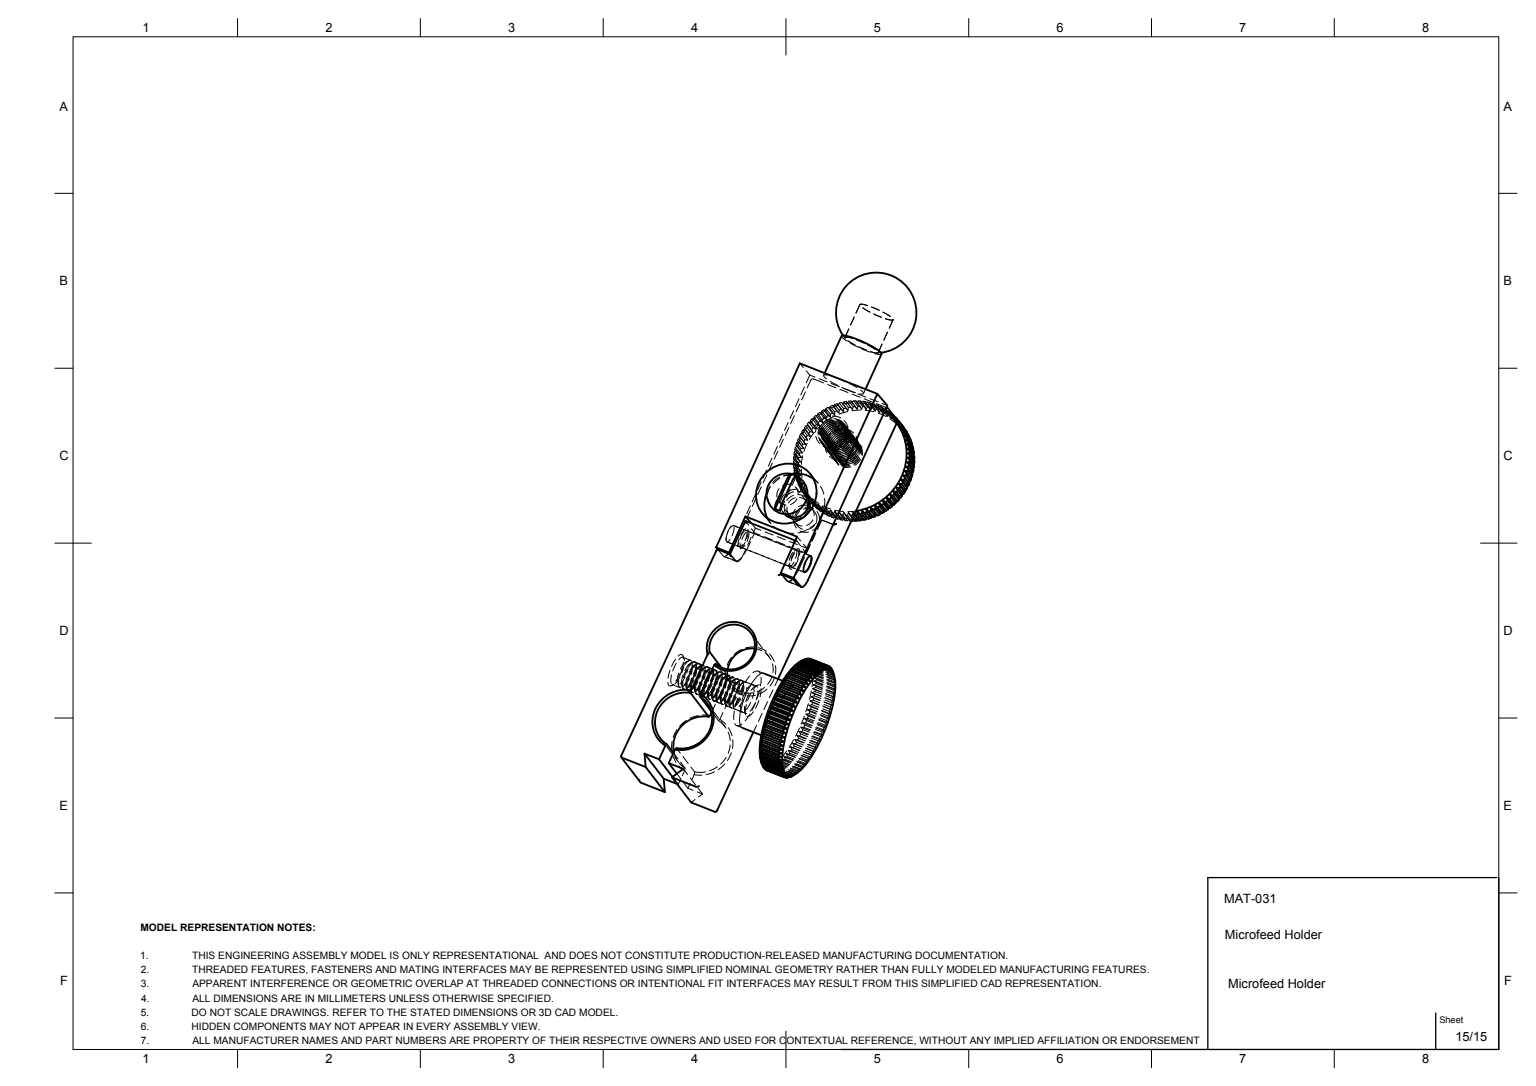
ISO-10303-21;
HEADER;
/* Generated by software containing ST-Developer
 * from STEP Tools, Inc. (www.steptools.com) 
 */

FILE_DESCRIPTION(
/* description */ ('STEP AP214'),
/* implementation_level */ '2;1');

FILE_NAME(
/* name */ 'Microfeed Holder.step',
/* time_stamp */ '2026-11-14T06:58:01-08:00',
/* author */ (''),
/* organization */ (''),
/* preprocessor_version */ 'ST-DEVELOPER v20.2',
/* originating_system */ 'Autodesk Translation Framework v15.17.0.0',
/* authorisation */ '');

FILE_SCHEMA (('AUTOMOTIVE_DESIGN { 1 0 10303 214 3 1 1 }'));
ENDSEC;

DATA;
#10=MECHANICAL_DESIGN_GEOMETRIC_PRESENTATION_REPRESENTATION('',(#1159,#1160,#1161,#1162,#1163,#1164,#1165),#38635);
#68=ELLIPSE('',#18534,0.424264068711536,0.299999999999714);
#69=ELLIPSE('',#18536,0.424264068712725,0.300000000000503);
#70=ELLIPSE('',#18544,0.424264068711314,0.299999999999553);
#71=ELLIPSE('',#18551,0.424264068712409,0.300000000000364);
#72=ELLIPSE('',#18570,0.424264068711872,0.299999999999922);
#73=ELLIPSE('',#18576,0.42426406871188,0.299999999999951);
#74=ELLIPSE('',#18583,0.424264068709732,0.299999999998459);
#75=ELLIPSE('',#18585,0.424264068710271,0.299999999998872);
#76=ELLIPSE('',#18587,0.424264068711053,0.29999999999941);
#77=ELLIPSE('',#18589,0.424264068710426,0.299999999998988);
#117=SPHERICAL_SURFACE('',#18547,0.3);
#118=SPHERICAL_SURFACE('',#18565,0.3);
#119=SPHERICAL_SURFACE('',#18567,0.3);
#120=SPHERICAL_SURFACE('',#18577,0.3);
#121=SPHERICAL_SURFACE('',#18580,0.3);
#122=SPHERICAL_SURFACE('',#18592,0.3);
#123=SPHERICAL_SURFACE('',#18653,5.5);
#179=TOROIDAL_SURFACE('',#18545,3.3,0.3);
#180=TOROIDAL_SURFACE('',#18563,3.3,0.3);
#181=TOROIDAL_SURFACE('',#18597,1.1,0.1);
#182=TOROIDAL_SURFACE('',#18602,1.1,0.1);
#183=TOROIDAL_SURFACE('',#18656,2.5,0.5);
#184=TOROIDAL_SURFACE('',#19189,1.81782234903766,0.9);
#185=TOROIDAL_SURFACE('',#19210,4.5,0.5);
#238=(
BOUNDED_CURVE()
B_SPLINE_CURVE(2,(#33393,#33394,#33395),.UNSPECIFIED.,.F.,.F.)
B_SPLINE_CURVE_WITH_KNOTS((3,3),(0.0421543904155743,0.059561882542862),
 .UNSPECIFIED.)
CURVE()
GEOMETRIC_REPRESENTATION_ITEM()
RATIONAL_B_SPLINE_CURVE((1.21505376344088,1.25768410333319,1.29885057471263))
REPRESENTATION_ITEM('')
);
#239=(
BOUNDED_CURVE()
B_SPLINE_CURVE(2,(#33398,#33399,#33400),.UNSPECIFIED.,.F.,.F.)
B_SPLINE_CURVE_WITH_KNOTS((3,3),(-0.162076637737085,-0.10981765032222),
 .UNSPECIFIED.)
CURVE()
GEOMETRIC_REPRESENTATION_ITEM()
RATIONAL_B_SPLINE_CURVE((1.22222222222222,1.19527460940787,1.16260162601569))
REPRESENTATION_ITEM('')
);
#240=(
BOUNDED_CURVE()
B_SPLINE_CURVE(2,(#33434,#33435,#33436),.UNSPECIFIED.,.F.,.F.)
B_SPLINE_CURVE_WITH_KNOTS((3,3),(0.109817650322217,0.162076637737086),
 .UNSPECIFIED.)
CURVE()
GEOMETRIC_REPRESENTATION_ITEM()
RATIONAL_B_SPLINE_CURVE((1.16260162601569,1.19527460940787,1.22222222222222))
REPRESENTATION_ITEM('')
);
#241=(
BOUNDED_CURVE()
B_SPLINE_CURVE(2,(#33439,#33440,#33441),.UNSPECIFIED.,.F.,.F.)
B_SPLINE_CURVE_WITH_KNOTS((3,3),(-0.0595618825429998,-0.0421543904157002),
 .UNSPECIFIED.)
CURVE()
GEOMETRIC_REPRESENTATION_ITEM()
RATIONAL_B_SPLINE_CURVE((1.29885057471333,1.25768410333386,1.21505376344153))
REPRESENTATION_ITEM('')
);
#242=(
BOUNDED_CURVE()
B_SPLINE_CURVE(2,(#34217,#34218,#34219),.UNSPECIFIED.,.F.,.F.)
B_SPLINE_CURVE_WITH_KNOTS((3,3),(0.536094506482407,0.589144372850599),
 .UNSPECIFIED.)
CURVE()
GEOMETRIC_REPRESENTATION_ITEM()
RATIONAL_B_SPLINE_CURVE((1.0242816296211,1.02311336089471,1.02147610370002))
REPRESENTATION_ITEM('')
);
#243=(
BOUNDED_CURVE()
B_SPLINE_CURVE(2,(#34223,#34224,#34225),.UNSPECIFIED.,.F.,.F.)
B_SPLINE_CURVE_WITH_KNOTS((3,3),(0.218746031477168,0.271795897845357),
 .UNSPECIFIED.)
CURVE()
GEOMETRIC_REPRESENTATION_ITEM()
RATIONAL_B_SPLINE_CURVE((1.02147610369998,1.02311336089466,1.02428162962105))
REPRESENTATION_ITEM('')
);
#244=(
BOUNDED_CURVE()
B_SPLINE_CURVE(2,(#34227,#34228,#34229),.UNSPECIFIED.,.F.,.F.)
B_SPLINE_CURVE_WITH_KNOTS((3,3),(0.536094506482406,0.589144372850588),
 .UNSPECIFIED.)
CURVE()
GEOMETRIC_REPRESENTATION_ITEM()
RATIONAL_B_SPLINE_CURVE((1.02428162962092,1.02311336089453,1.02147610369986))
REPRESENTATION_ITEM('')
);
#245=(
BOUNDED_CURVE()
B_SPLINE_CURVE(2,(#34233,#34234,#34235),.UNSPECIFIED.,.F.,.F.)
B_SPLINE_CURVE_WITH_KNOTS((3,3),(0.21874603147717,0.271795897845354),
 .UNSPECIFIED.)
CURVE()
GEOMETRIC_REPRESENTATION_ITEM()
RATIONAL_B_SPLINE_CURVE((1.02147610369991,1.02311336089458,1.02428162962097))
REPRESENTATION_ITEM('')
);
#246=(
BOUNDED_CURVE()
B_SPLINE_CURVE(2,(#34237,#34238,#34239),.UNSPECIFIED.,.F.,.F.)
B_SPLINE_CURVE_WITH_KNOTS((3,3),(0.536094506482412,0.589144372850605),
 .UNSPECIFIED.)
CURVE()
GEOMETRIC_REPRESENTATION_ITEM()
RATIONAL_B_SPLINE_CURVE((1.02428162962116,1.02311336089476,1.02147610370007))
REPRESENTATION_ITEM('')
);
#247=(
BOUNDED_CURVE()
B_SPLINE_CURVE(2,(#34243,#34244,#34245),.UNSPECIFIED.,.F.,.F.)
B_SPLINE_CURVE_WITH_KNOTS((3,3),(0.218746031477164,0.27179589784535),
 .UNSPECIFIED.)
CURVE()
GEOMETRIC_REPRESENTATION_ITEM()
RATIONAL_B_SPLINE_CURVE((1.02147610369995,1.02311336089462,1.02428162962101))
REPRESENTATION_ITEM('')
);
#248=(
BOUNDED_CURVE()
B_SPLINE_CURVE(2,(#34247,#34248,#34249),.UNSPECIFIED.,.F.,.F.)
B_SPLINE_CURVE_WITH_KNOTS((3,3),(0.536094506482389,0.589144372850566),
 .UNSPECIFIED.)
CURVE()
GEOMETRIC_REPRESENTATION_ITEM()
RATIONAL_B_SPLINE_CURVE((1.0242816296208,1.02311336089442,1.02147610369976))
REPRESENTATION_ITEM('')
);
#249=(
BOUNDED_CURVE()
B_SPLINE_CURVE(2,(#34253,#34254,#34255),.UNSPECIFIED.,.F.,.F.)
B_SPLINE_CURVE_WITH_KNOTS((3,3),(0.218746031477182,0.271795897845361),
 .UNSPECIFIED.)
CURVE()
GEOMETRIC_REPRESENTATION_ITEM()
RATIONAL_B_SPLINE_CURVE((1.02147610369979,1.02311336089445,1.02428162962083))
REPRESENTATION_ITEM('')
);
#250=(
BOUNDED_CURVE()
B_SPLINE_CURVE(2,(#34257,#34258,#34259),.UNSPECIFIED.,.F.,.F.)
B_SPLINE_CURVE_WITH_KNOTS((3,3),(0.536094506482412,0.589144372850601),
 .UNSPECIFIED.)
CURVE()
GEOMETRIC_REPRESENTATION_ITEM()
RATIONAL_B_SPLINE_CURVE((1.02428162962106,1.02311336089466,1.02147610369999))
REPRESENTATION_ITEM('')
);
#251=(
BOUNDED_CURVE()
B_SPLINE_CURVE(2,(#34263,#34264,#34265),.UNSPECIFIED.,.F.,.F.)
B_SPLINE_CURVE_WITH_KNOTS((3,3),(0.218746031477185,0.271795897845363),
 .UNSPECIFIED.)
CURVE()
GEOMETRIC_REPRESENTATION_ITEM()
RATIONAL_B_SPLINE_CURVE((1.02147610369979,1.02311336089445,1.02428162962084))
REPRESENTATION_ITEM('')
);
#252=(
BOUNDED_CURVE()
B_SPLINE_CURVE(2,(#34267,#34268,#34269),.UNSPECIFIED.,.F.,.F.)
B_SPLINE_CURVE_WITH_KNOTS((3,3),(0.536094506482394,0.589144372850572),
 .UNSPECIFIED.)
CURVE()
GEOMETRIC_REPRESENTATION_ITEM()
RATIONAL_B_SPLINE_CURVE((1.02428162962082,1.02311336089444,1.02147610369978))
REPRESENTATION_ITEM('')
);
#253=(
BOUNDED_CURVE()
B_SPLINE_CURVE(2,(#34273,#34274,#34275),.UNSPECIFIED.,.F.,.F.)
B_SPLINE_CURVE_WITH_KNOTS((3,3),(0.21874603147717,0.271795897845349),
 .UNSPECIFIED.)
CURVE()
GEOMETRIC_REPRESENTATION_ITEM()
RATIONAL_B_SPLINE_CURVE((1.02147610369983,1.0231133608945,1.02428162962088))
REPRESENTATION_ITEM('')
);
#254=(
BOUNDED_CURVE()
B_SPLINE_CURVE(2,(#34277,#34278,#34279),.UNSPECIFIED.,.F.,.F.)
B_SPLINE_CURVE_WITH_KNOTS((3,3),(0.536094506482412,0.589144372850599),
 .UNSPECIFIED.)
CURVE()
GEOMETRIC_REPRESENTATION_ITEM()
RATIONAL_B_SPLINE_CURVE((1.02428162962104,1.02311336089465,1.02147610369997))
REPRESENTATION_ITEM('')
);
#255=(
BOUNDED_CURVE()
B_SPLINE_CURVE(2,(#34283,#34284,#34285),.UNSPECIFIED.,.F.,.F.)
B_SPLINE_CURVE_WITH_KNOTS((3,3),(0.218746031477174,0.271795897845355),
 .UNSPECIFIED.)
CURVE()
GEOMETRIC_REPRESENTATION_ITEM()
RATIONAL_B_SPLINE_CURVE((1.02147610369982,1.02311336089449,1.02428162962087))
REPRESENTATION_ITEM('')
);
#256=(
BOUNDED_CURVE()
B_SPLINE_CURVE(2,(#34287,#34288,#34289),.UNSPECIFIED.,.F.,.F.)
B_SPLINE_CURVE_WITH_KNOTS((3,3),(0.536094506482407,0.589144372850592),
 .UNSPECIFIED.)
CURVE()
GEOMETRIC_REPRESENTATION_ITEM()
RATIONAL_B_SPLINE_CURVE((1.02428162962099,1.0231133608946,1.02147610369992))
REPRESENTATION_ITEM('')
);
#257=(
BOUNDED_CURVE()
B_SPLINE_CURVE(2,(#34293,#34294,#34295),.UNSPECIFIED.,.F.,.F.)
B_SPLINE_CURVE_WITH_KNOTS((3,3),(0.218746031477156,0.271795897845345),
 .UNSPECIFIED.)
CURVE()
GEOMETRIC_REPRESENTATION_ITEM()
RATIONAL_B_SPLINE_CURVE((1.02147610369998,1.02311336089466,1.02428162962106))
REPRESENTATION_ITEM('')
);
#258=(
BOUNDED_CURVE()
B_SPLINE_CURVE(2,(#34297,#34298,#34299),.UNSPECIFIED.,.F.,.F.)
B_SPLINE_CURVE_WITH_KNOTS((3,3),(0.53609450648241,0.5891443728506),
 .UNSPECIFIED.)
CURVE()
GEOMETRIC_REPRESENTATION_ITEM()
RATIONAL_B_SPLINE_CURVE((1.02428162962108,1.02311336089468,1.0214761037))
REPRESENTATION_ITEM('')
);
#259=(
BOUNDED_CURVE()
B_SPLINE_CURVE(2,(#34303,#34304,#34305),.UNSPECIFIED.,.F.,.F.)
B_SPLINE_CURVE_WITH_KNOTS((3,3),(0.21874603147718,0.271795897845362),
 .UNSPECIFIED.)
CURVE()
GEOMETRIC_REPRESENTATION_ITEM()
RATIONAL_B_SPLINE_CURVE((1.02147610369984,1.02311336089451,1.02428162962089))
REPRESENTATION_ITEM('')
);
#260=(
BOUNDED_CURVE()
B_SPLINE_CURVE(2,(#34307,#34308,#34309),.UNSPECIFIED.,.F.,.F.)
B_SPLINE_CURVE_WITH_KNOTS((3,3),(0.536094506482414,0.589144372850597),
 .UNSPECIFIED.)
CURVE()
GEOMETRIC_REPRESENTATION_ITEM()
RATIONAL_B_SPLINE_CURVE((1.02428162962095,1.02311336089456,1.02147610369989))
REPRESENTATION_ITEM('')
);
#261=(
BOUNDED_CURVE()
B_SPLINE_CURVE(2,(#34313,#34314,#34315),.UNSPECIFIED.,.F.,.F.)
B_SPLINE_CURVE_WITH_KNOTS((3,3),(0.218746031477174,0.27179589784536),
 .UNSPECIFIED.)
CURVE()
GEOMETRIC_REPRESENTATION_ITEM()
RATIONAL_B_SPLINE_CURVE((1.02147610369991,1.02311336089459,1.02428162962097))
REPRESENTATION_ITEM('')
);
#262=(
BOUNDED_CURVE()
B_SPLINE_CURVE(2,(#34317,#34318,#34319),.UNSPECIFIED.,.F.,.F.)
B_SPLINE_CURVE_WITH_KNOTS((3,3),(0.536094506482426,0.589144372850614),
 .UNSPECIFIED.)
CURVE()
GEOMETRIC_REPRESENTATION_ITEM()
RATIONAL_B_SPLINE_CURVE((1.02428162962107,1.02311336089468,1.0214761037))
REPRESENTATION_ITEM('')
);
#263=(
BOUNDED_CURVE()
B_SPLINE_CURVE(2,(#34323,#34324,#34325),.UNSPECIFIED.,.F.,.F.)
B_SPLINE_CURVE_WITH_KNOTS((3,3),(0.218746031477169,0.271795897845354),
 .UNSPECIFIED.)
CURVE()
GEOMETRIC_REPRESENTATION_ITEM()
RATIONAL_B_SPLINE_CURVE((1.02147610369993,1.0231133608946,1.02428162962099))
REPRESENTATION_ITEM('')
);
#264=(
BOUNDED_CURVE()
B_SPLINE_CURVE(2,(#34327,#34328,#34329),.UNSPECIFIED.,.F.,.F.)
B_SPLINE_CURVE_WITH_KNOTS((3,3),(0.536094506482401,0.589144372850587),
 .UNSPECIFIED.)
CURVE()
GEOMETRIC_REPRESENTATION_ITEM()
RATIONAL_B_SPLINE_CURVE((1.02428162962099,1.0231133608946,1.02147610369993))
REPRESENTATION_ITEM('')
);
#265=(
BOUNDED_CURVE()
B_SPLINE_CURVE(2,(#34333,#34334,#34335),.UNSPECIFIED.,.F.,.F.)
B_SPLINE_CURVE_WITH_KNOTS((3,3),(0.218746031477173,0.271795897845356),
 .UNSPECIFIED.)
CURVE()
GEOMETRIC_REPRESENTATION_ITEM()
RATIONAL_B_SPLINE_CURVE((1.02147610369988,1.02311336089455,1.02428162962094))
REPRESENTATION_ITEM('')
);
#266=(
BOUNDED_CURVE()
B_SPLINE_CURVE(2,(#34337,#34338,#34339),.UNSPECIFIED.,.F.,.F.)
B_SPLINE_CURVE_WITH_KNOTS((3,3),(0.536094506482398,0.589144372850579),
 .UNSPECIFIED.)
CURVE()
GEOMETRIC_REPRESENTATION_ITEM()
RATIONAL_B_SPLINE_CURVE((1.0242816296209,1.02311336089451,1.02147610369984))
REPRESENTATION_ITEM('')
);
#267=(
BOUNDED_CURVE()
B_SPLINE_CURVE(2,(#34343,#34344,#34345),.UNSPECIFIED.,.F.,.F.)
B_SPLINE_CURVE_WITH_KNOTS((3,3),(0.218746031477172,0.271795897845351),
 .UNSPECIFIED.)
CURVE()
GEOMETRIC_REPRESENTATION_ITEM()
RATIONAL_B_SPLINE_CURVE((1.02147610369978,1.02311336089444,1.02428162962083))
REPRESENTATION_ITEM('')
);
#268=(
BOUNDED_CURVE()
B_SPLINE_CURVE(2,(#34347,#34348,#34349),.UNSPECIFIED.,.F.,.F.)
B_SPLINE_CURVE_WITH_KNOTS((3,3),(0.536094506482419,0.589144372850608),
 .UNSPECIFIED.)
CURVE()
GEOMETRIC_REPRESENTATION_ITEM()
RATIONAL_B_SPLINE_CURVE((1.02428162962106,1.02311336089467,1.02147610369999))
REPRESENTATION_ITEM('')
);
#269=(
BOUNDED_CURVE()
B_SPLINE_CURVE(2,(#34353,#34354,#34355),.UNSPECIFIED.,.F.,.F.)
B_SPLINE_CURVE_WITH_KNOTS((3,3),(0.218746031477166,0.271795897845348),
 .UNSPECIFIED.)
CURVE()
GEOMETRIC_REPRESENTATION_ITEM()
RATIONAL_B_SPLINE_CURVE((1.02147610369987,1.02311336089454,1.02428162962093))
REPRESENTATION_ITEM('')
);
#270=(
BOUNDED_CURVE()
B_SPLINE_CURVE(2,(#34357,#34358,#34359),.UNSPECIFIED.,.F.,.F.)
B_SPLINE_CURVE_WITH_KNOTS((3,3),(0.536094506482413,0.589144372850599),
 .UNSPECIFIED.)
CURVE()
GEOMETRIC_REPRESENTATION_ITEM()
RATIONAL_B_SPLINE_CURVE((1.02428162962102,1.02311336089463,1.02147610369995))
REPRESENTATION_ITEM('')
);
#271=(
BOUNDED_CURVE()
B_SPLINE_CURVE(2,(#34363,#34364,#34365),.UNSPECIFIED.,.F.,.F.)
B_SPLINE_CURVE_WITH_KNOTS((3,3),(0.218746031477176,0.271795897845356),
 .UNSPECIFIED.)
CURVE()
GEOMETRIC_REPRESENTATION_ITEM()
RATIONAL_B_SPLINE_CURVE((1.02147610369983,1.0231133608945,1.02428162962088))
REPRESENTATION_ITEM('')
);
#272=(
BOUNDED_CURVE()
B_SPLINE_CURVE(2,(#34367,#34368,#34369),.UNSPECIFIED.,.F.,.F.)
B_SPLINE_CURVE_WITH_KNOTS((3,3),(0.536094506482413,0.589144372850592),
 .UNSPECIFIED.)
CURVE()
GEOMETRIC_REPRESENTATION_ITEM()
RATIONAL_B_SPLINE_CURVE((1.02428162962088,1.02311336089449,1.02147610369982))
REPRESENTATION_ITEM('')
);
#273=(
BOUNDED_CURVE()
B_SPLINE_CURVE(2,(#34373,#34374,#34375),.UNSPECIFIED.,.F.,.F.)
B_SPLINE_CURVE_WITH_KNOTS((3,3),(0.218746031477187,0.27179589784537),
 .UNSPECIFIED.)
CURVE()
GEOMETRIC_REPRESENTATION_ITEM()
RATIONAL_B_SPLINE_CURVE((1.02147610369983,1.0231133608945,1.02428162962088))
REPRESENTATION_ITEM('')
);
#274=(
BOUNDED_CURVE()
B_SPLINE_CURVE(2,(#34377,#34378,#34379),.UNSPECIFIED.,.F.,.F.)
B_SPLINE_CURVE_WITH_KNOTS((3,3),(0.53609450648241,0.589144372850596),
 .UNSPECIFIED.)
CURVE()
GEOMETRIC_REPRESENTATION_ITEM()
RATIONAL_B_SPLINE_CURVE((1.02428162962098,1.02311336089459,1.02147610369992))
REPRESENTATION_ITEM('')
);
#275=(
BOUNDED_CURVE()
B_SPLINE_CURVE(2,(#34383,#34384,#34385),.UNSPECIFIED.,.F.,.F.)
B_SPLINE_CURVE_WITH_KNOTS((3,3),(0.218746031477173,0.271795897845356),
 .UNSPECIFIED.)
CURVE()
GEOMETRIC_REPRESENTATION_ITEM()
RATIONAL_B_SPLINE_CURVE((1.02147610369988,1.02311336089455,1.02428162962094))
REPRESENTATION_ITEM('')
);
#276=(
BOUNDED_CURVE()
B_SPLINE_CURVE(2,(#34387,#34388,#34389),.UNSPECIFIED.,.F.,.F.)
B_SPLINE_CURVE_WITH_KNOTS((3,3),(0.536094506482401,0.589144372850587),
 .UNSPECIFIED.)
CURVE()
GEOMETRIC_REPRESENTATION_ITEM()
RATIONAL_B_SPLINE_CURVE((1.024281629621,1.02311336089461,1.02147610369994))
REPRESENTATION_ITEM('')
);
#277=(
BOUNDED_CURVE()
B_SPLINE_CURVE(2,(#34393,#34394,#34395),.UNSPECIFIED.,.F.,.F.)
B_SPLINE_CURVE_WITH_KNOTS((3,3),(0.218746031477176,0.271795897845359),
 .UNSPECIFIED.)
CURVE()
GEOMETRIC_REPRESENTATION_ITEM()
RATIONAL_B_SPLINE_CURVE((1.02147610369987,1.02311336089454,1.02428162962092))
REPRESENTATION_ITEM('')
);
#278=(
BOUNDED_CURVE()
B_SPLINE_CURVE(2,(#34397,#34398,#34399),.UNSPECIFIED.,.F.,.F.)
B_SPLINE_CURVE_WITH_KNOTS((3,3),(0.536094506482401,0.589144372850584),
 .UNSPECIFIED.)
CURVE()
GEOMETRIC_REPRESENTATION_ITEM()
RATIONAL_B_SPLINE_CURVE((1.02428162962093,1.02311336089454,1.02147610369987))
REPRESENTATION_ITEM('')
);
#279=(
BOUNDED_CURVE()
B_SPLINE_CURVE(2,(#34403,#34404,#34405),.UNSPECIFIED.,.F.,.F.)
B_SPLINE_CURVE_WITH_KNOTS((3,3),(0.218746031477161,0.271795897845347),
 .UNSPECIFIED.)
CURVE()
GEOMETRIC_REPRESENTATION_ITEM()
RATIONAL_B_SPLINE_CURVE((1.02147610369995,1.02311336089462,1.02428162962101))
REPRESENTATION_ITEM('')
);
#280=(
BOUNDED_CURVE()
B_SPLINE_CURVE(2,(#34407,#34408,#34409),.UNSPECIFIED.,.F.,.F.)
B_SPLINE_CURVE_WITH_KNOTS((3,3),(0.536094506482406,0.589144372850593),
 .UNSPECIFIED.)
CURVE()
GEOMETRIC_REPRESENTATION_ITEM()
RATIONAL_B_SPLINE_CURVE((1.02428162962101,1.02311336089462,1.02147610369994))
REPRESENTATION_ITEM('')
);
#281=(
BOUNDED_CURVE()
B_SPLINE_CURVE(2,(#34413,#34414,#34415),.UNSPECIFIED.,.F.,.F.)
B_SPLINE_CURVE_WITH_KNOTS((3,3),(0.218746031477175,0.271795897845356),
 .UNSPECIFIED.)
CURVE()
GEOMETRIC_REPRESENTATION_ITEM()
RATIONAL_B_SPLINE_CURVE((1.02147610369983,1.0231133608945,1.02428162962088))
REPRESENTATION_ITEM('')
);
#282=(
BOUNDED_CURVE()
B_SPLINE_CURVE(2,(#34417,#34418,#34419),.UNSPECIFIED.,.F.,.F.)
B_SPLINE_CURVE_WITH_KNOTS((3,3),(0.536094506482409,0.589144372850594),
 .UNSPECIFIED.)
CURVE()
GEOMETRIC_REPRESENTATION_ITEM()
RATIONAL_B_SPLINE_CURVE((1.02428162962098,1.02311336089459,1.02147610369992))
REPRESENTATION_ITEM('')
);
#283=(
BOUNDED_CURVE()
B_SPLINE_CURVE(2,(#34423,#34424,#34425),.UNSPECIFIED.,.F.,.F.)
B_SPLINE_CURVE_WITH_KNOTS((3,3),(0.218746031477174,0.271795897845362),
 .UNSPECIFIED.)
CURVE()
GEOMETRIC_REPRESENTATION_ITEM()
RATIONAL_B_SPLINE_CURVE((1.02147610369994,1.02311336089462,1.02428162962101))
REPRESENTATION_ITEM('')
);
#284=(
BOUNDED_CURVE()
B_SPLINE_CURVE(2,(#34427,#34428,#34429),.UNSPECIFIED.,.F.,.F.)
B_SPLINE_CURVE_WITH_KNOTS((3,3),(0.536094506482415,0.589144372850602),
 .UNSPECIFIED.)
CURVE()
GEOMETRIC_REPRESENTATION_ITEM()
RATIONAL_B_SPLINE_CURVE((1.02428162962101,1.02311336089462,1.02147610369994))
REPRESENTATION_ITEM('')
);
#285=(
BOUNDED_CURVE()
B_SPLINE_CURVE(2,(#34433,#34434,#34435),.UNSPECIFIED.,.F.,.F.)
B_SPLINE_CURVE_WITH_KNOTS((3,3),(0.218746031477172,0.271795897845355),
 .UNSPECIFIED.)
CURVE()
GEOMETRIC_REPRESENTATION_ITEM()
RATIONAL_B_SPLINE_CURVE((1.02147610369986,1.02311336089453,1.02428162962092))
REPRESENTATION_ITEM('')
);
#286=(
BOUNDED_CURVE()
B_SPLINE_CURVE(2,(#34437,#34438,#34439),.UNSPECIFIED.,.F.,.F.)
B_SPLINE_CURVE_WITH_KNOTS((3,3),(0.536094506482405,0.589144372850589),
 .UNSPECIFIED.)
CURVE()
GEOMETRIC_REPRESENTATION_ITEM()
RATIONAL_B_SPLINE_CURVE((1.02428162962097,1.02311336089458,1.02147610369991))
REPRESENTATION_ITEM('')
);
#287=(
BOUNDED_CURVE()
B_SPLINE_CURVE(2,(#34443,#34444,#34445),.UNSPECIFIED.,.F.,.F.)
B_SPLINE_CURVE_WITH_KNOTS((3,3),(0.218746031477162,0.271795897845346),
 .UNSPECIFIED.)
CURVE()
GEOMETRIC_REPRESENTATION_ITEM()
RATIONAL_B_SPLINE_CURVE((1.02147610369991,1.02311336089459,1.02428162962098))
REPRESENTATION_ITEM('')
);
#288=(
BOUNDED_CURVE()
B_SPLINE_CURVE(2,(#34447,#34448,#34449),.UNSPECIFIED.,.F.,.F.)
B_SPLINE_CURVE_WITH_KNOTS((3,3),(0.536094506482411,0.589144372850603),
 .UNSPECIFIED.)
CURVE()
GEOMETRIC_REPRESENTATION_ITEM()
RATIONAL_B_SPLINE_CURVE((1.02428162962113,1.02311336089474,1.02147610370005))
REPRESENTATION_ITEM('')
);
#289=(
BOUNDED_CURVE()
B_SPLINE_CURVE(2,(#34453,#34454,#34455),.UNSPECIFIED.,.F.,.F.)
B_SPLINE_CURVE_WITH_KNOTS((3,3),(0.218746031477171,0.271795897845351),
 .UNSPECIFIED.)
CURVE()
GEOMETRIC_REPRESENTATION_ITEM()
RATIONAL_B_SPLINE_CURVE((1.02147610369981,1.02311336089448,1.02428162962086))
REPRESENTATION_ITEM('')
);
#290=(
BOUNDED_CURVE()
B_SPLINE_CURVE(2,(#34457,#34458,#34459),.UNSPECIFIED.,.F.,.F.)
B_SPLINE_CURVE_WITH_KNOTS((3,3),(0.536094506482409,0.589144372850599),
 .UNSPECIFIED.)
CURVE()
GEOMETRIC_REPRESENTATION_ITEM()
RATIONAL_B_SPLINE_CURVE((1.02428162962106,1.02311336089467,1.02147610369999))
REPRESENTATION_ITEM('')
);
#291=(
BOUNDED_CURVE()
B_SPLINE_CURVE(2,(#34463,#34464,#34465),.UNSPECIFIED.,.F.,.F.)
B_SPLINE_CURVE_WITH_KNOTS((3,3),(0.218746031477179,0.271795897845364),
 .UNSPECIFIED.)
CURVE()
GEOMETRIC_REPRESENTATION_ITEM()
RATIONAL_B_SPLINE_CURVE((1.02147610369988,1.02311336089455,1.02428162962094))
REPRESENTATION_ITEM('')
);
#292=(
BOUNDED_CURVE()
B_SPLINE_CURVE(2,(#34467,#34468,#34469),.UNSPECIFIED.,.F.,.F.)
B_SPLINE_CURVE_WITH_KNOTS((3,3),(0.536094506482416,0.589144372850601),
 .UNSPECIFIED.)
CURVE()
GEOMETRIC_REPRESENTATION_ITEM()
RATIONAL_B_SPLINE_CURVE((1.024281629621,1.02311336089461,1.02147610369993))
REPRESENTATION_ITEM('')
);
#293=(
BOUNDED_CURVE()
B_SPLINE_CURVE(2,(#34473,#34474,#34475),.UNSPECIFIED.,.F.,.F.)
B_SPLINE_CURVE_WITH_KNOTS((3,3),(0.218746031477175,0.27179589784536),
 .UNSPECIFIED.)
CURVE()
GEOMETRIC_REPRESENTATION_ITEM()
RATIONAL_B_SPLINE_CURVE((1.02147610369991,1.02311336089459,1.02428162962098))
REPRESENTATION_ITEM('')
);
#294=(
BOUNDED_CURVE()
B_SPLINE_CURVE(2,(#34477,#34478,#34479),.UNSPECIFIED.,.F.,.F.)
B_SPLINE_CURVE_WITH_KNOTS((3,3),(0.5360945064824,0.58914437285059),
 .UNSPECIFIED.)
CURVE()
GEOMETRIC_REPRESENTATION_ITEM()
RATIONAL_B_SPLINE_CURVE((1.02428162962107,1.02311336089468,1.0214761037))
REPRESENTATION_ITEM('')
);
#295=(
BOUNDED_CURVE()
B_SPLINE_CURVE(2,(#34483,#34484,#34485),.UNSPECIFIED.,.F.,.F.)
B_SPLINE_CURVE_WITH_KNOTS((3,3),(0.218746031477166,0.271795897845347),
 .UNSPECIFIED.)
CURVE()
GEOMETRIC_REPRESENTATION_ITEM()
RATIONAL_B_SPLINE_CURVE((1.02147610369984,1.0231133608945,1.02428162962089))
REPRESENTATION_ITEM('')
);
#296=(
BOUNDED_CURVE()
B_SPLINE_CURVE(2,(#34487,#34488,#34489),.UNSPECIFIED.,.F.,.F.)
B_SPLINE_CURVE_WITH_KNOTS((3,3),(0.536094506482403,0.589144372850591),
 .UNSPECIFIED.)
CURVE()
GEOMETRIC_REPRESENTATION_ITEM()
RATIONAL_B_SPLINE_CURVE((1.02428162962102,1.02311336089463,1.02147610369995))
REPRESENTATION_ITEM('')
);
#297=(
BOUNDED_CURVE()
B_SPLINE_CURVE(2,(#34493,#34494,#34495),.UNSPECIFIED.,.F.,.F.)
B_SPLINE_CURVE_WITH_KNOTS((3,3),(0.218746031477165,0.271795897845349),
 .UNSPECIFIED.)
CURVE()
GEOMETRIC_REPRESENTATION_ITEM()
RATIONAL_B_SPLINE_CURVE((1.02147610369991,1.02311336089458,1.02428162962097))
REPRESENTATION_ITEM('')
);
#298=(
BOUNDED_CURVE()
B_SPLINE_CURVE(2,(#34497,#34498,#34499),.UNSPECIFIED.,.F.,.F.)
B_SPLINE_CURVE_WITH_KNOTS((3,3),(0.536094506482402,0.589144372850584),
 .UNSPECIFIED.)
CURVE()
GEOMETRIC_REPRESENTATION_ITEM()
RATIONAL_B_SPLINE_CURVE((1.02428162962092,1.02311336089454,1.02147610369987))
REPRESENTATION_ITEM('')
);
#299=(
BOUNDED_CURVE()
B_SPLINE_CURVE(2,(#34503,#34504,#34505),.UNSPECIFIED.,.F.,.F.)
B_SPLINE_CURVE_WITH_KNOTS((3,3),(0.218746031477178,0.271795897845364),
 .UNSPECIFIED.)
CURVE()
GEOMETRIC_REPRESENTATION_ITEM()
RATIONAL_B_SPLINE_CURVE((1.02147610369991,1.02311336089458,1.02428162962097))
REPRESENTATION_ITEM('')
);
#300=(
BOUNDED_CURVE()
B_SPLINE_CURVE(2,(#34507,#34508,#34509),.UNSPECIFIED.,.F.,.F.)
B_SPLINE_CURVE_WITH_KNOTS((3,3),(0.536094506482408,0.589144372850591),
 .UNSPECIFIED.)
CURVE()
GEOMETRIC_REPRESENTATION_ITEM()
RATIONAL_B_SPLINE_CURVE((1.02428162962092,1.02311336089453,1.02147610369986))
REPRESENTATION_ITEM('')
);
#301=(
BOUNDED_CURVE()
B_SPLINE_CURVE(2,(#34513,#34514,#34515),.UNSPECIFIED.,.F.,.F.)
B_SPLINE_CURVE_WITH_KNOTS((3,3),(0.218746031477175,0.27179589784536),
 .UNSPECIFIED.)
CURVE()
GEOMETRIC_REPRESENTATION_ITEM()
RATIONAL_B_SPLINE_CURVE((1.02147610369989,1.02311336089456,1.02428162962095))
REPRESENTATION_ITEM('')
);
#302=(
BOUNDED_CURVE()
B_SPLINE_CURVE(2,(#34517,#34518,#34519),.UNSPECIFIED.,.F.,.F.)
B_SPLINE_CURVE_WITH_KNOTS((3,3),(0.536094506482411,0.589144372850602),
 .UNSPECIFIED.)
CURVE()
GEOMETRIC_REPRESENTATION_ITEM()
RATIONAL_B_SPLINE_CURVE((1.0242816296211,1.02311336089471,1.02147610370002))
REPRESENTATION_ITEM('')
);
#303=(
BOUNDED_CURVE()
B_SPLINE_CURVE(2,(#34523,#34524,#34525),.UNSPECIFIED.,.F.,.F.)
B_SPLINE_CURVE_WITH_KNOTS((3,3),(0.218746031477173,0.271795897845357),
 .UNSPECIFIED.)
CURVE()
GEOMETRIC_REPRESENTATION_ITEM()
RATIONAL_B_SPLINE_CURVE((1.0214761036999,1.02311336089457,1.02428162962096))
REPRESENTATION_ITEM('')
);
#304=(
BOUNDED_CURVE()
B_SPLINE_CURVE(2,(#34527,#34528,#34529),.UNSPECIFIED.,.F.,.F.)
B_SPLINE_CURVE_WITH_KNOTS((3,3),(0.536094506482408,0.589144372850595),
 .UNSPECIFIED.)
CURVE()
GEOMETRIC_REPRESENTATION_ITEM()
RATIONAL_B_SPLINE_CURVE((1.02428162962105,1.02311336089466,1.02147610369998))
REPRESENTATION_ITEM('')
);
#305=(
BOUNDED_CURVE()
B_SPLINE_CURVE(2,(#34533,#34534,#34535),.UNSPECIFIED.,.F.,.F.)
B_SPLINE_CURVE_WITH_KNOTS((3,3),(0.218746031477171,0.271795897845354),
 .UNSPECIFIED.)
CURVE()
GEOMETRIC_REPRESENTATION_ITEM()
RATIONAL_B_SPLINE_CURVE((1.02147610369989,1.02311336089456,1.02428162962095))
REPRESENTATION_ITEM('')
);
#306=(
BOUNDED_CURVE()
B_SPLINE_CURVE(2,(#34537,#34538,#34539),.UNSPECIFIED.,.F.,.F.)
B_SPLINE_CURVE_WITH_KNOTS((3,3),(0.536094506482412,0.5891443728506),
 .UNSPECIFIED.)
CURVE()
GEOMETRIC_REPRESENTATION_ITEM()
RATIONAL_B_SPLINE_CURVE((1.02428162962106,1.02311336089467,1.02147610369999))
REPRESENTATION_ITEM('')
);
#307=(
BOUNDED_CURVE()
B_SPLINE_CURVE(2,(#34543,#34544,#34545),.UNSPECIFIED.,.F.,.F.)
B_SPLINE_CURVE_WITH_KNOTS((3,3),(0.218746031477183,0.27179589784537),
 .UNSPECIFIED.)
CURVE()
GEOMETRIC_REPRESENTATION_ITEM()
RATIONAL_B_SPLINE_CURVE((1.02147610369993,1.02311336089461,1.024281629621))
REPRESENTATION_ITEM('')
);
#308=(
BOUNDED_CURVE()
B_SPLINE_CURVE(2,(#34547,#34548,#34549),.UNSPECIFIED.,.F.,.F.)
B_SPLINE_CURVE_WITH_KNOTS((3,3),(0.536094506482412,0.589144372850597),
 .UNSPECIFIED.)
CURVE()
GEOMETRIC_REPRESENTATION_ITEM()
RATIONAL_B_SPLINE_CURVE((1.02428162962099,1.0231133608946,1.02147610369993))
REPRESENTATION_ITEM('')
);
#309=(
BOUNDED_CURVE()
B_SPLINE_CURVE(2,(#34553,#34554,#34555),.UNSPECIFIED.,.F.,.F.)
B_SPLINE_CURVE_WITH_KNOTS((3,3),(0.218746031477163,0.271795897845347),
 .UNSPECIFIED.)
CURVE()
GEOMETRIC_REPRESENTATION_ITEM()
RATIONAL_B_SPLINE_CURVE((1.02147610369992,1.0231133608946,1.02428162962099))
REPRESENTATION_ITEM('')
);
#310=(
BOUNDED_CURVE()
B_SPLINE_CURVE(2,(#34557,#34558,#34559),.UNSPECIFIED.,.F.,.F.)
B_SPLINE_CURVE_WITH_KNOTS((3,3),(0.536094506482402,0.589144372850587),
 .UNSPECIFIED.)
CURVE()
GEOMETRIC_REPRESENTATION_ITEM()
RATIONAL_B_SPLINE_CURVE((1.02428162962094,1.02311336089455,1.02147610369988))
REPRESENTATION_ITEM('')
);
#311=(
BOUNDED_CURVE()
B_SPLINE_CURVE(2,(#34563,#34564,#34565),.UNSPECIFIED.,.F.,.F.)
B_SPLINE_CURVE_WITH_KNOTS((3,3),(0.218746031477181,0.271795897845363),
 .UNSPECIFIED.)
CURVE()
GEOMETRIC_REPRESENTATION_ITEM()
RATIONAL_B_SPLINE_CURVE((1.02147610369986,1.02311336089453,1.02428162962091))
REPRESENTATION_ITEM('')
);
#312=(
BOUNDED_CURVE()
B_SPLINE_CURVE(2,(#34567,#34568,#34569),.UNSPECIFIED.,.F.,.F.)
B_SPLINE_CURVE_WITH_KNOTS((3,3),(0.536094506482409,0.58914437285059),
 .UNSPECIFIED.)
CURVE()
GEOMETRIC_REPRESENTATION_ITEM()
RATIONAL_B_SPLINE_CURVE((1.02428162962091,1.02311336089453,1.02147610369986))
REPRESENTATION_ITEM('')
);
#313=(
BOUNDED_CURVE()
B_SPLINE_CURVE(2,(#34573,#34574,#34575),.UNSPECIFIED.,.F.,.F.)
B_SPLINE_CURVE_WITH_KNOTS((3,3),(0.218746031477169,0.271795897845353),
 .UNSPECIFIED.)
CURVE()
GEOMETRIC_REPRESENTATION_ITEM()
RATIONAL_B_SPLINE_CURVE((1.0214761036999,1.02311336089457,1.02428162962096))
REPRESENTATION_ITEM('')
);
#314=(
BOUNDED_CURVE()
B_SPLINE_CURVE(2,(#34577,#34578,#34579),.UNSPECIFIED.,.F.,.F.)
B_SPLINE_CURVE_WITH_KNOTS((3,3),(0.536094506482403,0.58914437285059),
 .UNSPECIFIED.)
CURVE()
GEOMETRIC_REPRESENTATION_ITEM()
RATIONAL_B_SPLINE_CURVE((1.02428162962102,1.02311336089462,1.02147610369995))
REPRESENTATION_ITEM('')
);
#315=(
BOUNDED_CURVE()
B_SPLINE_CURVE(2,(#34583,#34584,#34585),.UNSPECIFIED.,.F.,.F.)
B_SPLINE_CURVE_WITH_KNOTS((3,3),(0.218746031477163,0.271795897845352),
 .UNSPECIFIED.)
CURVE()
GEOMETRIC_REPRESENTATION_ITEM()
RATIONAL_B_SPLINE_CURVE((1.02147610369997,1.02311336089465,1.02428162962104))
REPRESENTATION_ITEM('')
);
#316=(
BOUNDED_CURVE()
B_SPLINE_CURVE(2,(#34587,#34588,#34589),.UNSPECIFIED.,.F.,.F.)
B_SPLINE_CURVE_WITH_KNOTS((3,3),(0.536094506482408,0.589144372850588),
 .UNSPECIFIED.)
CURVE()
GEOMETRIC_REPRESENTATION_ITEM()
RATIONAL_B_SPLINE_CURVE((1.02428162962085,1.02311336089447,1.0214761036998))
REPRESENTATION_ITEM('')
);
#317=(
BOUNDED_CURVE()
B_SPLINE_CURVE(2,(#34593,#34594,#34595),.UNSPECIFIED.,.F.,.F.)
B_SPLINE_CURVE_WITH_KNOTS((3,3),(0.218746031477151,0.271795897845338),
 .UNSPECIFIED.)
CURVE()
GEOMETRIC_REPRESENTATION_ITEM()
RATIONAL_B_SPLINE_CURVE((1.02147610369997,1.02311336089465,1.02428162962104))
REPRESENTATION_ITEM('')
);
#318=(
BOUNDED_CURVE()
B_SPLINE_CURVE(2,(#34597,#34598,#34599),.UNSPECIFIED.,.F.,.F.)
B_SPLINE_CURVE_WITH_KNOTS((3,3),(0.536094506482401,0.589144372850584),
 .UNSPECIFIED.)
CURVE()
GEOMETRIC_REPRESENTATION_ITEM()
RATIONAL_B_SPLINE_CURVE((1.02428162962094,1.02311336089455,1.02147610369988))
REPRESENTATION_ITEM('')
);
#319=(
BOUNDED_CURVE()
B_SPLINE_CURVE(2,(#34603,#34604,#34605),.UNSPECIFIED.,.F.,.F.)
B_SPLINE_CURVE_WITH_KNOTS((3,3),(-0.271795897845348,-0.270098893534579),
 .UNSPECIFIED.)
CURVE()
GEOMETRIC_REPRESENTATION_ITEM()
RATIONAL_B_SPLINE_CURVE((1.02428162962101,1.02424425804592,1.02420640656119))
REPRESENTATION_ITEM('')
);
#320=(
BOUNDED_CURVE()
B_SPLINE_CURVE(2,(#34610,#34611,#34612),.UNSPECIFIED.,.F.,.F.)
B_SPLINE_CURVE_WITH_KNOTS((3,3),(-0.270098893534579,-0.218746031477162),
 .UNSPECIFIED.)
CURVE()
GEOMETRIC_REPRESENTATION_ITEM()
RATIONAL_B_SPLINE_CURVE((1.02420640656119,1.02306098691694,1.02147610369995))
REPRESENTATION_ITEM('')
);
#321=(
BOUNDED_CURVE()
B_SPLINE_CURVE(2,(#34614,#34615,#34616),.UNSPECIFIED.,.F.,.F.)
B_SPLINE_CURVE_WITH_KNOTS((3,3),(0.536094506482409,0.589144372850596),
 .UNSPECIFIED.)
CURVE()
GEOMETRIC_REPRESENTATION_ITEM()
RATIONAL_B_SPLINE_CURVE((1.02428162962102,1.02311336089463,1.02147610369996))
REPRESENTATION_ITEM('')
);
#322=(
BOUNDED_CURVE()
B_SPLINE_CURVE(2,(#34620,#34621,#34622),.UNSPECIFIED.,.F.,.F.)
B_SPLINE_CURVE_WITH_KNOTS((3,3),(0.21874603147716,0.271795897845345),
 .UNSPECIFIED.)
CURVE()
GEOMETRIC_REPRESENTATION_ITEM()
RATIONAL_B_SPLINE_CURVE((1.02147610369993,1.0231133608946,1.02428162962099))
REPRESENTATION_ITEM('')
);
#323=(
BOUNDED_CURVE()
B_SPLINE_CURVE(2,(#34624,#34625,#34626),.UNSPECIFIED.,.F.,.F.)
B_SPLINE_CURVE_WITH_KNOTS((3,3),(0.5360945064824,0.589144372850584),
 .UNSPECIFIED.)
CURVE()
GEOMETRIC_REPRESENTATION_ITEM()
RATIONAL_B_SPLINE_CURVE((1.02428162962094,1.02311336089455,1.02147610369988))
REPRESENTATION_ITEM('')
);
#324=(
BOUNDED_CURVE()
B_SPLINE_CURVE(2,(#34630,#34631,#34632),.UNSPECIFIED.,.F.,.F.)
B_SPLINE_CURVE_WITH_KNOTS((3,3),(0.218746031477174,0.271795897845361),
 .UNSPECIFIED.)
CURVE()
GEOMETRIC_REPRESENTATION_ITEM()
RATIONAL_B_SPLINE_CURVE((1.02147610369996,1.02311336089464,1.02428162962103))
REPRESENTATION_ITEM('')
);
#325=(
BOUNDED_CURVE()
B_SPLINE_CURVE(2,(#34634,#34635,#34636),.UNSPECIFIED.,.F.,.F.)
B_SPLINE_CURVE_WITH_KNOTS((3,3),(0.536094506482401,0.589144372850589),
 .UNSPECIFIED.)
CURVE()
GEOMETRIC_REPRESENTATION_ITEM()
RATIONAL_B_SPLINE_CURVE((1.02428162962104,1.02311336089465,1.02147610369997))
REPRESENTATION_ITEM('')
);
#326=(
BOUNDED_CURVE()
B_SPLINE_CURVE(2,(#34640,#34641,#34642),.UNSPECIFIED.,.F.,.F.)
B_SPLINE_CURVE_WITH_KNOTS((3,3),(0.218746031477168,0.271795897845352),
 .UNSPECIFIED.)
CURVE()
GEOMETRIC_REPRESENTATION_ITEM()
RATIONAL_B_SPLINE_CURVE((1.02147610369989,1.02311336089456,1.02428162962095))
REPRESENTATION_ITEM('')
);
#327=(
BOUNDED_CURVE()
B_SPLINE_CURVE(2,(#34644,#34645,#34646),.UNSPECIFIED.,.F.,.F.)
B_SPLINE_CURVE_WITH_KNOTS((3,3),(0.536094506482407,0.589144372850594),
 .UNSPECIFIED.)
CURVE()
GEOMETRIC_REPRESENTATION_ITEM()
RATIONAL_B_SPLINE_CURVE((1.02428162962103,1.02311336089464,1.02147610369996))
REPRESENTATION_ITEM('')
);
#328=(
BOUNDED_CURVE()
B_SPLINE_CURVE(2,(#34650,#34651,#34652),.UNSPECIFIED.,.F.,.F.)
B_SPLINE_CURVE_WITH_KNOTS((3,3),(0.218746031477174,0.27179589784536),
 .UNSPECIFIED.)
CURVE()
GEOMETRIC_REPRESENTATION_ITEM()
RATIONAL_B_SPLINE_CURVE((1.02147610369993,1.02311336089461,1.024281629621))
REPRESENTATION_ITEM('')
);
#329=(
BOUNDED_CURVE()
B_SPLINE_CURVE(2,(#34654,#34655,#34656),.UNSPECIFIED.,.F.,.F.)
B_SPLINE_CURVE_WITH_KNOTS((3,3),(0.536094506482403,0.589144372850591),
 .UNSPECIFIED.)
CURVE()
GEOMETRIC_REPRESENTATION_ITEM()
RATIONAL_B_SPLINE_CURVE((1.02428162962104,1.02311336089464,1.02147610369997))
REPRESENTATION_ITEM('')
);
#330=(
BOUNDED_CURVE()
B_SPLINE_CURVE(2,(#34660,#34661,#34662),.UNSPECIFIED.,.F.,.F.)
B_SPLINE_CURVE_WITH_KNOTS((3,3),(0.218746031477165,0.271795897845354),
 .UNSPECIFIED.)
CURVE()
GEOMETRIC_REPRESENTATION_ITEM()
RATIONAL_B_SPLINE_CURVE((1.02147610370001,1.02311336089469,1.02428162962109))
REPRESENTATION_ITEM('')
);
#331=(
BOUNDED_CURVE()
B_SPLINE_CURVE(2,(#34664,#34665,#34666),.UNSPECIFIED.,.F.,.F.)
B_SPLINE_CURVE_WITH_KNOTS((3,3),(0.536094506482406,0.589144372850589),
 .UNSPECIFIED.)
CURVE()
GEOMETRIC_REPRESENTATION_ITEM()
RATIONAL_B_SPLINE_CURVE((1.02428162962095,1.02311336089456,1.02147610369989))
REPRESENTATION_ITEM('')
);
#332=(
BOUNDED_CURVE()
B_SPLINE_CURVE(2,(#34670,#34671,#34672),.UNSPECIFIED.,.F.,.F.)
B_SPLINE_CURVE_WITH_KNOTS((3,3),(0.218746031477167,0.271795897845354),
 .UNSPECIFIED.)
CURVE()
GEOMETRIC_REPRESENTATION_ITEM()
RATIONAL_B_SPLINE_CURVE((1.02147610369995,1.02311336089462,1.02428162962101))
REPRESENTATION_ITEM('')
);
#333=(
BOUNDED_CURVE()
B_SPLINE_CURVE(2,(#34674,#34675,#34676),.UNSPECIFIED.,.F.,.F.)
B_SPLINE_CURVE_WITH_KNOTS((3,3),(0.536094506482406,0.58914437285059),
 .UNSPECIFIED.)
CURVE()
GEOMETRIC_REPRESENTATION_ITEM()
RATIONAL_B_SPLINE_CURVE((1.02428162962094,1.02311336089456,1.02147610369988))
REPRESENTATION_ITEM('')
);
#334=(
BOUNDED_CURVE()
B_SPLINE_CURVE(2,(#34680,#34681,#34682),.UNSPECIFIED.,.F.,.F.)
B_SPLINE_CURVE_WITH_KNOTS((3,3),(0.218746031477163,0.271795897845349),
 .UNSPECIFIED.)
CURVE()
GEOMETRIC_REPRESENTATION_ITEM()
RATIONAL_B_SPLINE_CURVE((1.02147610369995,1.02311336089462,1.02428162962102))
REPRESENTATION_ITEM('')
);
#335=(
BOUNDED_CURVE()
B_SPLINE_CURVE(2,(#34684,#34685,#34686),.UNSPECIFIED.,.F.,.F.)
B_SPLINE_CURVE_WITH_KNOTS((3,3),(0.536094506482405,0.58914437285059),
 .UNSPECIFIED.)
CURVE()
GEOMETRIC_REPRESENTATION_ITEM()
RATIONAL_B_SPLINE_CURVE((1.02428162962098,1.02311336089459,1.02147610369992))
REPRESENTATION_ITEM('')
);
#336=(
BOUNDED_CURVE()
B_SPLINE_CURVE(2,(#34690,#34691,#34692),.UNSPECIFIED.,.F.,.F.)
B_SPLINE_CURVE_WITH_KNOTS((3,3),(0.21874603147717,0.271795897845354),
 .UNSPECIFIED.)
CURVE()
GEOMETRIC_REPRESENTATION_ITEM()
RATIONAL_B_SPLINE_CURVE((1.0214761036999,1.02311336089457,1.02428162962096))
REPRESENTATION_ITEM('')
);
#337=(
BOUNDED_CURVE()
B_SPLINE_CURVE(2,(#34694,#34695,#34696),.UNSPECIFIED.,.F.,.F.)
B_SPLINE_CURVE_WITH_KNOTS((3,3),(0.536094506482405,0.589144372850589),
 .UNSPECIFIED.)
CURVE()
GEOMETRIC_REPRESENTATION_ITEM()
RATIONAL_B_SPLINE_CURVE((1.02428162962096,1.02311336089458,1.0214761036999))
REPRESENTATION_ITEM('')
);
#338=(
BOUNDED_CURVE()
B_SPLINE_CURVE(2,(#34700,#34701,#34702),.UNSPECIFIED.,.F.,.F.)
B_SPLINE_CURVE_WITH_KNOTS((3,3),(0.218746031477176,0.271795897845357),
 .UNSPECIFIED.)
CURVE()
GEOMETRIC_REPRESENTATION_ITEM()
RATIONAL_B_SPLINE_CURVE((1.02147610369985,1.02311336089452,1.02428162962091))
REPRESENTATION_ITEM('')
);
#339=(
BOUNDED_CURVE()
B_SPLINE_CURVE(2,(#34704,#34705,#34706),.UNSPECIFIED.,.F.,.F.)
B_SPLINE_CURVE_WITH_KNOTS((3,3),(0.536094506482407,0.589144372850591),
 .UNSPECIFIED.)
CURVE()
GEOMETRIC_REPRESENTATION_ITEM()
RATIONAL_B_SPLINE_CURVE((1.02428162962095,1.02311336089456,1.02147610369989))
REPRESENTATION_ITEM('')
);
#340=(
BOUNDED_CURVE()
B_SPLINE_CURVE(2,(#34710,#34711,#34712),.UNSPECIFIED.,.F.,.F.)
B_SPLINE_CURVE_WITH_KNOTS((3,3),(0.218746031477161,0.271795897845349),
 .UNSPECIFIED.)
CURVE()
GEOMETRIC_REPRESENTATION_ITEM()
RATIONAL_B_SPLINE_CURVE((1.02147610369998,1.02311336089466,1.02428162962106))
REPRESENTATION_ITEM('')
);
#341=(
BOUNDED_CURVE()
B_SPLINE_CURVE(2,(#34714,#34715,#34716),.UNSPECIFIED.,.F.,.F.)
B_SPLINE_CURVE_WITH_KNOTS((3,3),(0.536094506482414,0.589144372850592),
 .UNSPECIFIED.)
CURVE()
GEOMETRIC_REPRESENTATION_ITEM()
RATIONAL_B_SPLINE_CURVE((1.02428162962083,1.02311336089444,1.02147610369978))
REPRESENTATION_ITEM('')
);
#342=(
BOUNDED_CURVE()
B_SPLINE_CURVE(2,(#34720,#34721,#34722),.UNSPECIFIED.,.F.,.F.)
B_SPLINE_CURVE_WITH_KNOTS((3,3),(0.218746031477167,0.271795897845358),
 .UNSPECIFIED.)
CURVE()
GEOMETRIC_REPRESENTATION_ITEM()
RATIONAL_B_SPLINE_CURVE((1.02147610370001,1.02311336089469,1.02428162962108))
REPRESENTATION_ITEM('')
);
#343=(
BOUNDED_CURVE()
B_SPLINE_CURVE(2,(#34724,#34725,#34726),.UNSPECIFIED.,.F.,.F.)
B_SPLINE_CURVE_WITH_KNOTS((3,3),(0.536094506482411,0.589144372850593),
 .UNSPECIFIED.)
CURVE()
GEOMETRIC_REPRESENTATION_ITEM()
RATIONAL_B_SPLINE_CURVE((1.02428162962092,1.02311336089453,1.02147610369986))
REPRESENTATION_ITEM('')
);
#344=(
BOUNDED_CURVE()
B_SPLINE_CURVE(2,(#34730,#34731,#34732),.UNSPECIFIED.,.F.,.F.)
B_SPLINE_CURVE_WITH_KNOTS((3,3),(0.21874603147718,0.27179589784536),
 .UNSPECIFIED.)
CURVE()
GEOMETRIC_REPRESENTATION_ITEM()
RATIONAL_B_SPLINE_CURVE((1.02147610369982,1.02311336089449,1.02428162962087))
REPRESENTATION_ITEM('')
);
#345=(
BOUNDED_CURVE()
B_SPLINE_CURVE(2,(#34734,#34735,#34736),.UNSPECIFIED.,.F.,.F.)
B_SPLINE_CURVE_WITH_KNOTS((3,3),(0.536094506482394,0.589144372850576),
 .UNSPECIFIED.)
CURVE()
GEOMETRIC_REPRESENTATION_ITEM()
RATIONAL_B_SPLINE_CURVE((1.0242816296209,1.02311336089451,1.02147610369985))
REPRESENTATION_ITEM('')
);
#346=(
BOUNDED_CURVE()
B_SPLINE_CURVE(2,(#34740,#34741,#34742),.UNSPECIFIED.,.F.,.F.)
B_SPLINE_CURVE_WITH_KNOTS((3,3),(0.218746031477168,0.271795897845353),
 .UNSPECIFIED.)
CURVE()
GEOMETRIC_REPRESENTATION_ITEM()
RATIONAL_B_SPLINE_CURVE((1.02147610369992,1.0231133608946,1.02428162962099))
REPRESENTATION_ITEM('')
);
#347=(
BOUNDED_CURVE()
B_SPLINE_CURVE(2,(#34744,#34745,#34746),.UNSPECIFIED.,.F.,.F.)
B_SPLINE_CURVE_WITH_KNOTS((3,3),(0.536094506482401,0.589144372850586),
 .UNSPECIFIED.)
CURVE()
GEOMETRIC_REPRESENTATION_ITEM()
RATIONAL_B_SPLINE_CURVE((1.02428162962097,1.02311336089458,1.02147610369991))
REPRESENTATION_ITEM('')
);
#348=(
BOUNDED_CURVE()
B_SPLINE_CURVE(2,(#34750,#34751,#34752),.UNSPECIFIED.,.F.,.F.)
B_SPLINE_CURVE_WITH_KNOTS((3,3),(0.218746031477169,0.271795897845357),
 .UNSPECIFIED.)
CURVE()
GEOMETRIC_REPRESENTATION_ITEM()
RATIONAL_B_SPLINE_CURVE((1.02147610369996,1.02311336089463,1.02428162962103))
REPRESENTATION_ITEM('')
);
#349=(
BOUNDED_CURVE()
B_SPLINE_CURVE(2,(#34754,#34755,#34756),.UNSPECIFIED.,.F.,.F.)
B_SPLINE_CURVE_WITH_KNOTS((3,3),(0.53609450648239,0.589144372850573),
 .UNSPECIFIED.)
CURVE()
GEOMETRIC_REPRESENTATION_ITEM()
RATIONAL_B_SPLINE_CURVE((1.02428162962093,1.02311336089454,1.02147610369987))
REPRESENTATION_ITEM('')
);
#350=(
BOUNDED_CURVE()
B_SPLINE_CURVE(2,(#34760,#34761,#34762),.UNSPECIFIED.,.F.,.F.)
B_SPLINE_CURVE_WITH_KNOTS((3,3),(0.218746031477159,0.271795897845342),
 .UNSPECIFIED.)
CURVE()
GEOMETRIC_REPRESENTATION_ITEM()
RATIONAL_B_SPLINE_CURVE((1.02147610369989,1.02311336089456,1.02428162962095))
REPRESENTATION_ITEM('')
);
#351=(
BOUNDED_CURVE()
B_SPLINE_CURVE(2,(#34764,#34765,#34766),.UNSPECIFIED.,.F.,.F.)
B_SPLINE_CURVE_WITH_KNOTS((3,3),(0.536094506482392,0.58914437285058),
 .UNSPECIFIED.)
CURVE()
GEOMETRIC_REPRESENTATION_ITEM()
RATIONAL_B_SPLINE_CURVE((1.02428162962103,1.02311336089464,1.02147610369996))
REPRESENTATION_ITEM('')
);
#352=(
BOUNDED_CURVE()
B_SPLINE_CURVE(2,(#34770,#34771,#34772),.UNSPECIFIED.,.F.,.F.)
B_SPLINE_CURVE_WITH_KNOTS((3,3),(0.218746031477161,0.271795897845349),
 .UNSPECIFIED.)
CURVE()
GEOMETRIC_REPRESENTATION_ITEM()
RATIONAL_B_SPLINE_CURVE((1.02147610369998,1.02311336089466,1.02428162962105))
REPRESENTATION_ITEM('')
);
#353=(
BOUNDED_CURVE()
B_SPLINE_CURVE(2,(#34774,#34775,#34776),.UNSPECIFIED.,.F.,.F.)
B_SPLINE_CURVE_WITH_KNOTS((3,3),(0.536094506482406,0.589144372850593),
 .UNSPECIFIED.)
CURVE()
GEOMETRIC_REPRESENTATION_ITEM()
RATIONAL_B_SPLINE_CURVE((1.024281629621,1.02311336089461,1.02147610369993))
REPRESENTATION_ITEM('')
);
#354=(
BOUNDED_CURVE()
B_SPLINE_CURVE(2,(#34780,#34781,#34782),.UNSPECIFIED.,.F.,.F.)
B_SPLINE_CURVE_WITH_KNOTS((3,3),(0.218746031477174,0.271795897845361),
 .UNSPECIFIED.)
CURVE()
GEOMETRIC_REPRESENTATION_ITEM()
RATIONAL_B_SPLINE_CURVE((1.02147610369995,1.02311336089462,1.02428162962101))
REPRESENTATION_ITEM('')
);
#355=(
BOUNDED_CURVE()
B_SPLINE_CURVE(2,(#34784,#34785,#34786),.UNSPECIFIED.,.F.,.F.)
B_SPLINE_CURVE_WITH_KNOTS((3,3),(0.536094506482403,0.589144372850589),
 .UNSPECIFIED.)
CURVE()
GEOMETRIC_REPRESENTATION_ITEM()
RATIONAL_B_SPLINE_CURVE((1.02428162962099,1.0231133608946,1.02147610369993))
REPRESENTATION_ITEM('')
);
#356=(
BOUNDED_CURVE()
B_SPLINE_CURVE(2,(#34790,#34791,#34792),.UNSPECIFIED.,.F.,.F.)
B_SPLINE_CURVE_WITH_KNOTS((3,3),(0.218746031477177,0.271795897845364),
 .UNSPECIFIED.)
CURVE()
GEOMETRIC_REPRESENTATION_ITEM()
RATIONAL_B_SPLINE_CURVE((1.0214761036999,1.02311336089457,1.02428162962096))
REPRESENTATION_ITEM('')
);
#357=(
BOUNDED_CURVE()
B_SPLINE_CURVE(2,(#34794,#34795,#34796),.UNSPECIFIED.,.F.,.F.)
B_SPLINE_CURVE_WITH_KNOTS((3,3),(0.536094506482414,0.589144372850605),
 .UNSPECIFIED.)
CURVE()
GEOMETRIC_REPRESENTATION_ITEM()
RATIONAL_B_SPLINE_CURVE((1.02428162962111,1.02311336089472,1.02147610370003))
REPRESENTATION_ITEM('')
);
#358=(
BOUNDED_CURVE()
B_SPLINE_CURVE(2,(#34800,#34801,#34802),.UNSPECIFIED.,.F.,.F.)
B_SPLINE_CURVE_WITH_KNOTS((3,3),(0.218746031477174,0.271795897845363),
 .UNSPECIFIED.)
CURVE()
GEOMETRIC_REPRESENTATION_ITEM()
RATIONAL_B_SPLINE_CURVE((1.02147610369998,1.02311336089465,1.02428162962105))
REPRESENTATION_ITEM('')
);
#359=(
BOUNDED_CURVE()
B_SPLINE_CURVE(2,(#34804,#34805,#34806),.UNSPECIFIED.,.F.,.F.)
B_SPLINE_CURVE_WITH_KNOTS((3,3),(0.536094506482404,0.589144372850588),
 .UNSPECIFIED.)
CURVE()
GEOMETRIC_REPRESENTATION_ITEM()
RATIONAL_B_SPLINE_CURVE((1.02428162962096,1.02311336089458,1.0214761036999))
REPRESENTATION_ITEM('')
);
#360=(
BOUNDED_CURVE()
B_SPLINE_CURVE(2,(#34810,#34811,#34812),.UNSPECIFIED.,.F.,.F.)
B_SPLINE_CURVE_WITH_KNOTS((3,3),(0.218746031477183,0.271795897845364),
 .UNSPECIFIED.)
CURVE()
GEOMETRIC_REPRESENTATION_ITEM()
RATIONAL_B_SPLINE_CURVE((1.02147610369985,1.02311336089452,1.0242816296209))
REPRESENTATION_ITEM('')
);
#361=(
BOUNDED_CURVE()
B_SPLINE_CURVE(2,(#34814,#34815,#34816),.UNSPECIFIED.,.F.,.F.)
B_SPLINE_CURVE_WITH_KNOTS((3,3),(0.536094506482398,0.589144372850582),
 .UNSPECIFIED.)
CURVE()
GEOMETRIC_REPRESENTATION_ITEM()
RATIONAL_B_SPLINE_CURVE((1.02428162962094,1.02311336089455,1.02147610369988))
REPRESENTATION_ITEM('')
);
#362=(
BOUNDED_CURVE()
B_SPLINE_CURVE(2,(#34820,#34821,#34822),.UNSPECIFIED.,.F.,.F.)
B_SPLINE_CURVE_WITH_KNOTS((3,3),(0.21874603147717,0.271795897845347),
 .UNSPECIFIED.)
CURVE()
GEOMETRIC_REPRESENTATION_ITEM()
RATIONAL_B_SPLINE_CURVE((1.0214761036998,1.02311336089446,1.02428162962084))
REPRESENTATION_ITEM('')
);
#363=(
BOUNDED_CURVE()
B_SPLINE_CURVE(2,(#34824,#34825,#34826),.UNSPECIFIED.,.F.,.F.)
B_SPLINE_CURVE_WITH_KNOTS((3,3),(0.536094506482403,0.589144372850584),
 .UNSPECIFIED.)
CURVE()
GEOMETRIC_REPRESENTATION_ITEM()
RATIONAL_B_SPLINE_CURVE((1.02428162962089,1.02311336089451,1.02147610369984))
REPRESENTATION_ITEM('')
);
#364=(
BOUNDED_CURVE()
B_SPLINE_CURVE(2,(#34830,#34831,#34832),.UNSPECIFIED.,.F.,.F.)
B_SPLINE_CURVE_WITH_KNOTS((3,3),(0.218746031477161,0.271795897845346),
 .UNSPECIFIED.)
CURVE()
GEOMETRIC_REPRESENTATION_ITEM()
RATIONAL_B_SPLINE_CURVE((1.02147610369993,1.0231133608946,1.024281629621))
REPRESENTATION_ITEM('')
);
#365=(
BOUNDED_CURVE()
B_SPLINE_CURVE(2,(#34834,#34835,#34836),.UNSPECIFIED.,.F.,.F.)
B_SPLINE_CURVE_WITH_KNOTS((3,3),(0.53609450648241,0.589144372850597),
 .UNSPECIFIED.)
CURVE()
GEOMETRIC_REPRESENTATION_ITEM()
RATIONAL_B_SPLINE_CURVE((1.02428162962105,1.02311336089465,1.02147610369997))
REPRESENTATION_ITEM('')
);
#366=(
BOUNDED_CURVE()
B_SPLINE_CURVE(2,(#34840,#34841,#34842),.UNSPECIFIED.,.F.,.F.)
B_SPLINE_CURVE_WITH_KNOTS((3,3),(0.21874603147718,0.271795897845363),
 .UNSPECIFIED.)
CURVE()
GEOMETRIC_REPRESENTATION_ITEM()
RATIONAL_B_SPLINE_CURVE((1.02147610369987,1.02311336089453,1.02428162962092))
REPRESENTATION_ITEM('')
);
#367=(
BOUNDED_CURVE()
B_SPLINE_CURVE(2,(#34844,#34845,#34846),.UNSPECIFIED.,.F.,.F.)
B_SPLINE_CURVE_WITH_KNOTS((3,3),(0.536094506482391,0.589144372850573),
 .UNSPECIFIED.)
CURVE()
GEOMETRIC_REPRESENTATION_ITEM()
RATIONAL_B_SPLINE_CURVE((1.02428162962087,1.02311336089449,1.02147610369982))
REPRESENTATION_ITEM('')
);
#368=(
BOUNDED_CURVE()
B_SPLINE_CURVE(2,(#34850,#34851,#34852),.UNSPECIFIED.,.F.,.F.)
B_SPLINE_CURVE_WITH_KNOTS((3,3),(0.218746031477181,0.271795897845364),
 .UNSPECIFIED.)
CURVE()
GEOMETRIC_REPRESENTATION_ITEM()
RATIONAL_B_SPLINE_CURVE((1.02147610369986,1.02311336089452,1.02428162962091))
REPRESENTATION_ITEM('')
);
#369=(
BOUNDED_CURVE()
B_SPLINE_CURVE(2,(#34854,#34855,#34856),.UNSPECIFIED.,.F.,.F.)
B_SPLINE_CURVE_WITH_KNOTS((3,3),(0.536094506482413,0.589144372850602),
 .UNSPECIFIED.)
CURVE()
GEOMETRIC_REPRESENTATION_ITEM()
RATIONAL_B_SPLINE_CURVE((1.02428162962106,1.02311336089467,1.02147610369999))
REPRESENTATION_ITEM('')
);
#370=(
BOUNDED_CURVE()
B_SPLINE_CURVE(2,(#34860,#34861,#34862),.UNSPECIFIED.,.F.,.F.)
B_SPLINE_CURVE_WITH_KNOTS((3,3),(0.218746031477165,0.271795897845346),
 .UNSPECIFIED.)
CURVE()
GEOMETRIC_REPRESENTATION_ITEM()
RATIONAL_B_SPLINE_CURVE((1.02147610369987,1.02311336089454,1.02428162962093))
REPRESENTATION_ITEM('')
);
#371=(
BOUNDED_CURVE()
B_SPLINE_CURVE(2,(#34864,#34865,#34866),.UNSPECIFIED.,.F.,.F.)
B_SPLINE_CURVE_WITH_KNOTS((3,3),(0.53609450648241,0.589144372850598),
 .UNSPECIFIED.)
CURVE()
GEOMETRIC_REPRESENTATION_ITEM()
RATIONAL_B_SPLINE_CURVE((1.02428162962105,1.02311336089466,1.02147610369998))
REPRESENTATION_ITEM('')
);
#372=(
BOUNDED_CURVE()
B_SPLINE_CURVE(2,(#34870,#34871,#34872),.UNSPECIFIED.,.F.,.F.)
B_SPLINE_CURVE_WITH_KNOTS((3,3),(0.21874603147717,0.271795897845357),
 .UNSPECIFIED.)
CURVE()
GEOMETRIC_REPRESENTATION_ITEM()
RATIONAL_B_SPLINE_CURVE((1.02147610369995,1.02311336089463,1.02428162962102))
REPRESENTATION_ITEM('')
);
#373=(
BOUNDED_CURVE()
B_SPLINE_CURVE(2,(#34874,#34875,#34876),.UNSPECIFIED.,.F.,.F.)
B_SPLINE_CURVE_WITH_KNOTS((3,3),(0.536094506482409,0.589144372850597),
 .UNSPECIFIED.)
CURVE()
GEOMETRIC_REPRESENTATION_ITEM()
RATIONAL_B_SPLINE_CURVE((1.02428162962106,1.02311336089466,1.02147610369998))
REPRESENTATION_ITEM('')
);
#374=(
BOUNDED_CURVE()
B_SPLINE_CURVE(2,(#34880,#34881,#34882),.UNSPECIFIED.,.F.,.F.)
B_SPLINE_CURVE_WITH_KNOTS((3,3),(0.21874603147717,0.271795897845356),
 .UNSPECIFIED.)
CURVE()
GEOMETRIC_REPRESENTATION_ITEM()
RATIONAL_B_SPLINE_CURVE((1.02147610369992,1.02311336089459,1.02428162962098))
REPRESENTATION_ITEM('')
);
#375=(
BOUNDED_CURVE()
B_SPLINE_CURVE(2,(#34884,#34885,#34886),.UNSPECIFIED.,.F.,.F.)
B_SPLINE_CURVE_WITH_KNOTS((3,3),(0.536094506482409,0.589144372850597),
 .UNSPECIFIED.)
CURVE()
GEOMETRIC_REPRESENTATION_ITEM()
RATIONAL_B_SPLINE_CURVE((1.02428162962106,1.02311336089467,1.02147610369999))
REPRESENTATION_ITEM('')
);
#376=(
BOUNDED_CURVE()
B_SPLINE_CURVE(2,(#34890,#34891,#34892),.UNSPECIFIED.,.F.,.F.)
B_SPLINE_CURVE_WITH_KNOTS((3,3),(0.218746031477176,0.271795897845358),
 .UNSPECIFIED.)
CURVE()
GEOMETRIC_REPRESENTATION_ITEM()
RATIONAL_B_SPLINE_CURVE((1.02147610369985,1.02311336089452,1.0242816296209))
REPRESENTATION_ITEM('')
);
#377=(
BOUNDED_CURVE()
B_SPLINE_CURVE(2,(#34894,#34895,#34896),.UNSPECIFIED.,.F.,.F.)
B_SPLINE_CURVE_WITH_KNOTS((3,3),(0.536094506482385,0.589144372850568),
 .UNSPECIFIED.)
CURVE()
GEOMETRIC_REPRESENTATION_ITEM()
RATIONAL_B_SPLINE_CURVE((1.02428162962089,1.0231133608945,1.02147610369984))
REPRESENTATION_ITEM('')
);
#378=(
BOUNDED_CURVE()
B_SPLINE_CURVE(2,(#34900,#34901,#34902),.UNSPECIFIED.,.F.,.F.)
B_SPLINE_CURVE_WITH_KNOTS((3,3),(0.218746031477173,0.271795897845358),
 .UNSPECIFIED.)
CURVE()
GEOMETRIC_REPRESENTATION_ITEM()
RATIONAL_B_SPLINE_CURVE((1.02147610369988,1.02311336089455,1.02428162962094))
REPRESENTATION_ITEM('')
);
#379=(
BOUNDED_CURVE()
B_SPLINE_CURVE(2,(#34904,#34905,#34906),.UNSPECIFIED.,.F.,.F.)
B_SPLINE_CURVE_WITH_KNOTS((3,3),(0.536094506482398,0.589144372850582),
 .UNSPECIFIED.)
CURVE()
GEOMETRIC_REPRESENTATION_ITEM()
RATIONAL_B_SPLINE_CURVE((1.02428162962091,1.02311336089453,1.02147610369986))
REPRESENTATION_ITEM('')
);
#380=(
BOUNDED_CURVE()
B_SPLINE_CURVE(2,(#34910,#34911,#34912),.UNSPECIFIED.,.F.,.F.)
B_SPLINE_CURVE_WITH_KNOTS((3,3),(0.218746031477167,0.271795897845352),
 .UNSPECIFIED.)
CURVE()
GEOMETRIC_REPRESENTATION_ITEM()
RATIONAL_B_SPLINE_CURVE((1.02147610369992,1.0231133608946,1.02428162962099))
REPRESENTATION_ITEM('')
);
#381=(
BOUNDED_CURVE()
B_SPLINE_CURVE(2,(#34914,#34915,#34916),.UNSPECIFIED.,.F.,.F.)
B_SPLINE_CURVE_WITH_KNOTS((3,3),(0.536094506482388,0.589144372850568),
 .UNSPECIFIED.)
CURVE()
GEOMETRIC_REPRESENTATION_ITEM()
RATIONAL_B_SPLINE_CURVE((1.02428162962083,1.02311336089444,1.02147610369978))
REPRESENTATION_ITEM('')
);
#382=(
BOUNDED_CURVE()
B_SPLINE_CURVE(2,(#34920,#34921,#34922),.UNSPECIFIED.,.F.,.F.)
B_SPLINE_CURVE_WITH_KNOTS((3,3),(0.218746031477159,0.271795897845343),
 .UNSPECIFIED.)
CURVE()
GEOMETRIC_REPRESENTATION_ITEM()
RATIONAL_B_SPLINE_CURVE((1.02147610369992,1.02311336089459,1.02428162962098))
REPRESENTATION_ITEM('')
);
#383=(
BOUNDED_CURVE()
B_SPLINE_CURVE(2,(#34924,#34925,#34926),.UNSPECIFIED.,.F.,.F.)
B_SPLINE_CURVE_WITH_KNOTS((3,3),(0.536094506482409,0.589144372850598),
 .UNSPECIFIED.)
CURVE()
GEOMETRIC_REPRESENTATION_ITEM()
RATIONAL_B_SPLINE_CURVE((1.02428162962104,1.02311336089465,1.02147610369997))
REPRESENTATION_ITEM('')
);
#384=(
BOUNDED_CURVE()
B_SPLINE_CURVE(2,(#34930,#34931,#34932),.UNSPECIFIED.,.F.,.F.)
B_SPLINE_CURVE_WITH_KNOTS((3,3),(0.218746031477167,0.271795897845353),
 .UNSPECIFIED.)
CURVE()
GEOMETRIC_REPRESENTATION_ITEM()
RATIONAL_B_SPLINE_CURVE((1.02147610369994,1.02311336089461,1.024281629621))
REPRESENTATION_ITEM('')
);
#385=(
BOUNDED_CURVE()
B_SPLINE_CURVE(2,(#34934,#34935,#34936),.UNSPECIFIED.,.F.,.F.)
B_SPLINE_CURVE_WITH_KNOTS((3,3),(0.536094506482415,0.589144372850595),
 .UNSPECIFIED.)
CURVE()
GEOMETRIC_REPRESENTATION_ITEM()
RATIONAL_B_SPLINE_CURVE((1.0242816296209,1.02311336089451,1.02147610369984))
REPRESENTATION_ITEM('')
);
#386=(
BOUNDED_CURVE()
B_SPLINE_CURVE(2,(#34940,#34941,#34942),.UNSPECIFIED.,.F.,.F.)
B_SPLINE_CURVE_WITH_KNOTS((3,3),(0.218746031477164,0.271795897845348),
 .UNSPECIFIED.)
CURVE()
GEOMETRIC_REPRESENTATION_ITEM()
RATIONAL_B_SPLINE_CURVE((1.02147610369991,1.02311336089458,1.02428162962097))
REPRESENTATION_ITEM('')
);
#387=(
BOUNDED_CURVE()
B_SPLINE_CURVE(2,(#34944,#34945,#34946),.UNSPECIFIED.,.F.,.F.)
B_SPLINE_CURVE_WITH_KNOTS((3,3),(0.536094506482408,0.589144372850597),
 .UNSPECIFIED.)
CURVE()
GEOMETRIC_REPRESENTATION_ITEM()
RATIONAL_B_SPLINE_CURVE((1.02428162962106,1.02311336089466,1.02147610369999))
REPRESENTATION_ITEM('')
);
#388=(
BOUNDED_CURVE()
B_SPLINE_CURVE(2,(#34950,#34951,#34952),.UNSPECIFIED.,.F.,.F.)
B_SPLINE_CURVE_WITH_KNOTS((3,3),(0.218746031477166,0.271795897845352),
 .UNSPECIFIED.)
CURVE()
GEOMETRIC_REPRESENTATION_ITEM()
RATIONAL_B_SPLINE_CURVE((1.02147610369992,1.0231133608946,1.02428162962099))
REPRESENTATION_ITEM('')
);
#389=(
BOUNDED_CURVE()
B_SPLINE_CURVE(2,(#34954,#34955,#34956),.UNSPECIFIED.,.F.,.F.)
B_SPLINE_CURVE_WITH_KNOTS((3,3),(0.536094506482395,0.589144372850571),
 .UNSPECIFIED.)
CURVE()
GEOMETRIC_REPRESENTATION_ITEM()
RATIONAL_B_SPLINE_CURVE((1.02428162962077,1.02311336089439,1.02147610369973))
REPRESENTATION_ITEM('')
);
#390=(
BOUNDED_CURVE()
B_SPLINE_CURVE(2,(#34960,#34961,#34962),.UNSPECIFIED.,.F.,.F.)
B_SPLINE_CURVE_WITH_KNOTS((3,3),(0.218746031477178,0.27179589784536),
 .UNSPECIFIED.)
CURVE()
GEOMETRIC_REPRESENTATION_ITEM()
RATIONAL_B_SPLINE_CURVE((1.02147610369982,1.02311336089448,1.02428162962087))
REPRESENTATION_ITEM('')
);
#391=(
BOUNDED_CURVE()
B_SPLINE_CURVE(2,(#34964,#34965,#34966),.UNSPECIFIED.,.F.,.F.)
B_SPLINE_CURVE_WITH_KNOTS((3,3),(0.536094506482417,0.589144372850603),
 .UNSPECIFIED.)
CURVE()
GEOMETRIC_REPRESENTATION_ITEM()
RATIONAL_B_SPLINE_CURVE((1.02428162962101,1.02311336089462,1.02147610369994))
REPRESENTATION_ITEM('')
);
#392=(
BOUNDED_CURVE()
B_SPLINE_CURVE(2,(#34970,#34971,#34972),.UNSPECIFIED.,.F.,.F.)
B_SPLINE_CURVE_WITH_KNOTS((3,3),(0.218746031477165,0.271795897845348),
 .UNSPECIFIED.)
CURVE()
GEOMETRIC_REPRESENTATION_ITEM()
RATIONAL_B_SPLINE_CURVE((1.02147610369987,1.02311336089454,1.02428162962093))
REPRESENTATION_ITEM('')
);
#393=(
BOUNDED_CURVE()
B_SPLINE_CURVE(2,(#34974,#34975,#34976),.UNSPECIFIED.,.F.,.F.)
B_SPLINE_CURVE_WITH_KNOTS((3,3),(0.536094506482408,0.589144372850592),
 .UNSPECIFIED.)
CURVE()
GEOMETRIC_REPRESENTATION_ITEM()
RATIONAL_B_SPLINE_CURVE((1.02428162962092,1.02311336089454,1.02147610369987))
REPRESENTATION_ITEM('')
);
#394=(
BOUNDED_CURVE()
B_SPLINE_CURVE(2,(#34980,#34981,#34982),.UNSPECIFIED.,.F.,.F.)
B_SPLINE_CURVE_WITH_KNOTS((3,3),(0.218746031477181,0.271795897845365),
 .UNSPECIFIED.)
CURVE()
GEOMETRIC_REPRESENTATION_ITEM()
RATIONAL_B_SPLINE_CURVE((1.02147610369986,1.02311336089453,1.02428162962092))
REPRESENTATION_ITEM('')
);
#395=(
BOUNDED_CURVE()
B_SPLINE_CURVE(2,(#34984,#34985,#34986),.UNSPECIFIED.,.F.,.F.)
B_SPLINE_CURVE_WITH_KNOTS((3,3),(0.536094506482407,0.589144372850588),
 .UNSPECIFIED.)
CURVE()
GEOMETRIC_REPRESENTATION_ITEM()
RATIONAL_B_SPLINE_CURVE((1.02428162962089,1.0231133608945,1.02147610369984))
REPRESENTATION_ITEM('')
);
#396=(
BOUNDED_CURVE()
B_SPLINE_CURVE(2,(#34989,#34990,#34991),.UNSPECIFIED.,.F.,.F.)
B_SPLINE_CURVE_WITH_KNOTS((3,3),(0.218746031477154,0.27179589784534),
 .UNSPECIFIED.)
CURVE()
GEOMETRIC_REPRESENTATION_ITEM()
RATIONAL_B_SPLINE_CURVE((1.02147610369997,1.02311336089464,1.02428162962104))
REPRESENTATION_ITEM('')
);
#397=(
BOUNDED_CURVE()
B_SPLINE_CURVE(2,(#34995,#34996,#34997),.UNSPECIFIED.,.F.,.F.)
B_SPLINE_CURVE_WITH_KNOTS((3,3),(0.536094506482396,0.589144372850575),
 .UNSPECIFIED.)
CURVE()
GEOMETRIC_REPRESENTATION_ITEM()
RATIONAL_B_SPLINE_CURVE((1.02428162962084,1.02311336089446,1.0214761036998))
REPRESENTATION_ITEM('')
);
#398=(
BOUNDED_CURVE()
B_SPLINE_CURVE(2,(#35001,#35002,#35003),.UNSPECIFIED.,.F.,.F.)
B_SPLINE_CURVE_WITH_KNOTS((3,3),(-0.271795897845359,-0.218746031477171),
 .UNSPECIFIED.)
CURVE()
GEOMETRIC_REPRESENTATION_ITEM()
RATIONAL_B_SPLINE_CURVE((1.02428162962104,1.02311336089465,1.02147610369997))
REPRESENTATION_ITEM('')
);
#399=(
BOUNDED_CURVE()
B_SPLINE_CURVE(2,(#35005,#35006,#35007),.UNSPECIFIED.,.F.,.F.)
B_SPLINE_CURVE_WITH_KNOTS((3,3),(-0.589144372850596,-0.536094506482412),
 .UNSPECIFIED.)
CURVE()
GEOMETRIC_REPRESENTATION_ITEM()
RATIONAL_B_SPLINE_CURVE((1.02147610369993,1.02311336089461,1.024281629621))
REPRESENTATION_ITEM('')
);
#400=(
BOUNDED_CURVE()
B_SPLINE_CURVE(2,(#35011,#35012,#35013),.UNSPECIFIED.,.F.,.F.)
B_SPLINE_CURVE_WITH_KNOTS((3,3),(-0.271795897845366,-0.218746031477182),
 .UNSPECIFIED.)
CURVE()
GEOMETRIC_REPRESENTATION_ITEM()
RATIONAL_B_SPLINE_CURVE((1.02428162962093,1.02311336089455,1.02147610369988))
REPRESENTATION_ITEM('')
);
#401=(
BOUNDED_CURVE()
B_SPLINE_CURVE(2,(#35015,#35016,#35017),.UNSPECIFIED.,.F.,.F.)
B_SPLINE_CURVE_WITH_KNOTS((3,3),(-0.589144372850618,-0.53609450648243),
 .UNSPECIFIED.)
CURVE()
GEOMETRIC_REPRESENTATION_ITEM()
RATIONAL_B_SPLINE_CURVE((1.02147610370001,1.02311336089469,1.02428162962108))
REPRESENTATION_ITEM('')
);
#402=(
BOUNDED_CURVE()
B_SPLINE_CURVE(2,(#35021,#35022,#35023),.UNSPECIFIED.,.F.,.F.)
B_SPLINE_CURVE_WITH_KNOTS((3,3),(-0.271795897845358,-0.218746031477173),
 .UNSPECIFIED.)
CURVE()
GEOMETRIC_REPRESENTATION_ITEM()
RATIONAL_B_SPLINE_CURVE((1.02428162962097,1.02311336089459,1.02147610369991))
REPRESENTATION_ITEM('')
);
#403=(
BOUNDED_CURVE()
B_SPLINE_CURVE(2,(#35025,#35026,#35027),.UNSPECIFIED.,.F.,.F.)
B_SPLINE_CURVE_WITH_KNOTS((3,3),(-0.589144372850595,-0.53609450648241),
 .UNSPECIFIED.)
CURVE()
GEOMETRIC_REPRESENTATION_ITEM()
RATIONAL_B_SPLINE_CURVE((1.02147610369992,1.0231133608946,1.02428162962099))
REPRESENTATION_ITEM('')
);
#404=(
BOUNDED_CURVE()
B_SPLINE_CURVE(2,(#35031,#35032,#35033),.UNSPECIFIED.,.F.,.F.)
B_SPLINE_CURVE_WITH_KNOTS((3,3),(-0.271795897845356,-0.218746031477171),
 .UNSPECIFIED.)
CURVE()
GEOMETRIC_REPRESENTATION_ITEM()
RATIONAL_B_SPLINE_CURVE((1.024281629621,1.02311336089461,1.02147610369993))
REPRESENTATION_ITEM('')
);
#405=(
BOUNDED_CURVE()
B_SPLINE_CURVE(2,(#35035,#35036,#35037),.UNSPECIFIED.,.F.,.F.)
B_SPLINE_CURVE_WITH_KNOTS((3,3),(-0.589144372850588,-0.536094506482404),
 .UNSPECIFIED.)
CURVE()
GEOMETRIC_REPRESENTATION_ITEM()
RATIONAL_B_SPLINE_CURVE((1.0214761036999,1.02311336089458,1.02428162962097))
REPRESENTATION_ITEM('')
);
#406=(
BOUNDED_CURVE()
B_SPLINE_CURVE(2,(#35041,#35042,#35043),.UNSPECIFIED.,.F.,.F.)
B_SPLINE_CURVE_WITH_KNOTS((3,3),(-0.271795897845343,-0.218746031477154),
 .UNSPECIFIED.)
CURVE()
GEOMETRIC_REPRESENTATION_ITEM()
RATIONAL_B_SPLINE_CURVE((1.02428162962107,1.02311336089467,1.02147610369999))
REPRESENTATION_ITEM('')
);
#407=(
BOUNDED_CURVE()
B_SPLINE_CURVE(2,(#35045,#35046,#35047),.UNSPECIFIED.,.F.,.F.)
B_SPLINE_CURVE_WITH_KNOTS((3,3),(-0.589144372850603,-0.536094506482417),
 .UNSPECIFIED.)
CURVE()
GEOMETRIC_REPRESENTATION_ITEM()
RATIONAL_B_SPLINE_CURVE((1.02147610369995,1.02311336089463,1.02428162962102))
REPRESENTATION_ITEM('')
);
#408=(
BOUNDED_CURVE()
B_SPLINE_CURVE(2,(#35051,#35052,#35053),.UNSPECIFIED.,.F.,.F.)
B_SPLINE_CURVE_WITH_KNOTS((3,3),(-0.271795897845354,-0.218746031477172),
 .UNSPECIFIED.)
CURVE()
GEOMETRIC_REPRESENTATION_ITEM()
RATIONAL_B_SPLINE_CURVE((1.02428162962093,1.02311336089455,1.02147610369988))
REPRESENTATION_ITEM('')
);
#409=(
BOUNDED_CURVE()
B_SPLINE_CURVE(2,(#35055,#35056,#35057),.UNSPECIFIED.,.F.,.F.)
B_SPLINE_CURVE_WITH_KNOTS((3,3),(-0.589144372850597,-0.536094506482412),
 .UNSPECIFIED.)
CURVE()
GEOMETRIC_REPRESENTATION_ITEM()
RATIONAL_B_SPLINE_CURVE((1.02147610369993,1.02311336089461,1.024281629621))
REPRESENTATION_ITEM('')
);
#410=(
BOUNDED_CURVE()
B_SPLINE_CURVE(2,(#35061,#35062,#35063),.UNSPECIFIED.,.F.,.F.)
B_SPLINE_CURVE_WITH_KNOTS((3,3),(-0.271795897845357,-0.218746031477169),
 .UNSPECIFIED.)
CURVE()
GEOMETRIC_REPRESENTATION_ITEM()
RATIONAL_B_SPLINE_CURVE((1.02428162962103,1.02311336089464,1.02147610369996))
REPRESENTATION_ITEM('')
);
#411=(
BOUNDED_CURVE()
B_SPLINE_CURVE(2,(#35065,#35066,#35067),.UNSPECIFIED.,.F.,.F.)
B_SPLINE_CURVE_WITH_KNOTS((3,3),(-0.589144372850578,-0.536094506482397),
 .UNSPECIFIED.)
CURVE()
GEOMETRIC_REPRESENTATION_ITEM()
RATIONAL_B_SPLINE_CURVE((1.02147610369984,1.02311336089451,1.02428162962089))
REPRESENTATION_ITEM('')
);
#412=(
BOUNDED_CURVE()
B_SPLINE_CURVE(2,(#35071,#35072,#35073),.UNSPECIFIED.,.F.,.F.)
B_SPLINE_CURVE_WITH_KNOTS((3,3),(-0.271795897845352,-0.21874603147717),
 .UNSPECIFIED.)
CURVE()
GEOMETRIC_REPRESENTATION_ITEM()
RATIONAL_B_SPLINE_CURVE((1.02428162962095,1.02311336089456,1.02147610369989))
REPRESENTATION_ITEM('')
);
#413=(
BOUNDED_CURVE()
B_SPLINE_CURVE(2,(#35075,#35076,#35077),.UNSPECIFIED.,.F.,.F.)
B_SPLINE_CURVE_WITH_KNOTS((3,3),(-0.589144372850593,-0.536094506482411),
 .UNSPECIFIED.)
CURVE()
GEOMETRIC_REPRESENTATION_ITEM()
RATIONAL_B_SPLINE_CURVE((1.02147610369986,1.02311336089453,1.02428162962091))
REPRESENTATION_ITEM('')
);
#414=(
BOUNDED_CURVE()
B_SPLINE_CURVE(2,(#35081,#35082,#35083),.UNSPECIFIED.,.F.,.F.)
B_SPLINE_CURVE_WITH_KNOTS((3,3),(-0.271795897845351,-0.218746031477166),
 .UNSPECIFIED.)
CURVE()
GEOMETRIC_REPRESENTATION_ITEM()
RATIONAL_B_SPLINE_CURVE((1.02428162962098,1.02311336089459,1.02147610369992))
REPRESENTATION_ITEM('')
);
#415=(
BOUNDED_CURVE()
B_SPLINE_CURVE(2,(#35085,#35086,#35087),.UNSPECIFIED.,.F.,.F.)
B_SPLINE_CURVE_WITH_KNOTS((3,3),(-0.589144372850585,-0.536094506482403),
 .UNSPECIFIED.)
CURVE()
GEOMETRIC_REPRESENTATION_ITEM()
RATIONAL_B_SPLINE_CURVE((1.02147610369985,1.02311336089452,1.02428162962091))
REPRESENTATION_ITEM('')
);
#416=(
BOUNDED_CURVE()
B_SPLINE_CURVE(2,(#35091,#35092,#35093),.UNSPECIFIED.,.F.,.F.)
B_SPLINE_CURVE_WITH_KNOTS((3,3),(-0.271795897845359,-0.218746031477178),
 .UNSPECIFIED.)
CURVE()
GEOMETRIC_REPRESENTATION_ITEM()
RATIONAL_B_SPLINE_CURVE((1.02428162962089,1.02311336089451,1.02147610369984))
REPRESENTATION_ITEM('')
);
#417=(
BOUNDED_CURVE()
B_SPLINE_CURVE(2,(#35095,#35096,#35097),.UNSPECIFIED.,.F.,.F.)
B_SPLINE_CURVE_WITH_KNOTS((3,3),(-0.589144372850604,-0.536094506482418),
 .UNSPECIFIED.)
CURVE()
GEOMETRIC_REPRESENTATION_ITEM()
RATIONAL_B_SPLINE_CURVE((1.02147610369994,1.02311336089462,1.02428162962101))
REPRESENTATION_ITEM('')
);
#418=(
BOUNDED_CURVE()
B_SPLINE_CURVE(2,(#35101,#35102,#35103),.UNSPECIFIED.,.F.,.F.)
B_SPLINE_CURVE_WITH_KNOTS((3,3),(-0.271795897845358,-0.218746031477175),
 .UNSPECIFIED.)
CURVE()
GEOMETRIC_REPRESENTATION_ITEM()
RATIONAL_B_SPLINE_CURVE((1.02428162962093,1.02311336089454,1.02147610369987))
REPRESENTATION_ITEM('')
);
#419=(
BOUNDED_CURVE()
B_SPLINE_CURVE(2,(#35105,#35106,#35107),.UNSPECIFIED.,.F.,.F.)
B_SPLINE_CURVE_WITH_KNOTS((3,3),(-0.589144372850589,-0.536094506482406),
 .UNSPECIFIED.)
CURVE()
GEOMETRIC_REPRESENTATION_ITEM()
RATIONAL_B_SPLINE_CURVE((1.02147610369989,1.02311336089456,1.02428162962095))
REPRESENTATION_ITEM('')
);
#420=(
BOUNDED_CURVE()
B_SPLINE_CURVE(2,(#35111,#35112,#35113),.UNSPECIFIED.,.F.,.F.)
B_SPLINE_CURVE_WITH_KNOTS((3,3),(-0.271795897845353,-0.218746031477168),
 .UNSPECIFIED.)
CURVE()
GEOMETRIC_REPRESENTATION_ITEM()
RATIONAL_B_SPLINE_CURVE((1.02428162962098,1.0231133608946,1.02147610369992))
REPRESENTATION_ITEM('')
);
#421=(
BOUNDED_CURVE()
B_SPLINE_CURVE(2,(#35115,#35116,#35117),.UNSPECIFIED.,.F.,.F.)
B_SPLINE_CURVE_WITH_KNOTS((3,3),(-0.589144372850587,-0.536094506482403),
 .UNSPECIFIED.)
CURVE()
GEOMETRIC_REPRESENTATION_ITEM()
RATIONAL_B_SPLINE_CURVE((1.02147610369986,1.02311336089453,1.02428162962092))
REPRESENTATION_ITEM('')
);
#422=(
BOUNDED_CURVE()
B_SPLINE_CURVE(2,(#35121,#35122,#35123),.UNSPECIFIED.,.F.,.F.)
B_SPLINE_CURVE_WITH_KNOTS((3,3),(-0.271795897845348,-0.218746031477167),
 .UNSPECIFIED.)
CURVE()
GEOMETRIC_REPRESENTATION_ITEM()
RATIONAL_B_SPLINE_CURVE((1.02428162962092,1.02311336089453,1.02147610369986))
REPRESENTATION_ITEM('')
);
#423=(
BOUNDED_CURVE()
B_SPLINE_CURVE(2,(#35125,#35126,#35127),.UNSPECIFIED.,.F.,.F.)
B_SPLINE_CURVE_WITH_KNOTS((3,3),(-0.589144372850583,-0.536094506482401),
 .UNSPECIFIED.)
CURVE()
GEOMETRIC_REPRESENTATION_ITEM()
RATIONAL_B_SPLINE_CURVE((1.02147610369985,1.02311336089452,1.0242816296209))
REPRESENTATION_ITEM('')
);
#424=(
BOUNDED_CURVE()
B_SPLINE_CURVE(2,(#35131,#35132,#35133),.UNSPECIFIED.,.F.,.F.)
B_SPLINE_CURVE_WITH_KNOTS((3,3),(-0.271795897845352,-0.218746031477164),
 .UNSPECIFIED.)
CURVE()
GEOMETRIC_REPRESENTATION_ITEM()
RATIONAL_B_SPLINE_CURVE((1.02428162962106,1.02311336089466,1.02147610369999))
REPRESENTATION_ITEM('')
);
#425=(
BOUNDED_CURVE()
B_SPLINE_CURVE(2,(#35135,#35136,#35137),.UNSPECIFIED.,.F.,.F.)
B_SPLINE_CURVE_WITH_KNOTS((3,3),(-0.589144372850585,-0.536094506482407),
 .UNSPECIFIED.)
CURVE()
GEOMETRIC_REPRESENTATION_ITEM()
RATIONAL_B_SPLINE_CURVE((1.02147610369979,1.02311336089446,1.02428162962084))
REPRESENTATION_ITEM('')
);
#426=(
BOUNDED_CURVE()
B_SPLINE_CURVE(2,(#35141,#35142,#35143),.UNSPECIFIED.,.F.,.F.)
B_SPLINE_CURVE_WITH_KNOTS((3,3),(-0.271795897845344,-0.21874603147716),
 .UNSPECIFIED.)
CURVE()
GEOMETRIC_REPRESENTATION_ITEM()
RATIONAL_B_SPLINE_CURVE((1.02428162962098,1.02311336089459,1.02147610369992))
REPRESENTATION_ITEM('')
);
#427=(
BOUNDED_CURVE()
B_SPLINE_CURVE(2,(#35145,#35146,#35147),.UNSPECIFIED.,.F.,.F.)
B_SPLINE_CURVE_WITH_KNOTS((3,3),(-0.589144372850594,-0.536094506482412),
 .UNSPECIFIED.)
CURVE()
GEOMETRIC_REPRESENTATION_ITEM()
RATIONAL_B_SPLINE_CURVE((1.02147610369985,1.02311336089452,1.02428162962091))
REPRESENTATION_ITEM('')
);
#428=(
BOUNDED_CURVE()
B_SPLINE_CURVE(2,(#35151,#35152,#35153),.UNSPECIFIED.,.F.,.F.)
B_SPLINE_CURVE_WITH_KNOTS((3,3),(-0.271795897845361,-0.218746031477178),
 .UNSPECIFIED.)
CURVE()
GEOMETRIC_REPRESENTATION_ITEM()
RATIONAL_B_SPLINE_CURVE((1.02428162962094,1.02311336089455,1.02147610369988))
REPRESENTATION_ITEM('')
);
#429=(
BOUNDED_CURVE()
B_SPLINE_CURVE(2,(#35155,#35156,#35157),.UNSPECIFIED.,.F.,.F.)
B_SPLINE_CURVE_WITH_KNOTS((3,3),(-0.589144372850589,-0.536094506482408),
 .UNSPECIFIED.)
CURVE()
GEOMETRIC_REPRESENTATION_ITEM()
RATIONAL_B_SPLINE_CURVE((1.02147610369984,1.02311336089451,1.02428162962089))
REPRESENTATION_ITEM('')
);
#430=(
BOUNDED_CURVE()
B_SPLINE_CURVE(2,(#35161,#35162,#35163),.UNSPECIFIED.,.F.,.F.)
B_SPLINE_CURVE_WITH_KNOTS((3,3),(-0.271795897845358,-0.218746031477168),
 .UNSPECIFIED.)
CURVE()
GEOMETRIC_REPRESENTATION_ITEM()
RATIONAL_B_SPLINE_CURVE((1.0242816296211,1.02311336089471,1.02147610370002))
REPRESENTATION_ITEM('')
);
#431=(
BOUNDED_CURVE()
B_SPLINE_CURVE(2,(#35165,#35166,#35167),.UNSPECIFIED.,.F.,.F.)
B_SPLINE_CURVE_WITH_KNOTS((3,3),(-0.5891443728506,-0.536094506482411),
 .UNSPECIFIED.)
CURVE()
GEOMETRIC_REPRESENTATION_ITEM()
RATIONAL_B_SPLINE_CURVE((1.02147610369999,1.02311336089467,1.02428162962106))
REPRESENTATION_ITEM('')
);
#432=(
BOUNDED_CURVE()
B_SPLINE_CURVE(2,(#35171,#35172,#35173),.UNSPECIFIED.,.F.,.F.)
B_SPLINE_CURVE_WITH_KNOTS((3,3),(-0.271795897845357,-0.218746031477171),
 .UNSPECIFIED.)
CURVE()
GEOMETRIC_REPRESENTATION_ITEM()
RATIONAL_B_SPLINE_CURVE((1.02428162962099,1.0231133608946,1.02147610369993))
REPRESENTATION_ITEM('')
);
#433=(
BOUNDED_CURVE()
B_SPLINE_CURVE(2,(#35175,#35176,#35177),.UNSPECIFIED.,.F.,.F.)
B_SPLINE_CURVE_WITH_KNOTS((3,3),(-0.589144372850592,-0.536094506482407),
 .UNSPECIFIED.)
CURVE()
GEOMETRIC_REPRESENTATION_ITEM()
RATIONAL_B_SPLINE_CURVE((1.02147610369992,1.0231133608946,1.02428162962099))
REPRESENTATION_ITEM('')
);
#434=(
BOUNDED_CURVE()
B_SPLINE_CURVE(2,(#35181,#35182,#35183),.UNSPECIFIED.,.F.,.F.)
B_SPLINE_CURVE_WITH_KNOTS((3,3),(-0.27179589784535,-0.218746031477161),
 .UNSPECIFIED.)
CURVE()
GEOMETRIC_REPRESENTATION_ITEM()
RATIONAL_B_SPLINE_CURVE((1.02428162962108,1.02311336089469,1.02147610370001))
REPRESENTATION_ITEM('')
);
#435=(
BOUNDED_CURVE()
B_SPLINE_CURVE(2,(#35185,#35186,#35187),.UNSPECIFIED.,.F.,.F.)
B_SPLINE_CURVE_WITH_KNOTS((3,3),(-0.589144372850596,-0.536094506482411),
 .UNSPECIFIED.)
CURVE()
GEOMETRIC_REPRESENTATION_ITEM()
RATIONAL_B_SPLINE_CURVE((1.02147610369991,1.02311336089458,1.02428162962097))
REPRESENTATION_ITEM('')
);
#436=(
BOUNDED_CURVE()
B_SPLINE_CURVE(2,(#35191,#35192,#35193),.UNSPECIFIED.,.F.,.F.)
B_SPLINE_CURVE_WITH_KNOTS((3,3),(-0.271795897845359,-0.218746031477175),
 .UNSPECIFIED.)
CURVE()
GEOMETRIC_REPRESENTATION_ITEM()
RATIONAL_B_SPLINE_CURVE((1.02428162962097,1.02311336089458,1.02147610369991))
REPRESENTATION_ITEM('')
);
#437=(
BOUNDED_CURVE()
B_SPLINE_CURVE(2,(#35195,#35196,#35197),.UNSPECIFIED.,.F.,.F.)
B_SPLINE_CURVE_WITH_KNOTS((3,3),(-0.589144372850594,-0.536094506482411),
 .UNSPECIFIED.)
CURVE()
GEOMETRIC_REPRESENTATION_ITEM()
RATIONAL_B_SPLINE_CURVE((1.02147610369989,1.02311336089456,1.02428162962095))
REPRESENTATION_ITEM('')
);
#438=(
BOUNDED_CURVE()
B_SPLINE_CURVE(2,(#35201,#35202,#35203),.UNSPECIFIED.,.F.,.F.)
B_SPLINE_CURVE_WITH_KNOTS((3,3),(-0.271795897845358,-0.218746031477177),
 .UNSPECIFIED.)
CURVE()
GEOMETRIC_REPRESENTATION_ITEM()
RATIONAL_B_SPLINE_CURVE((1.02428162962088,1.0231133608945,1.02147610369983))
REPRESENTATION_ITEM('')
);
#439=(
BOUNDED_CURVE()
B_SPLINE_CURVE(2,(#35205,#35206,#35207),.UNSPECIFIED.,.F.,.F.)
B_SPLINE_CURVE_WITH_KNOTS((3,3),(-0.589144372850591,-0.536094506482403),
 .UNSPECIFIED.)
CURVE()
GEOMETRIC_REPRESENTATION_ITEM()
RATIONAL_B_SPLINE_CURVE((1.02147610369996,1.02311336089463,1.02428162962103))
REPRESENTATION_ITEM('')
);
#440=(
BOUNDED_CURVE()
B_SPLINE_CURVE(2,(#35211,#35212,#35213),.UNSPECIFIED.,.F.,.F.)
B_SPLINE_CURVE_WITH_KNOTS((3,3),(-0.271795897845352,-0.218746031477168),
 .UNSPECIFIED.)
CURVE()
GEOMETRIC_REPRESENTATION_ITEM()
RATIONAL_B_SPLINE_CURVE((1.02428162962098,1.02311336089459,1.02147610369992))
REPRESENTATION_ITEM('')
);
#441=(
BOUNDED_CURVE()
B_SPLINE_CURVE(2,(#35215,#35216,#35217),.UNSPECIFIED.,.F.,.F.)
B_SPLINE_CURVE_WITH_KNOTS((3,3),(-0.589144372850591,-0.536094506482408),
 .UNSPECIFIED.)
CURVE()
GEOMETRIC_REPRESENTATION_ITEM()
RATIONAL_B_SPLINE_CURVE((1.02147610369988,1.02311336089455,1.02428162962094))
REPRESENTATION_ITEM('')
);
#442=(
BOUNDED_CURVE()
B_SPLINE_CURVE(2,(#35221,#35222,#35223),.UNSPECIFIED.,.F.,.F.)
B_SPLINE_CURVE_WITH_KNOTS((3,3),(-0.271795897845345,-0.21874603147716),
 .UNSPECIFIED.)
CURVE()
GEOMETRIC_REPRESENTATION_ITEM()
RATIONAL_B_SPLINE_CURVE((1.024281629621,1.02311336089461,1.02147610369993))
REPRESENTATION_ITEM('')
);
#443=(
BOUNDED_CURVE()
B_SPLINE_CURVE(2,(#35225,#35226,#35227),.UNSPECIFIED.,.F.,.F.)
B_SPLINE_CURVE_WITH_KNOTS((3,3),(-0.589144372850594,-0.536094506482409),
 .UNSPECIFIED.)
CURVE()
GEOMETRIC_REPRESENTATION_ITEM()
RATIONAL_B_SPLINE_CURVE((1.02147610369992,1.02311336089459,1.02428162962098))
REPRESENTATION_ITEM('')
);
#444=(
BOUNDED_CURVE()
B_SPLINE_CURVE(2,(#35231,#35232,#35233),.UNSPECIFIED.,.F.,.F.)
B_SPLINE_CURVE_WITH_KNOTS((3,3),(-0.271795897845346,-0.218746031477163),
 .UNSPECIFIED.)
CURVE()
GEOMETRIC_REPRESENTATION_ITEM()
RATIONAL_B_SPLINE_CURVE((1.02428162962097,1.02311336089458,1.02147610369991))
REPRESENTATION_ITEM('')
);
#445=(
BOUNDED_CURVE()
B_SPLINE_CURVE(2,(#35235,#35236,#35237),.UNSPECIFIED.,.F.,.F.)
B_SPLINE_CURVE_WITH_KNOTS((3,3),(-0.589144372850596,-0.536094506482413),
 .UNSPECIFIED.)
CURVE()
GEOMETRIC_REPRESENTATION_ITEM()
RATIONAL_B_SPLINE_CURVE((1.02147610369989,1.02311336089456,1.02428162962095))
REPRESENTATION_ITEM('')
);
#446=(
BOUNDED_CURVE()
B_SPLINE_CURVE(2,(#35241,#35242,#35243),.UNSPECIFIED.,.F.,.F.)
B_SPLINE_CURVE_WITH_KNOTS((3,3),(-0.271795897845354,-0.218746031477172),
 .UNSPECIFIED.)
CURVE()
GEOMETRIC_REPRESENTATION_ITEM()
RATIONAL_B_SPLINE_CURVE((1.02428162962092,1.02311336089453,1.02147610369987))
REPRESENTATION_ITEM('')
);
#447=(
BOUNDED_CURVE()
B_SPLINE_CURVE(2,(#35245,#35246,#35247),.UNSPECIFIED.,.F.,.F.)
B_SPLINE_CURVE_WITH_KNOTS((3,3),(-0.589144372850593,-0.53609450648241),
 .UNSPECIFIED.)
CURVE()
GEOMETRIC_REPRESENTATION_ITEM()
RATIONAL_B_SPLINE_CURVE((1.02147610369989,1.02311336089456,1.02428162962095))
REPRESENTATION_ITEM('')
);
#448=(
BOUNDED_CURVE()
B_SPLINE_CURVE(2,(#35251,#35252,#35253),.UNSPECIFIED.,.F.,.F.)
B_SPLINE_CURVE_WITH_KNOTS((3,3),(-0.271795897845358,-0.218746031477176),
 .UNSPECIFIED.)
CURVE()
GEOMETRIC_REPRESENTATION_ITEM()
RATIONAL_B_SPLINE_CURVE((1.02428162962091,1.02311336089452,1.02147610369985))
REPRESENTATION_ITEM('')
);
#449=(
BOUNDED_CURVE()
B_SPLINE_CURVE(2,(#35255,#35256,#35257),.UNSPECIFIED.,.F.,.F.)
B_SPLINE_CURVE_WITH_KNOTS((3,3),(-0.589144372850596,-0.536094506482412),
 .UNSPECIFIED.)
CURVE()
GEOMETRIC_REPRESENTATION_ITEM()
RATIONAL_B_SPLINE_CURVE((1.02147610369988,1.02311336089455,1.02428162962094))
REPRESENTATION_ITEM('')
);
#450=(
BOUNDED_CURVE()
B_SPLINE_CURVE(2,(#35261,#35262,#35263),.UNSPECIFIED.,.F.,.F.)
B_SPLINE_CURVE_WITH_KNOTS((3,3),(-0.271795897845353,-0.218746031477168),
 .UNSPECIFIED.)
CURVE()
GEOMETRIC_REPRESENTATION_ITEM()
RATIONAL_B_SPLINE_CURVE((1.024281629621,1.02311336089461,1.02147610369994))
REPRESENTATION_ITEM('')
);
#451=(
BOUNDED_CURVE()
B_SPLINE_CURVE(2,(#35265,#35266,#35267),.UNSPECIFIED.,.F.,.F.)
B_SPLINE_CURVE_WITH_KNOTS((3,3),(-0.589144372850586,-0.536094506482402),
 .UNSPECIFIED.)
CURVE()
GEOMETRIC_REPRESENTATION_ITEM()
RATIONAL_B_SPLINE_CURVE((1.02147610369992,1.02311336089459,1.02428162962098))
REPRESENTATION_ITEM('')
);
#452=(
BOUNDED_CURVE()
B_SPLINE_CURVE(2,(#35271,#35272,#35273),.UNSPECIFIED.,.F.,.F.)
B_SPLINE_CURVE_WITH_KNOTS((3,3),(-0.271795897845356,-0.218746031477171),
 .UNSPECIFIED.)
CURVE()
GEOMETRIC_REPRESENTATION_ITEM()
RATIONAL_B_SPLINE_CURVE((1.02428162962097,1.02311336089458,1.0214761036999))
REPRESENTATION_ITEM('')
);
#453=(
BOUNDED_CURVE()
B_SPLINE_CURVE(2,(#35275,#35276,#35277),.UNSPECIFIED.,.F.,.F.)
B_SPLINE_CURVE_WITH_KNOTS((3,3),(-0.589144372850589,-0.536094506482406),
 .UNSPECIFIED.)
CURVE()
GEOMETRIC_REPRESENTATION_ITEM()
RATIONAL_B_SPLINE_CURVE((1.02147610369989,1.02311336089456,1.02428162962095))
REPRESENTATION_ITEM('')
);
#454=(
BOUNDED_CURVE()
B_SPLINE_CURVE(2,(#35281,#35282,#35283),.UNSPECIFIED.,.F.,.F.)
B_SPLINE_CURVE_WITH_KNOTS((3,3),(-0.271795897845358,-0.218746031477175),
 .UNSPECIFIED.)
CURVE()
GEOMETRIC_REPRESENTATION_ITEM()
RATIONAL_B_SPLINE_CURVE((1.02428162962095,1.02311336089456,1.02147610369989))
REPRESENTATION_ITEM('')
);
#455=(
BOUNDED_CURVE()
B_SPLINE_CURVE(2,(#35285,#35286,#35287),.UNSPECIFIED.,.F.,.F.)
B_SPLINE_CURVE_WITH_KNOTS((3,3),(-0.589144372850611,-0.536094506482426),
 .UNSPECIFIED.)
CURVE()
GEOMETRIC_REPRESENTATION_ITEM()
RATIONAL_B_SPLINE_CURVE((1.02147610369994,1.02311336089462,1.02428162962101))
REPRESENTATION_ITEM('')
);
#456=(
BOUNDED_CURVE()
B_SPLINE_CURVE(2,(#35291,#35292,#35293),.UNSPECIFIED.,.F.,.F.)
B_SPLINE_CURVE_WITH_KNOTS((3,3),(-0.271795897845356,-0.218746031477171),
 .UNSPECIFIED.)
CURVE()
GEOMETRIC_REPRESENTATION_ITEM()
RATIONAL_B_SPLINE_CURVE((1.02428162962099,1.0231133608946,1.02147610369993))
REPRESENTATION_ITEM('')
);
#457=(
BOUNDED_CURVE()
B_SPLINE_CURVE(2,(#35295,#35296,#35297),.UNSPECIFIED.,.F.,.F.)
B_SPLINE_CURVE_WITH_KNOTS((3,3),(-0.589144372850582,-0.536094506482403),
 .UNSPECIFIED.)
CURVE()
GEOMETRIC_REPRESENTATION_ITEM()
RATIONAL_B_SPLINE_CURVE((1.02147610369981,1.02311336089448,1.02428162962086))
REPRESENTATION_ITEM('')
);
#458=(
BOUNDED_CURVE()
B_SPLINE_CURVE(2,(#35301,#35302,#35303),.UNSPECIFIED.,.F.,.F.)
B_SPLINE_CURVE_WITH_KNOTS((3,3),(-0.271795897845348,-0.218746031477162),
 .UNSPECIFIED.)
CURVE()
GEOMETRIC_REPRESENTATION_ITEM()
RATIONAL_B_SPLINE_CURVE((1.02428162962101,1.02311336089462,1.02147610369994))
REPRESENTATION_ITEM('')
);
#459=(
BOUNDED_CURVE()
B_SPLINE_CURVE(2,(#35305,#35306,#35307),.UNSPECIFIED.,.F.,.F.)
B_SPLINE_CURVE_WITH_KNOTS((3,3),(-0.589144372850586,-0.536094506482406),
 .UNSPECIFIED.)
CURVE()
GEOMETRIC_REPRESENTATION_ITEM()
RATIONAL_B_SPLINE_CURVE((1.02147610369985,1.02311336089452,1.02428162962091))
REPRESENTATION_ITEM('')
);
#460=(
BOUNDED_CURVE()
B_SPLINE_CURVE(2,(#35311,#35312,#35313),.UNSPECIFIED.,.F.,.F.)
B_SPLINE_CURVE_WITH_KNOTS((3,3),(-0.271795897845348,-0.218746031477166),
 .UNSPECIFIED.)
CURVE()
GEOMETRIC_REPRESENTATION_ITEM()
RATIONAL_B_SPLINE_CURVE((1.02428162962094,1.02311336089455,1.02147610369988))
REPRESENTATION_ITEM('')
);
#461=(
BOUNDED_CURVE()
B_SPLINE_CURVE(2,(#35315,#35316,#35317),.UNSPECIFIED.,.F.,.F.)
B_SPLINE_CURVE_WITH_KNOTS((3,3),(-0.589144372850589,-0.536094506482402),
 .UNSPECIFIED.)
CURVE()
GEOMETRIC_REPRESENTATION_ITEM()
RATIONAL_B_SPLINE_CURVE((1.02147610369993,1.0231133608946,1.02428162962099))
REPRESENTATION_ITEM('')
);
#462=(
BOUNDED_CURVE()
B_SPLINE_CURVE(2,(#35321,#35322,#35323),.UNSPECIFIED.,.F.,.F.)
B_SPLINE_CURVE_WITH_KNOTS((3,3),(-0.271795897845359,-0.218746031477172),
 .UNSPECIFIED.)
CURVE()
GEOMETRIC_REPRESENTATION_ITEM()
RATIONAL_B_SPLINE_CURVE((1.02428162962103,1.02311336089464,1.02147610369996))
REPRESENTATION_ITEM('')
);
#463=(
BOUNDED_CURVE()
B_SPLINE_CURVE(2,(#35325,#35326,#35327),.UNSPECIFIED.,.F.,.F.)
B_SPLINE_CURVE_WITH_KNOTS((3,3),(-0.589144372850584,-0.536094506482398),
 .UNSPECIFIED.)
CURVE()
GEOMETRIC_REPRESENTATION_ITEM()
RATIONAL_B_SPLINE_CURVE((1.02147610369995,1.02311336089463,1.02428162962102))
REPRESENTATION_ITEM('')
);
#464=(
BOUNDED_CURVE()
B_SPLINE_CURVE(2,(#35331,#35332,#35333),.UNSPECIFIED.,.F.,.F.)
B_SPLINE_CURVE_WITH_KNOTS((3,3),(-0.271795897845344,-0.218746031477162),
 .UNSPECIFIED.)
CURVE()
GEOMETRIC_REPRESENTATION_ITEM()
RATIONAL_B_SPLINE_CURVE((1.02428162962092,1.02311336089454,1.02147610369987))
REPRESENTATION_ITEM('')
);
#465=(
BOUNDED_CURVE()
B_SPLINE_CURVE(2,(#35335,#35336,#35337),.UNSPECIFIED.,.F.,.F.)
B_SPLINE_CURVE_WITH_KNOTS((3,3),(-0.589144372850587,-0.536094506482403),
 .UNSPECIFIED.)
CURVE()
GEOMETRIC_REPRESENTATION_ITEM()
RATIONAL_B_SPLINE_CURVE((1.0214761036999,1.02311336089457,1.02428162962096))
REPRESENTATION_ITEM('')
);
#466=(
BOUNDED_CURVE()
B_SPLINE_CURVE(2,(#35341,#35342,#35343),.UNSPECIFIED.,.F.,.F.)
B_SPLINE_CURVE_WITH_KNOTS((3,3),(-0.27179589784536,-0.218746031477177),
 .UNSPECIFIED.)
CURVE()
GEOMETRIC_REPRESENTATION_ITEM()
RATIONAL_B_SPLINE_CURVE((1.02428162962093,1.02311336089455,1.02147610369988))
REPRESENTATION_ITEM('')
);
#467=(
BOUNDED_CURVE()
B_SPLINE_CURVE(2,(#35345,#35346,#35347),.UNSPECIFIED.,.F.,.F.)
B_SPLINE_CURVE_WITH_KNOTS((3,3),(-0.589144372850582,-0.536094506482399),
 .UNSPECIFIED.)
CURVE()
GEOMETRIC_REPRESENTATION_ITEM()
RATIONAL_B_SPLINE_CURVE((1.02147610369987,1.02311336089454,1.02428162962092))
REPRESENTATION_ITEM('')
);
#468=(
BOUNDED_CURVE()
B_SPLINE_CURVE(2,(#35351,#35352,#35353),.UNSPECIFIED.,.F.,.F.)
B_SPLINE_CURVE_WITH_KNOTS((3,3),(-0.27179589784536,-0.21874603147718),
 .UNSPECIFIED.)
CURVE()
GEOMETRIC_REPRESENTATION_ITEM()
RATIONAL_B_SPLINE_CURVE((1.02428162962089,1.0231133608945,1.02147610369983))
REPRESENTATION_ITEM('')
);
#469=(
BOUNDED_CURVE()
B_SPLINE_CURVE(2,(#35355,#35356,#35357),.UNSPECIFIED.,.F.,.F.)
B_SPLINE_CURVE_WITH_KNOTS((3,3),(-0.589144372850591,-0.536094506482404),
 .UNSPECIFIED.)
CURVE()
GEOMETRIC_REPRESENTATION_ITEM()
RATIONAL_B_SPLINE_CURVE((1.02147610369995,1.02311336089462,1.02428162962101))
REPRESENTATION_ITEM('')
);
#470=(
BOUNDED_CURVE()
B_SPLINE_CURVE(2,(#35361,#35362,#35363),.UNSPECIFIED.,.F.,.F.)
B_SPLINE_CURVE_WITH_KNOTS((3,3),(-0.271795897845354,-0.21874603147717),
 .UNSPECIFIED.)
CURVE()
GEOMETRIC_REPRESENTATION_ITEM()
RATIONAL_B_SPLINE_CURVE((1.02428162962096,1.02311336089457,1.0214761036999))
REPRESENTATION_ITEM('')
);
#471=(
BOUNDED_CURVE()
B_SPLINE_CURVE(2,(#35365,#35366,#35367),.UNSPECIFIED.,.F.,.F.)
B_SPLINE_CURVE_WITH_KNOTS((3,3),(-0.58914437285059,-0.536094506482403),
 .UNSPECIFIED.)
CURVE()
GEOMETRIC_REPRESENTATION_ITEM()
RATIONAL_B_SPLINE_CURVE((1.02147610369995,1.02311336089463,1.02428162962102))
REPRESENTATION_ITEM('')
);
#472=(
BOUNDED_CURVE()
B_SPLINE_CURVE(2,(#35371,#35372,#35373),.UNSPECIFIED.,.F.,.F.)
B_SPLINE_CURVE_WITH_KNOTS((3,3),(-0.271795897845357,-0.218746031477171),
 .UNSPECIFIED.)
CURVE()
GEOMETRIC_REPRESENTATION_ITEM()
RATIONAL_B_SPLINE_CURVE((1.024281629621,1.02311336089461,1.02147610369993))
REPRESENTATION_ITEM('')
);
#473=(
BOUNDED_CURVE()
B_SPLINE_CURVE(2,(#35375,#35376,#35377),.UNSPECIFIED.,.F.,.F.)
B_SPLINE_CURVE_WITH_KNOTS((3,3),(-0.589144372850596,-0.536094506482413),
 .UNSPECIFIED.)
CURVE()
GEOMETRIC_REPRESENTATION_ITEM()
RATIONAL_B_SPLINE_CURVE((1.02147610369988,1.02311336089455,1.02428162962094))
REPRESENTATION_ITEM('')
);
#474=(
BOUNDED_CURVE()
B_SPLINE_CURVE(2,(#35381,#35382,#35383),.UNSPECIFIED.,.F.,.F.)
B_SPLINE_CURVE_WITH_KNOTS((3,3),(-0.27179589784535,-0.270098893534619),
 .UNSPECIFIED.)
CURVE()
GEOMETRIC_REPRESENTATION_ITEM()
RATIONAL_B_SPLINE_CURVE((1.02428162962103,1.02424425804593,1.02420640656121))
REPRESENTATION_ITEM('')
);
#475=(
BOUNDED_CURVE()
B_SPLINE_CURVE(2,(#35388,#35389,#35390),.UNSPECIFIED.,.F.,.F.)
B_SPLINE_CURVE_WITH_KNOTS((3,3),(-0.270098893534619,-0.218746031477162),
 .UNSPECIFIED.)
CURVE()
GEOMETRIC_REPRESENTATION_ITEM()
RATIONAL_B_SPLINE_CURVE((1.02420640656121,1.02306098691696,1.02147610369996))
REPRESENTATION_ITEM('')
);
#476=(
BOUNDED_CURVE()
B_SPLINE_CURVE(2,(#35392,#35393,#35394),.UNSPECIFIED.,.F.,.F.)
B_SPLINE_CURVE_WITH_KNOTS((3,3),(-0.589144372850598,-0.536094506482416),
 .UNSPECIFIED.)
CURVE()
GEOMETRIC_REPRESENTATION_ITEM()
RATIONAL_B_SPLINE_CURVE((1.02147610369987,1.02311336089454,1.02428162962093))
REPRESENTATION_ITEM('')
);
#477=(
BOUNDED_CURVE()
B_SPLINE_CURVE(2,(#35398,#35399,#35400),.UNSPECIFIED.,.F.,.F.)
B_SPLINE_CURVE_WITH_KNOTS((3,3),(-0.271795897845349,-0.218746031477166),
 .UNSPECIFIED.)
CURVE()
GEOMETRIC_REPRESENTATION_ITEM()
RATIONAL_B_SPLINE_CURVE((1.02428162962097,1.02311336089458,1.02147610369991))
REPRESENTATION_ITEM('')
);
#478=(
BOUNDED_CURVE()
B_SPLINE_CURVE(2,(#35402,#35403,#35404),.UNSPECIFIED.,.F.,.F.)
B_SPLINE_CURVE_WITH_KNOTS((3,3),(-0.589144372850578,-0.536094506482394),
 .UNSPECIFIED.)
CURVE()
GEOMETRIC_REPRESENTATION_ITEM()
RATIONAL_B_SPLINE_CURVE((1.02147610369988,1.02311336089455,1.02428162962093))
REPRESENTATION_ITEM('')
);
#479=(
BOUNDED_CURVE()
B_SPLINE_CURVE(2,(#35408,#35409,#35410),.UNSPECIFIED.,.F.,.F.)
B_SPLINE_CURVE_WITH_KNOTS((3,3),(-0.27179589784536,-0.218746031477173),
 .UNSPECIFIED.)
CURVE()
GEOMETRIC_REPRESENTATION_ITEM()
RATIONAL_B_SPLINE_CURVE((1.024281629621,1.02311336089461,1.02147610369993))
REPRESENTATION_ITEM('')
);
#480=(
BOUNDED_CURVE()
B_SPLINE_CURVE(2,(#35412,#35413,#35414),.UNSPECIFIED.,.F.,.F.)
B_SPLINE_CURVE_WITH_KNOTS((3,3),(-0.589144372850572,-0.536094506482391),
 .UNSPECIFIED.)
CURVE()
GEOMETRIC_REPRESENTATION_ITEM()
RATIONAL_B_SPLINE_CURVE((1.02147610369982,1.02311336089448,1.02428162962086))
REPRESENTATION_ITEM('')
);
#481=(
BOUNDED_CURVE()
B_SPLINE_CURVE(2,(#35418,#35419,#35420),.UNSPECIFIED.,.F.,.F.)
B_SPLINE_CURVE_WITH_KNOTS((3,3),(-0.271795897845356,-0.21874603147717),
 .UNSPECIFIED.)
CURVE()
GEOMETRIC_REPRESENTATION_ITEM()
RATIONAL_B_SPLINE_CURVE((1.02428162962099,1.0231133608946,1.02147610369993))
REPRESENTATION_ITEM('')
);
#482=(
BOUNDED_CURVE()
B_SPLINE_CURVE(2,(#35422,#35423,#35424),.UNSPECIFIED.,.F.,.F.)
B_SPLINE_CURVE_WITH_KNOTS((3,3),(-0.589144372850566,-0.536094506482389),
 .UNSPECIFIED.)
CURVE()
GEOMETRIC_REPRESENTATION_ITEM()
RATIONAL_B_SPLINE_CURVE((1.02147610369972,1.02311336089438,1.02428162962076))
REPRESENTATION_ITEM('')
);
#483=(
BOUNDED_CURVE()
B_SPLINE_CURVE(2,(#35428,#35429,#35430),.UNSPECIFIED.,.F.,.F.)
B_SPLINE_CURVE_WITH_KNOTS((3,3),(-0.271795897845343,-0.218746031477157),
 .UNSPECIFIED.)
CURVE()
GEOMETRIC_REPRESENTATION_ITEM()
RATIONAL_B_SPLINE_CURVE((1.02428162962101,1.02311336089462,1.02147610369994))
REPRESENTATION_ITEM('')
);
#484=(
BOUNDED_CURVE()
B_SPLINE_CURVE(2,(#35432,#35433,#35434),.UNSPECIFIED.,.F.,.F.)
B_SPLINE_CURVE_WITH_KNOTS((3,3),(-0.589144372850584,-0.536094506482395),
 .UNSPECIFIED.)
CURVE()
GEOMETRIC_REPRESENTATION_ITEM()
RATIONAL_B_SPLINE_CURVE((1.02147610369997,1.02311336089465,1.02428162962104))
REPRESENTATION_ITEM('')
);
#485=(
BOUNDED_CURVE()
B_SPLINE_CURVE(2,(#35438,#35439,#35440),.UNSPECIFIED.,.F.,.F.)
B_SPLINE_CURVE_WITH_KNOTS((3,3),(-0.27179589784534,-0.218746031477154),
 .UNSPECIFIED.)
CURVE()
GEOMETRIC_REPRESENTATION_ITEM()
RATIONAL_B_SPLINE_CURVE((1.02428162962103,1.02311336089464,1.02147610369996))
REPRESENTATION_ITEM('')
);
#486=(
BOUNDED_CURVE()
B_SPLINE_CURVE(2,(#35442,#35443,#35444),.UNSPECIFIED.,.F.,.F.)
B_SPLINE_CURVE_WITH_KNOTS((3,3),(-0.589144372850587,-0.536094506482399),
 .UNSPECIFIED.)
CURVE()
GEOMETRIC_REPRESENTATION_ITEM()
RATIONAL_B_SPLINE_CURVE((1.02147610369995,1.02311336089463,1.02428162962102))
REPRESENTATION_ITEM('')
);
#487=(
BOUNDED_CURVE()
B_SPLINE_CURVE(2,(#35448,#35449,#35450),.UNSPECIFIED.,.F.,.F.)
B_SPLINE_CURVE_WITH_KNOTS((3,3),(-0.271795897845355,-0.218746031477173),
 .UNSPECIFIED.)
CURVE()
GEOMETRIC_REPRESENTATION_ITEM()
RATIONAL_B_SPLINE_CURVE((1.02428162962092,1.02311336089454,1.02147610369987))
REPRESENTATION_ITEM('')
);
#488=(
BOUNDED_CURVE()
B_SPLINE_CURVE(2,(#35452,#35453,#35454),.UNSPECIFIED.,.F.,.F.)
B_SPLINE_CURVE_WITH_KNOTS((3,3),(-0.58914437285059,-0.536094506482405),
 .UNSPECIFIED.)
CURVE()
GEOMETRIC_REPRESENTATION_ITEM()
RATIONAL_B_SPLINE_CURVE((1.02147610369994,1.02311336089462,1.02428162962101))
REPRESENTATION_ITEM('')
);
#489=(
BOUNDED_CURVE()
B_SPLINE_CURVE(2,(#35458,#35459,#35460),.UNSPECIFIED.,.F.,.F.)
B_SPLINE_CURVE_WITH_KNOTS((3,3),(-0.271795897845348,-0.218746031477163),
 .UNSPECIFIED.)
CURVE()
GEOMETRIC_REPRESENTATION_ITEM()
RATIONAL_B_SPLINE_CURVE((1.02428162962098,1.02311336089459,1.02147610369992))
REPRESENTATION_ITEM('')
);
#490=(
BOUNDED_CURVE()
B_SPLINE_CURVE(2,(#35462,#35463,#35464),.UNSPECIFIED.,.F.,.F.)
B_SPLINE_CURVE_WITH_KNOTS((3,3),(-0.589144372850584,-0.536094506482403),
 .UNSPECIFIED.)
CURVE()
GEOMETRIC_REPRESENTATION_ITEM()
RATIONAL_B_SPLINE_CURVE((1.02147610369983,1.0231133608945,1.02428162962088))
REPRESENTATION_ITEM('')
);
#491=(
BOUNDED_CURVE()
B_SPLINE_CURVE(2,(#35468,#35469,#35470),.UNSPECIFIED.,.F.,.F.)
B_SPLINE_CURVE_WITH_KNOTS((3,3),(-0.27179589784536,-0.218746031477177),
 .UNSPECIFIED.)
CURVE()
GEOMETRIC_REPRESENTATION_ITEM()
RATIONAL_B_SPLINE_CURVE((1.02428162962094,1.02311336089455,1.02147610369988))
REPRESENTATION_ITEM('')
);
#492=(
BOUNDED_CURVE()
B_SPLINE_CURVE(2,(#35472,#35473,#35474),.UNSPECIFIED.,.F.,.F.)
B_SPLINE_CURVE_WITH_KNOTS((3,3),(-0.589144372850591,-0.536094506482406),
 .UNSPECIFIED.)
CURVE()
GEOMETRIC_REPRESENTATION_ITEM()
RATIONAL_B_SPLINE_CURVE((1.02147610369995,1.02311336089463,1.02428162962102))
REPRESENTATION_ITEM('')
);
#493=(
BOUNDED_CURVE()
B_SPLINE_CURVE(2,(#35478,#35479,#35480),.UNSPECIFIED.,.F.,.F.)
B_SPLINE_CURVE_WITH_KNOTS((3,3),(-0.271795897845357,-0.218746031477177),
 .UNSPECIFIED.)
CURVE()
GEOMETRIC_REPRESENTATION_ITEM()
RATIONAL_B_SPLINE_CURVE((1.02428162962087,1.02311336089449,1.02147610369982))
REPRESENTATION_ITEM('')
);
#494=(
BOUNDED_CURVE()
B_SPLINE_CURVE(2,(#35482,#35483,#35484),.UNSPECIFIED.,.F.,.F.)
B_SPLINE_CURVE_WITH_KNOTS((3,3),(-0.589144372850584,-0.536094506482401),
 .UNSPECIFIED.)
CURVE()
GEOMETRIC_REPRESENTATION_ITEM()
RATIONAL_B_SPLINE_CURVE((1.02147610369986,1.02311336089452,1.02428162962091))
REPRESENTATION_ITEM('')
);
#495=(
BOUNDED_CURVE()
B_SPLINE_CURVE(2,(#35488,#35489,#35490),.UNSPECIFIED.,.F.,.F.)
B_SPLINE_CURVE_WITH_KNOTS((3,3),(-0.27179589784536,-0.21874603147717),
 .UNSPECIFIED.)
CURVE()
GEOMETRIC_REPRESENTATION_ITEM()
RATIONAL_B_SPLINE_CURVE((1.02428162962108,1.02311336089468,1.0214761037))
REPRESENTATION_ITEM('')
);
#496=(
BOUNDED_CURVE()
B_SPLINE_CURVE(2,(#35492,#35493,#35494),.UNSPECIFIED.,.F.,.F.)
B_SPLINE_CURVE_WITH_KNOTS((3,3),(-0.589144372850587,-0.536094506482401),
 .UNSPECIFIED.)
CURVE()
GEOMETRIC_REPRESENTATION_ITEM()
RATIONAL_B_SPLINE_CURVE((1.02147610369992,1.02311336089459,1.02428162962098))
REPRESENTATION_ITEM('')
);
#497=(
BOUNDED_CURVE()
B_SPLINE_CURVE(2,(#35498,#35499,#35500),.UNSPECIFIED.,.F.,.F.)
B_SPLINE_CURVE_WITH_KNOTS((3,3),(-0.271795897845351,-0.218746031477167),
 .UNSPECIFIED.)
CURVE()
GEOMETRIC_REPRESENTATION_ITEM()
RATIONAL_B_SPLINE_CURVE((1.02428162962096,1.02311336089457,1.0214761036999))
REPRESENTATION_ITEM('')
);
#498=(
BOUNDED_CURVE()
B_SPLINE_CURVE(2,(#35502,#35503,#35504),.UNSPECIFIED.,.F.,.F.)
B_SPLINE_CURVE_WITH_KNOTS((3,3),(-0.589144372850593,-0.53609450648241),
 .UNSPECIFIED.)
CURVE()
GEOMETRIC_REPRESENTATION_ITEM()
RATIONAL_B_SPLINE_CURVE((1.02147610369987,1.02311336089454,1.02428162962093))
REPRESENTATION_ITEM('')
);
#499=(
BOUNDED_CURVE()
B_SPLINE_CURVE(2,(#35508,#35509,#35510),.UNSPECIFIED.,.F.,.F.)
B_SPLINE_CURVE_WITH_KNOTS((3,3),(-0.271795897845359,-0.218746031477174),
 .UNSPECIFIED.)
CURVE()
GEOMETRIC_REPRESENTATION_ITEM()
RATIONAL_B_SPLINE_CURVE((1.02428162962098,1.02311336089459,1.02147610369992))
REPRESENTATION_ITEM('')
);
#500=(
BOUNDED_CURVE()
B_SPLINE_CURVE(2,(#35512,#35513,#35514),.UNSPECIFIED.,.F.,.F.)
B_SPLINE_CURVE_WITH_KNOTS((3,3),(-0.589144372850586,-0.536094506482401),
 .UNSPECIFIED.)
CURVE()
GEOMETRIC_REPRESENTATION_ITEM()
RATIONAL_B_SPLINE_CURVE((1.02147610369989,1.02311336089456,1.02428162962095))
REPRESENTATION_ITEM('')
);
#501=(
BOUNDED_CURVE()
B_SPLINE_CURVE(2,(#35518,#35519,#35520),.UNSPECIFIED.,.F.,.F.)
B_SPLINE_CURVE_WITH_KNOTS((3,3),(-0.271795897845355,-0.218746031477172),
 .UNSPECIFIED.)
CURVE()
GEOMETRIC_REPRESENTATION_ITEM()
RATIONAL_B_SPLINE_CURVE((1.02428162962095,1.02311336089456,1.02147610369989))
REPRESENTATION_ITEM('')
);
#502=(
BOUNDED_CURVE()
B_SPLINE_CURVE(2,(#35522,#35523,#35524),.UNSPECIFIED.,.F.,.F.)
B_SPLINE_CURVE_WITH_KNOTS((3,3),(-0.589144372850602,-0.536094506482415),
 .UNSPECIFIED.)
CURVE()
GEOMETRIC_REPRESENTATION_ITEM()
RATIONAL_B_SPLINE_CURVE((1.02147610369999,1.02311336089467,1.02428162962106))
REPRESENTATION_ITEM('')
);
#503=(
BOUNDED_CURVE()
B_SPLINE_CURVE(2,(#35528,#35529,#35530),.UNSPECIFIED.,.F.,.F.)
B_SPLINE_CURVE_WITH_KNOTS((3,3),(-0.271795897845356,-0.218746031477167),
 .UNSPECIFIED.)
CURVE()
GEOMETRIC_REPRESENTATION_ITEM()
RATIONAL_B_SPLINE_CURVE((1.02428162962107,1.02311336089467,1.02147610369999))
REPRESENTATION_ITEM('')
);
#504=(
BOUNDED_CURVE()
B_SPLINE_CURVE(2,(#35532,#35533,#35534),.UNSPECIFIED.,.F.,.F.)
B_SPLINE_CURVE_WITH_KNOTS((3,3),(-0.589144372850598,-0.53609450648241),
 .UNSPECIFIED.)
CURVE()
GEOMETRIC_REPRESENTATION_ITEM()
RATIONAL_B_SPLINE_CURVE((1.02147610369999,1.02311336089467,1.02428162962106))
REPRESENTATION_ITEM('')
);
#505=(
BOUNDED_CURVE()
B_SPLINE_CURVE(2,(#35538,#35539,#35540),.UNSPECIFIED.,.F.,.F.)
B_SPLINE_CURVE_WITH_KNOTS((3,3),(-0.271795897845352,-0.218746031477168),
 .UNSPECIFIED.)
CURVE()
GEOMETRIC_REPRESENTATION_ITEM()
RATIONAL_B_SPLINE_CURVE((1.02428162962095,1.02311336089457,1.02147610369989))
REPRESENTATION_ITEM('')
);
#506=(
BOUNDED_CURVE()
B_SPLINE_CURVE(2,(#35542,#35543,#35544),.UNSPECIFIED.,.F.,.F.)
B_SPLINE_CURVE_WITH_KNOTS((3,3),(-0.5891443728506,-0.536094506482413),
 .UNSPECIFIED.)
CURVE()
GEOMETRIC_REPRESENTATION_ITEM()
RATIONAL_B_SPLINE_CURVE((1.02147610369997,1.02311336089465,1.02428162962104))
REPRESENTATION_ITEM('')
);
#507=(
BOUNDED_CURVE()
B_SPLINE_CURVE(2,(#35548,#35549,#35550),.UNSPECIFIED.,.F.,.F.)
B_SPLINE_CURVE_WITH_KNOTS((3,3),(-0.271795897845352,-0.218746031477163),
 .UNSPECIFIED.)
CURVE()
GEOMETRIC_REPRESENTATION_ITEM()
RATIONAL_B_SPLINE_CURVE((1.02428162962108,1.02311336089468,1.0214761037))
REPRESENTATION_ITEM('')
);
#508=(
BOUNDED_CURVE()
B_SPLINE_CURVE(2,(#35552,#35553,#35554),.UNSPECIFIED.,.F.,.F.)
B_SPLINE_CURVE_WITH_KNOTS((3,3),(-0.589144372850592,-0.536094506482407),
 .UNSPECIFIED.)
CURVE()
GEOMETRIC_REPRESENTATION_ITEM()
RATIONAL_B_SPLINE_CURVE((1.02147610369993,1.0231133608946,1.02428162962099))
REPRESENTATION_ITEM('')
);
#509=(
BOUNDED_CURVE()
B_SPLINE_CURVE(2,(#35558,#35559,#35560),.UNSPECIFIED.,.F.,.F.)
B_SPLINE_CURVE_WITH_KNOTS((3,3),(-0.271795897845362,-0.218746031477183),
 .UNSPECIFIED.)
CURVE()
GEOMETRIC_REPRESENTATION_ITEM()
RATIONAL_B_SPLINE_CURVE((1.02428162962086,1.02311336089448,1.02147610369982))
REPRESENTATION_ITEM('')
);
#510=(
BOUNDED_CURVE()
B_SPLINE_CURVE(2,(#35562,#35563,#35564),.UNSPECIFIED.,.F.,.F.)
B_SPLINE_CURVE_WITH_KNOTS((3,3),(-0.589144372850588,-0.536094506482407),
 .UNSPECIFIED.)
CURVE()
GEOMETRIC_REPRESENTATION_ITEM()
RATIONAL_B_SPLINE_CURVE((1.02147610369984,1.0231133608945,1.02428162962089))
REPRESENTATION_ITEM('')
);
#511=(
BOUNDED_CURVE()
B_SPLINE_CURVE(2,(#35568,#35569,#35570),.UNSPECIFIED.,.F.,.F.)
B_SPLINE_CURVE_WITH_KNOTS((3,3),(-0.271795897845349,-0.218746031477166),
 .UNSPECIFIED.)
CURVE()
GEOMETRIC_REPRESENTATION_ITEM()
RATIONAL_B_SPLINE_CURVE((1.02428162962096,1.02311336089457,1.0214761036999))
REPRESENTATION_ITEM('')
);
#512=(
BOUNDED_CURVE()
B_SPLINE_CURVE(2,(#35572,#35573,#35574),.UNSPECIFIED.,.F.,.F.)
B_SPLINE_CURVE_WITH_KNOTS((3,3),(-0.589144372850592,-0.536094506482409),
 .UNSPECIFIED.)
CURVE()
GEOMETRIC_REPRESENTATION_ITEM()
RATIONAL_B_SPLINE_CURVE((1.02147610369988,1.02311336089455,1.02428162962093))
REPRESENTATION_ITEM('')
);
#513=(
BOUNDED_CURVE()
B_SPLINE_CURVE(2,(#35578,#35579,#35580),.UNSPECIFIED.,.F.,.F.)
B_SPLINE_CURVE_WITH_KNOTS((3,3),(-0.271795897845356,-0.218746031477174),
 .UNSPECIFIED.)
CURVE()
GEOMETRIC_REPRESENTATION_ITEM()
RATIONAL_B_SPLINE_CURVE((1.0242816296209,1.02311336089451,1.02147610369985))
REPRESENTATION_ITEM('')
);
#514=(
BOUNDED_CURVE()
B_SPLINE_CURVE(2,(#35582,#35583,#35584),.UNSPECIFIED.,.F.,.F.)
B_SPLINE_CURVE_WITH_KNOTS((3,3),(-0.589144372850584,-0.536094506482399),
 .UNSPECIFIED.)
CURVE()
GEOMETRIC_REPRESENTATION_ITEM()
RATIONAL_B_SPLINE_CURVE((1.02147610369989,1.02311336089456,1.02428162962095))
REPRESENTATION_ITEM('')
);
#515=(
BOUNDED_CURVE()
B_SPLINE_CURVE(2,(#35588,#35589,#35590),.UNSPECIFIED.,.F.,.F.)
B_SPLINE_CURVE_WITH_KNOTS((3,3),(-0.271795897845347,-0.218746031477166),
 .UNSPECIFIED.)
CURVE()
GEOMETRIC_REPRESENTATION_ITEM()
RATIONAL_B_SPLINE_CURVE((1.02428162962092,1.02311336089453,1.02147610369987))
REPRESENTATION_ITEM('')
);
#516=(
BOUNDED_CURVE()
B_SPLINE_CURVE(2,(#35592,#35593,#35594),.UNSPECIFIED.,.F.,.F.)
B_SPLINE_CURVE_WITH_KNOTS((3,3),(-0.58914437285059,-0.536094506482399),
 .UNSPECIFIED.)
CURVE()
GEOMETRIC_REPRESENTATION_ITEM()
RATIONAL_B_SPLINE_CURVE((1.02147610370001,1.02311336089469,1.02428162962109))
REPRESENTATION_ITEM('')
);
#517=(
BOUNDED_CURVE()
B_SPLINE_CURVE(2,(#35598,#35599,#35600),.UNSPECIFIED.,.F.,.F.)
B_SPLINE_CURVE_WITH_KNOTS((3,3),(-0.271795897845344,-0.218746031477161),
 .UNSPECIFIED.)
CURVE()
GEOMETRIC_REPRESENTATION_ITEM()
RATIONAL_B_SPLINE_CURVE((1.02428162962097,1.02311336089458,1.02147610369991))
REPRESENTATION_ITEM('')
);
#518=(
BOUNDED_CURVE()
B_SPLINE_CURVE(2,(#35602,#35603,#35604),.UNSPECIFIED.,.F.,.F.)
B_SPLINE_CURVE_WITH_KNOTS((3,3),(-0.589144372850593,-0.536094506482405),
 .UNSPECIFIED.)
CURVE()
GEOMETRIC_REPRESENTATION_ITEM()
RATIONAL_B_SPLINE_CURVE((1.02147610369996,1.02311336089464,1.02428162962103))
REPRESENTATION_ITEM('')
);
#519=(
BOUNDED_CURVE()
B_SPLINE_CURVE(2,(#35608,#35609,#35610),.UNSPECIFIED.,.F.,.F.)
B_SPLINE_CURVE_WITH_KNOTS((3,3),(-0.271795897845349,-0.218746031477166),
 .UNSPECIFIED.)
CURVE()
GEOMETRIC_REPRESENTATION_ITEM()
RATIONAL_B_SPLINE_CURVE((1.02428162962095,1.02311336089457,1.02147610369989))
REPRESENTATION_ITEM('')
);
#520=(
BOUNDED_CURVE()
B_SPLINE_CURVE(2,(#35612,#35613,#35614),.UNSPECIFIED.,.F.,.F.)
B_SPLINE_CURVE_WITH_KNOTS((3,3),(-0.589144372850592,-0.536094506482407),
 .UNSPECIFIED.)
CURVE()
GEOMETRIC_REPRESENTATION_ITEM()
RATIONAL_B_SPLINE_CURVE((1.02147610369992,1.02311336089459,1.02428162962098))
REPRESENTATION_ITEM('')
);
#521=(
BOUNDED_CURVE()
B_SPLINE_CURVE(2,(#35618,#35619,#35620),.UNSPECIFIED.,.F.,.F.)
B_SPLINE_CURVE_WITH_KNOTS((3,3),(-0.271795897845362,-0.218746031477179),
 .UNSPECIFIED.)
CURVE()
GEOMETRIC_REPRESENTATION_ITEM()
RATIONAL_B_SPLINE_CURVE((1.02428162962093,1.02311336089454,1.02147610369987))
REPRESENTATION_ITEM('')
);
#522=(
BOUNDED_CURVE()
B_SPLINE_CURVE(2,(#35622,#35623,#35624),.UNSPECIFIED.,.F.,.F.)
B_SPLINE_CURVE_WITH_KNOTS((3,3),(-0.589144372850592,-0.536094506482405),
 .UNSPECIFIED.)
CURVE()
GEOMETRIC_REPRESENTATION_ITEM()
RATIONAL_B_SPLINE_CURVE((1.02147610369993,1.02311336089461,1.024281629621))
REPRESENTATION_ITEM('')
);
#523=(
BOUNDED_CURVE()
B_SPLINE_CURVE(2,(#35628,#35629,#35630),.UNSPECIFIED.,.F.,.F.)
B_SPLINE_CURVE_WITH_KNOTS((3,3),(-0.271795897845364,-0.218746031477179),
 .UNSPECIFIED.)
CURVE()
GEOMETRIC_REPRESENTATION_ITEM()
RATIONAL_B_SPLINE_CURVE((1.02428162962097,1.02311336089458,1.02147610369991))
REPRESENTATION_ITEM('')
);
#524=(
BOUNDED_CURVE()
B_SPLINE_CURVE(2,(#35632,#35633,#35634),.UNSPECIFIED.,.F.,.F.)
B_SPLINE_CURVE_WITH_KNOTS((3,3),(-0.589144372850588,-0.536094506482402),
 .UNSPECIFIED.)
CURVE()
GEOMETRIC_REPRESENTATION_ITEM()
RATIONAL_B_SPLINE_CURVE((1.02147610369993,1.0231133608946,1.02428162962099))
REPRESENTATION_ITEM('')
);
#525=(
BOUNDED_CURVE()
B_SPLINE_CURVE(2,(#35638,#35639,#35640),.UNSPECIFIED.,.F.,.F.)
B_SPLINE_CURVE_WITH_KNOTS((3,3),(-0.271795897845357,-0.218746031477173),
 .UNSPECIFIED.)
CURVE()
GEOMETRIC_REPRESENTATION_ITEM()
RATIONAL_B_SPLINE_CURVE((1.02428162962094,1.02311336089455,1.02147610369988))
REPRESENTATION_ITEM('')
);
#526=(
BOUNDED_CURVE()
B_SPLINE_CURVE(2,(#35642,#35643,#35644),.UNSPECIFIED.,.F.,.F.)
B_SPLINE_CURVE_WITH_KNOTS((3,3),(-0.589144372850606,-0.536094506482418),
 .UNSPECIFIED.)
CURVE()
GEOMETRIC_REPRESENTATION_ITEM()
RATIONAL_B_SPLINE_CURVE((1.02147610369999,1.02311336089467,1.02428162962107))
REPRESENTATION_ITEM('')
);
#527=(
BOUNDED_CURVE()
B_SPLINE_CURVE(2,(#35648,#35649,#35650),.UNSPECIFIED.,.F.,.F.)
B_SPLINE_CURVE_WITH_KNOTS((3,3),(-0.27179589784536,-0.218746031477177),
 .UNSPECIFIED.)
CURVE()
GEOMETRIC_REPRESENTATION_ITEM()
RATIONAL_B_SPLINE_CURVE((1.02428162962094,1.02311336089455,1.02147610369988))
REPRESENTATION_ITEM('')
);
#528=(
BOUNDED_CURVE()
B_SPLINE_CURVE(2,(#35652,#35653,#35654),.UNSPECIFIED.,.F.,.F.)
B_SPLINE_CURVE_WITH_KNOTS((3,3),(-0.589144372850577,-0.536094506482401),
 .UNSPECIFIED.)
CURVE()
GEOMETRIC_REPRESENTATION_ITEM()
RATIONAL_B_SPLINE_CURVE((1.02147610369975,1.02311336089441,1.02428162962079))
REPRESENTATION_ITEM('')
);
#529=(
BOUNDED_CURVE()
B_SPLINE_CURVE(2,(#35658,#35659,#35660),.UNSPECIFIED.,.F.,.F.)
B_SPLINE_CURVE_WITH_KNOTS((3,3),(-0.271795897845361,-0.218746031477175),
 .UNSPECIFIED.)
CURVE()
GEOMETRIC_REPRESENTATION_ITEM()
RATIONAL_B_SPLINE_CURVE((1.02428162962098,1.02311336089459,1.02147610369992))
REPRESENTATION_ITEM('')
);
#530=(
BOUNDED_CURVE()
B_SPLINE_CURVE(2,(#35662,#35663,#35664),.UNSPECIFIED.,.F.,.F.)
B_SPLINE_CURVE_WITH_KNOTS((3,3),(-0.589144372850604,-0.536094506482412),
 .UNSPECIFIED.)
CURVE()
GEOMETRIC_REPRESENTATION_ITEM()
RATIONAL_B_SPLINE_CURVE((1.02147610370004,1.02311336089473,1.02428162962113))
REPRESENTATION_ITEM('')
);
#531=(
BOUNDED_CURVE()
B_SPLINE_CURVE(2,(#35668,#35669,#35670),.UNSPECIFIED.,.F.,.F.)
B_SPLINE_CURVE_WITH_KNOTS((3,3),(-0.271795897845358,-0.218746031477174),
 .UNSPECIFIED.)
CURVE()
GEOMETRIC_REPRESENTATION_ITEM()
RATIONAL_B_SPLINE_CURVE((1.02428162962094,1.02311336089455,1.02147610369988))
REPRESENTATION_ITEM('')
);
#532=(
BOUNDED_CURVE()
B_SPLINE_CURVE(2,(#35672,#35673,#35674),.UNSPECIFIED.,.F.,.F.)
B_SPLINE_CURVE_WITH_KNOTS((3,3),(-0.589144372850599,-0.536094506482411),
 .UNSPECIFIED.)
CURVE()
GEOMETRIC_REPRESENTATION_ITEM()
RATIONAL_B_SPLINE_CURVE((1.02147610369999,1.02311336089467,1.02428162962106))
REPRESENTATION_ITEM('')
);
#533=(
BOUNDED_CURVE()
B_SPLINE_CURVE(2,(#35678,#35679,#35680),.UNSPECIFIED.,.F.,.F.)
B_SPLINE_CURVE_WITH_KNOTS((3,3),(-0.271795897845357,-0.218746031477171),
 .UNSPECIFIED.)
CURVE()
GEOMETRIC_REPRESENTATION_ITEM()
RATIONAL_B_SPLINE_CURVE((1.02428162962099,1.0231133608946,1.02147610369993))
REPRESENTATION_ITEM('')
);
#534=(
BOUNDED_CURVE()
B_SPLINE_CURVE(2,(#35682,#35683,#35684),.UNSPECIFIED.,.F.,.F.)
B_SPLINE_CURVE_WITH_KNOTS((3,3),(-0.58914437285059,-0.536094506482401),
 .UNSPECIFIED.)
CURVE()
GEOMETRIC_REPRESENTATION_ITEM()
RATIONAL_B_SPLINE_CURVE((1.02147610369998,1.02311336089466,1.02428162962105))
REPRESENTATION_ITEM('')
);
#535=(
BOUNDED_CURVE()
B_SPLINE_CURVE(2,(#35688,#35689,#35690),.UNSPECIFIED.,.F.,.F.)
B_SPLINE_CURVE_WITH_KNOTS((3,3),(-0.271795897845351,-0.218746031477169),
 .UNSPECIFIED.)
CURVE()
GEOMETRIC_REPRESENTATION_ITEM()
RATIONAL_B_SPLINE_CURVE((1.02428162962091,1.02311336089453,1.02147610369986))
REPRESENTATION_ITEM('')
);
#536=(
BOUNDED_CURVE()
B_SPLINE_CURVE(2,(#35692,#35693,#35694),.UNSPECIFIED.,.F.,.F.)
B_SPLINE_CURVE_WITH_KNOTS((3,3),(-0.589144372850574,-0.536094506482395),
 .UNSPECIFIED.)
CURVE()
GEOMETRIC_REPRESENTATION_ITEM()
RATIONAL_B_SPLINE_CURVE((1.02147610369979,1.02311336089445,1.02428162962084))
REPRESENTATION_ITEM('')
);
#537=(
BOUNDED_CURVE()
B_SPLINE_CURVE(2,(#35698,#35699,#35700),.UNSPECIFIED.,.F.,.F.)
B_SPLINE_CURVE_WITH_KNOTS((3,3),(-0.271795897845357,-0.21874603147717),
 .UNSPECIFIED.)
CURVE()
GEOMETRIC_REPRESENTATION_ITEM()
RATIONAL_B_SPLINE_CURVE((1.02428162962101,1.02311336089462,1.02147610369994))
REPRESENTATION_ITEM('')
);
#538=(
BOUNDED_CURVE()
B_SPLINE_CURVE(2,(#35702,#35703,#35704),.UNSPECIFIED.,.F.,.F.)
B_SPLINE_CURVE_WITH_KNOTS((3,3),(-0.589144372850572,-0.536094506482391),
 .UNSPECIFIED.)
CURVE()
GEOMETRIC_REPRESENTATION_ITEM()
RATIONAL_B_SPLINE_CURVE((1.02147610369981,1.02311336089448,1.02428162962086))
REPRESENTATION_ITEM('')
);
#539=(
BOUNDED_CURVE()
B_SPLINE_CURVE(2,(#35708,#35709,#35710),.UNSPECIFIED.,.F.,.F.)
B_SPLINE_CURVE_WITH_KNOTS((3,3),(-0.271795897845355,-0.218746031477175),
 .UNSPECIFIED.)
CURVE()
GEOMETRIC_REPRESENTATION_ITEM()
RATIONAL_B_SPLINE_CURVE((1.02428162962088,1.02311336089449,1.02147610369983))
REPRESENTATION_ITEM('')
);
#540=(
BOUNDED_CURVE()
B_SPLINE_CURVE(2,(#35712,#35713,#35714),.UNSPECIFIED.,.F.,.F.)
B_SPLINE_CURVE_WITH_KNOTS((3,3),(-0.589144372850594,-0.53609450648241),
 .UNSPECIFIED.)
CURVE()
GEOMETRIC_REPRESENTATION_ITEM()
RATIONAL_B_SPLINE_CURVE((1.02147610369989,1.02311336089456,1.02428162962095))
REPRESENTATION_ITEM('')
);
#541=(
BOUNDED_CURVE()
B_SPLINE_CURVE(2,(#35718,#35719,#35720),.UNSPECIFIED.,.F.,.F.)
B_SPLINE_CURVE_WITH_KNOTS((3,3),(-0.271795897845355,-0.218746031477174),
 .UNSPECIFIED.)
CURVE()
GEOMETRIC_REPRESENTATION_ITEM()
RATIONAL_B_SPLINE_CURVE((1.0242816296209,1.02311336089451,1.02147610369984))
REPRESENTATION_ITEM('')
);
#542=(
BOUNDED_CURVE()
B_SPLINE_CURVE(2,(#35722,#35723,#35724),.UNSPECIFIED.,.F.,.F.)
B_SPLINE_CURVE_WITH_KNOTS((3,3),(-0.589144372850579,-0.536094506482395),
 .UNSPECIFIED.)
CURVE()
GEOMETRIC_REPRESENTATION_ITEM()
RATIONAL_B_SPLINE_CURVE((1.02147610369989,1.02311336089457,1.02428162962095))
REPRESENTATION_ITEM('')
);
#543=(
BOUNDED_CURVE()
B_SPLINE_CURVE(2,(#35728,#35729,#35730),.UNSPECIFIED.,.F.,.F.)
B_SPLINE_CURVE_WITH_KNOTS((3,3),(-0.271795897845349,-0.218746031477161),
 .UNSPECIFIED.)
CURVE()
GEOMETRIC_REPRESENTATION_ITEM()
RATIONAL_B_SPLINE_CURVE((1.02428162962106,1.02311336089467,1.02147610369999))
REPRESENTATION_ITEM('')
);
#544=(
BOUNDED_CURVE()
B_SPLINE_CURVE(2,(#35732,#35733,#35734),.UNSPECIFIED.,.F.,.F.)
B_SPLINE_CURVE_WITH_KNOTS((3,3),(-0.589144372850575,-0.536094506482389),
 .UNSPECIFIED.)
CURVE()
GEOMETRIC_REPRESENTATION_ITEM()
RATIONAL_B_SPLINE_CURVE((1.02147610369993,1.0231133608946,1.02428162962099))
REPRESENTATION_ITEM('')
);
#545=(
BOUNDED_CURVE()
B_SPLINE_CURVE(2,(#35738,#35739,#35740),.UNSPECIFIED.,.F.,.F.)
B_SPLINE_CURVE_WITH_KNOTS((3,3),(-0.271795897845358,-0.218746031477173),
 .UNSPECIFIED.)
CURVE()
GEOMETRIC_REPRESENTATION_ITEM()
RATIONAL_B_SPLINE_CURVE((1.02428162962099,1.0231133608946,1.02147610369993))
REPRESENTATION_ITEM('')
);
#546=(
BOUNDED_CURVE()
B_SPLINE_CURVE(2,(#35742,#35743,#35744),.UNSPECIFIED.,.F.,.F.)
B_SPLINE_CURVE_WITH_KNOTS((3,3),(-0.589144372850595,-0.536094506482406),
 .UNSPECIFIED.)
CURVE()
GEOMETRIC_REPRESENTATION_ITEM()
RATIONAL_B_SPLINE_CURVE((1.02147610369996,1.02311336089464,1.02428162962103))
REPRESENTATION_ITEM('')
);
#547=(
BOUNDED_CURVE()
B_SPLINE_CURVE(2,(#35748,#35749,#35750),.UNSPECIFIED.,.F.,.F.)
B_SPLINE_CURVE_WITH_KNOTS((3,3),(-0.271795897845368,-0.218746031477185),
 .UNSPECIFIED.)
CURVE()
GEOMETRIC_REPRESENTATION_ITEM()
RATIONAL_B_SPLINE_CURVE((1.02428162962092,1.02311336089454,1.02147610369987))
REPRESENTATION_ITEM('')
);
#548=(
BOUNDED_CURVE()
B_SPLINE_CURVE(2,(#35752,#35753,#35754),.UNSPECIFIED.,.F.,.F.)
B_SPLINE_CURVE_WITH_KNOTS((3,3),(-0.589144372850581,-0.536094506482396),
 .UNSPECIFIED.)
CURVE()
GEOMETRIC_REPRESENTATION_ITEM()
RATIONAL_B_SPLINE_CURVE((1.02147610369993,1.0231133608946,1.02428162962099))
REPRESENTATION_ITEM('')
);
#549=(
BOUNDED_CURVE()
B_SPLINE_CURVE(2,(#35758,#35759,#35760),.UNSPECIFIED.,.F.,.F.)
B_SPLINE_CURVE_WITH_KNOTS((3,3),(-0.271795897845348,-0.218746031477166),
 .UNSPECIFIED.)
CURVE()
GEOMETRIC_REPRESENTATION_ITEM()
RATIONAL_B_SPLINE_CURVE((1.02428162962094,1.02311336089455,1.02147610369988))
REPRESENTATION_ITEM('')
);
#550=(
BOUNDED_CURVE()
B_SPLINE_CURVE(2,(#35762,#35763,#35764),.UNSPECIFIED.,.F.,.F.)
B_SPLINE_CURVE_WITH_KNOTS((3,3),(-0.589144372850584,-0.536094506482403),
 .UNSPECIFIED.)
CURVE()
GEOMETRIC_REPRESENTATION_ITEM()
RATIONAL_B_SPLINE_CURVE((1.02147610369986,1.02311336089453,1.02428162962092))
REPRESENTATION_ITEM('')
);
#551=(
BOUNDED_CURVE()
B_SPLINE_CURVE(2,(#35767,#35768,#35769),.UNSPECIFIED.,.F.,.F.)
B_SPLINE_CURVE_WITH_KNOTS((3,3),(-0.271795897845352,-0.218746031477171),
 .UNSPECIFIED.)
CURVE()
GEOMETRIC_REPRESENTATION_ITEM()
RATIONAL_B_SPLINE_CURVE((1.02428162962091,1.02311336089452,1.02147610369985))
REPRESENTATION_ITEM('')
);
#552=(
BOUNDED_CURVE()
B_SPLINE_CURVE(2,(#36567,#36568,#36569),.UNSPECIFIED.,.F.,.F.)
B_SPLINE_CURVE_WITH_KNOTS((3,3),(0.536094506482412,0.5891443728506),
 .UNSPECIFIED.)
CURVE()
GEOMETRIC_REPRESENTATION_ITEM()
RATIONAL_B_SPLINE_CURVE((1.02428162962103,1.02311336089463,1.02147610369996))
REPRESENTATION_ITEM('')
);
#553=(
BOUNDED_CURVE()
B_SPLINE_CURVE(2,(#36573,#36574,#36575),.UNSPECIFIED.,.F.,.F.)
B_SPLINE_CURVE_WITH_KNOTS((3,3),(-0.27179589784535,-0.218746031477165),
 .UNSPECIFIED.)
CURVE()
GEOMETRIC_REPRESENTATION_ITEM()
RATIONAL_B_SPLINE_CURVE((1.02428162962098,1.02311336089459,1.02147610369991))
REPRESENTATION_ITEM('')
);
#554=(
BOUNDED_CURVE()
B_SPLINE_CURVE(2,(#36577,#36578,#36579),.UNSPECIFIED.,.F.,.F.)
B_SPLINE_CURVE_WITH_KNOTS((3,3),(-0.589144372850602,-0.536094506482414),
 .UNSPECIFIED.)
CURVE()
GEOMETRIC_REPRESENTATION_ITEM()
RATIONAL_B_SPLINE_CURVE((1.02147610369995,1.02311336089463,1.02428162962102))
REPRESENTATION_ITEM('')
);
#555=(
BOUNDED_CURVE()
B_SPLINE_CURVE(2,(#36583,#36584,#36585),.UNSPECIFIED.,.F.,.F.)
B_SPLINE_CURVE_WITH_KNOTS((3,3),(-0.271795897845356,-0.218746031477171),
 .UNSPECIFIED.)
CURVE()
GEOMETRIC_REPRESENTATION_ITEM()
RATIONAL_B_SPLINE_CURVE((1.02428162962098,1.02311336089459,1.02147610369991))
REPRESENTATION_ITEM('')
);
#556=(
BOUNDED_CURVE()
B_SPLINE_CURVE(2,(#36587,#36588,#36589),.UNSPECIFIED.,.F.,.F.)
B_SPLINE_CURVE_WITH_KNOTS((3,3),(-0.589144372850587,-0.536094506482402),
 .UNSPECIFIED.)
CURVE()
GEOMETRIC_REPRESENTATION_ITEM()
RATIONAL_B_SPLINE_CURVE((1.02147610369992,1.0231133608946,1.02428162962099))
REPRESENTATION_ITEM('')
);
#557=(
BOUNDED_CURVE()
B_SPLINE_CURVE(2,(#36593,#36594,#36595),.UNSPECIFIED.,.F.,.F.)
B_SPLINE_CURVE_WITH_KNOTS((3,3),(-0.271795897845345,-0.218746031477163),
 .UNSPECIFIED.)
CURVE()
GEOMETRIC_REPRESENTATION_ITEM()
RATIONAL_B_SPLINE_CURVE((1.02428162962094,1.02311336089455,1.02147610369988))
REPRESENTATION_ITEM('')
);
#558=(
BOUNDED_CURVE()
B_SPLINE_CURVE(2,(#36597,#36598,#36599),.UNSPECIFIED.,.F.,.F.)
B_SPLINE_CURVE_WITH_KNOTS((3,3),(-0.589144372850589,-0.536094506482405),
 .UNSPECIFIED.)
CURVE()
GEOMETRIC_REPRESENTATION_ITEM()
RATIONAL_B_SPLINE_CURVE((1.02147610369991,1.02311336089458,1.02428162962097))
REPRESENTATION_ITEM('')
);
#559=(
BOUNDED_CURVE()
B_SPLINE_CURVE(2,(#36603,#36604,#36605),.UNSPECIFIED.,.F.,.F.)
B_SPLINE_CURVE_WITH_KNOTS((3,3),(-0.271795897845365,-0.218746031477182),
 .UNSPECIFIED.)
CURVE()
GEOMETRIC_REPRESENTATION_ITEM()
RATIONAL_B_SPLINE_CURVE((1.02428162962089,1.02311336089451,1.02147610369984))
REPRESENTATION_ITEM('')
);
#560=(
BOUNDED_CURVE()
B_SPLINE_CURVE(2,(#36607,#36608,#36609),.UNSPECIFIED.,.F.,.F.)
B_SPLINE_CURVE_WITH_KNOTS((3,3),(-0.589144372850583,-0.536094506482398),
 .UNSPECIFIED.)
CURVE()
GEOMETRIC_REPRESENTATION_ITEM()
RATIONAL_B_SPLINE_CURVE((1.02147610369992,1.02311336089459,1.02428162962098))
REPRESENTATION_ITEM('')
);
#561=(
BOUNDED_CURVE()
B_SPLINE_CURVE(2,(#36613,#36614,#36615),.UNSPECIFIED.,.F.,.F.)
B_SPLINE_CURVE_WITH_KNOTS((3,3),(-0.271795897845351,-0.218746031477163),
 .UNSPECIFIED.)
CURVE()
GEOMETRIC_REPRESENTATION_ITEM()
RATIONAL_B_SPLINE_CURVE((1.02428162962104,1.02311336089465,1.02147610369997))
REPRESENTATION_ITEM('')
);
#562=(
BOUNDED_CURVE()
B_SPLINE_CURVE(2,(#36617,#36618,#36619),.UNSPECIFIED.,.F.,.F.)
B_SPLINE_CURVE_WITH_KNOTS((3,3),(-0.589144372850602,-0.536094506482419),
 .UNSPECIFIED.)
CURVE()
GEOMETRIC_REPRESENTATION_ITEM()
RATIONAL_B_SPLINE_CURVE((1.02147610369988,1.02311336089455,1.02428162962094))
REPRESENTATION_ITEM('')
);
#563=(
BOUNDED_CURVE()
B_SPLINE_CURVE(2,(#36623,#36624,#36625),.UNSPECIFIED.,.F.,.F.)
B_SPLINE_CURVE_WITH_KNOTS((3,3),(-0.271795897845357,-0.21874603147717),
 .UNSPECIFIED.)
CURVE()
GEOMETRIC_REPRESENTATION_ITEM()
RATIONAL_B_SPLINE_CURVE((1.02428162962102,1.02311336089463,1.02147610369995))
REPRESENTATION_ITEM('')
);
#564=(
BOUNDED_CURVE()
B_SPLINE_CURVE(2,(#36627,#36628,#36629),.UNSPECIFIED.,.F.,.F.)
B_SPLINE_CURVE_WITH_KNOTS((3,3),(-0.589144372850595,-0.536094506482411),
 .UNSPECIFIED.)
CURVE()
GEOMETRIC_REPRESENTATION_ITEM()
RATIONAL_B_SPLINE_CURVE((1.02147610369988,1.02311336089455,1.02428162962094))
REPRESENTATION_ITEM('')
);
#565=(
BOUNDED_CURVE()
B_SPLINE_CURVE(2,(#36633,#36634,#36635),.UNSPECIFIED.,.F.,.F.)
B_SPLINE_CURVE_WITH_KNOTS((3,3),(-0.271795897845351,-0.218746031477165),
 .UNSPECIFIED.)
CURVE()
GEOMETRIC_REPRESENTATION_ITEM()
RATIONAL_B_SPLINE_CURVE((1.02428162962101,1.02311336089462,1.02147610369994))
REPRESENTATION_ITEM('')
);
#566=(
BOUNDED_CURVE()
B_SPLINE_CURVE(2,(#36637,#36638,#36639),.UNSPECIFIED.,.F.,.F.)
B_SPLINE_CURVE_WITH_KNOTS((3,3),(-0.589144372850605,-0.536094506482423),
 .UNSPECIFIED.)
CURVE()
GEOMETRIC_REPRESENTATION_ITEM()
RATIONAL_B_SPLINE_CURVE((1.02147610369987,1.02311336089453,1.02428162962092))
REPRESENTATION_ITEM('')
);
#567=(
BOUNDED_CURVE()
B_SPLINE_CURVE(2,(#36643,#36644,#36645),.UNSPECIFIED.,.F.,.F.)
B_SPLINE_CURVE_WITH_KNOTS((3,3),(-0.271795897845359,-0.218746031477179),
 .UNSPECIFIED.)
CURVE()
GEOMETRIC_REPRESENTATION_ITEM()
RATIONAL_B_SPLINE_CURVE((1.02428162962085,1.02311336089447,1.02147610369981))
REPRESENTATION_ITEM('')
);
#568=(
BOUNDED_CURVE()
B_SPLINE_CURVE(2,(#36647,#36648,#36649),.UNSPECIFIED.,.F.,.F.)
B_SPLINE_CURVE_WITH_KNOTS((3,3),(-0.589144372850621,-0.536094506482433),
 .UNSPECIFIED.)
CURVE()
GEOMETRIC_REPRESENTATION_ITEM()
RATIONAL_B_SPLINE_CURVE((1.02147610369998,1.02311336089466,1.02428162962105))
REPRESENTATION_ITEM('')
);
#569=(
BOUNDED_CURVE()
B_SPLINE_CURVE(2,(#36653,#36654,#36655),.UNSPECIFIED.,.F.,.F.)
B_SPLINE_CURVE_WITH_KNOTS((3,3),(-0.271795897845357,-0.218746031477166),
 .UNSPECIFIED.)
CURVE()
GEOMETRIC_REPRESENTATION_ITEM()
RATIONAL_B_SPLINE_CURVE((1.02428162962107,1.02311336089468,1.0214761037))
REPRESENTATION_ITEM('')
);
#570=(
BOUNDED_CURVE()
B_SPLINE_CURVE(2,(#36657,#36658,#36659),.UNSPECIFIED.,.F.,.F.)
B_SPLINE_CURVE_WITH_KNOTS((3,3),(-0.589144372850594,-0.536094506482414),
 .UNSPECIFIED.)
CURVE()
GEOMETRIC_REPRESENTATION_ITEM()
RATIONAL_B_SPLINE_CURVE((1.02147610369981,1.02311336089447,1.02428162962085))
REPRESENTATION_ITEM('')
);
#571=(
BOUNDED_CURVE()
B_SPLINE_CURVE(2,(#36663,#36664,#36665),.UNSPECIFIED.,.F.,.F.)
B_SPLINE_CURVE_WITH_KNOTS((3,3),(-0.271795897845359,-0.218746031477176),
 .UNSPECIFIED.)
CURVE()
GEOMETRIC_REPRESENTATION_ITEM()
RATIONAL_B_SPLINE_CURVE((1.02428162962093,1.02311336089454,1.02147610369987))
REPRESENTATION_ITEM('')
);
#572=(
BOUNDED_CURVE()
B_SPLINE_CURVE(2,(#36667,#36668,#36669),.UNSPECIFIED.,.F.,.F.)
B_SPLINE_CURVE_WITH_KNOTS((3,3),(-0.589144372850597,-0.536094506482409),
 .UNSPECIFIED.)
CURVE()
GEOMETRIC_REPRESENTATION_ITEM()
RATIONAL_B_SPLINE_CURVE((1.02147610369995,1.02311336089463,1.02428162962102))
REPRESENTATION_ITEM('')
);
#573=(
BOUNDED_CURVE()
B_SPLINE_CURVE(2,(#36673,#36674,#36675),.UNSPECIFIED.,.F.,.F.)
B_SPLINE_CURVE_WITH_KNOTS((3,3),(-0.271795897845349,-0.218746031477168),
 .UNSPECIFIED.)
CURVE()
GEOMETRIC_REPRESENTATION_ITEM()
RATIONAL_B_SPLINE_CURVE((1.02428162962088,1.0231133608945,1.02147610369983))
REPRESENTATION_ITEM('')
);
#574=(
BOUNDED_CURVE()
B_SPLINE_CURVE(2,(#36677,#36678,#36679),.UNSPECIFIED.,.F.,.F.)
B_SPLINE_CURVE_WITH_KNOTS((3,3),(-0.589144372850612,-0.536094506482427),
 .UNSPECIFIED.)
CURVE()
GEOMETRIC_REPRESENTATION_ITEM()
RATIONAL_B_SPLINE_CURVE((1.02147610369991,1.02311336089458,1.02428162962097))
REPRESENTATION_ITEM('')
);
#575=(
BOUNDED_CURVE()
B_SPLINE_CURVE(2,(#36683,#36684,#36685),.UNSPECIFIED.,.F.,.F.)
B_SPLINE_CURVE_WITH_KNOTS((3,3),(-0.27179589784536,-0.218746031477173),
 .UNSPECIFIED.)
CURVE()
GEOMETRIC_REPRESENTATION_ITEM()
RATIONAL_B_SPLINE_CURVE((1.02428162962101,1.02311336089462,1.02147610369994))
REPRESENTATION_ITEM('')
);
#576=(
BOUNDED_CURVE()
B_SPLINE_CURVE(2,(#36687,#36688,#36689),.UNSPECIFIED.,.F.,.F.)
B_SPLINE_CURVE_WITH_KNOTS((3,3),(-0.589144372850594,-0.536094506482412),
 .UNSPECIFIED.)
CURVE()
GEOMETRIC_REPRESENTATION_ITEM()
RATIONAL_B_SPLINE_CURVE((1.02147610369986,1.02311336089453,1.02428162962092))
REPRESENTATION_ITEM('')
);
#577=(
BOUNDED_CURVE()
B_SPLINE_CURVE(2,(#36693,#36694,#36695),.UNSPECIFIED.,.F.,.F.)
B_SPLINE_CURVE_WITH_KNOTS((3,3),(-0.271795897845352,-0.218746031477168),
 .UNSPECIFIED.)
CURVE()
GEOMETRIC_REPRESENTATION_ITEM()
RATIONAL_B_SPLINE_CURVE((1.02428162962095,1.02311336089456,1.02147610369989))
REPRESENTATION_ITEM('')
);
#578=(
BOUNDED_CURVE()
B_SPLINE_CURVE(2,(#36697,#36698,#36699),.UNSPECIFIED.,.F.,.F.)
B_SPLINE_CURVE_WITH_KNOTS((3,3),(-0.589144372850596,-0.536094506482406),
 .UNSPECIFIED.)
CURVE()
GEOMETRIC_REPRESENTATION_ITEM()
RATIONAL_B_SPLINE_CURVE((1.02147610369999,1.02311336089467,1.02428162962107))
REPRESENTATION_ITEM('')
);
#579=(
BOUNDED_CURVE()
B_SPLINE_CURVE(2,(#36703,#36704,#36705),.UNSPECIFIED.,.F.,.F.)
B_SPLINE_CURVE_WITH_KNOTS((3,3),(-0.271795897845352,-0.218746031477168),
 .UNSPECIFIED.)
CURVE()
GEOMETRIC_REPRESENTATION_ITEM()
RATIONAL_B_SPLINE_CURVE((1.02428162962096,1.02311336089457,1.0214761036999))
REPRESENTATION_ITEM('')
);
#580=(
BOUNDED_CURVE()
B_SPLINE_CURVE(2,(#36707,#36708,#36709),.UNSPECIFIED.,.F.,.F.)
B_SPLINE_CURVE_WITH_KNOTS((3,3),(-0.589144372850588,-0.536094506482405),
 .UNSPECIFIED.)
CURVE()
GEOMETRIC_REPRESENTATION_ITEM()
RATIONAL_B_SPLINE_CURVE((1.02147610369987,1.02311336089454,1.02428162962093))
REPRESENTATION_ITEM('')
);
#581=(
BOUNDED_CURVE()
B_SPLINE_CURVE(2,(#36713,#36714,#36715),.UNSPECIFIED.,.F.,.F.)
B_SPLINE_CURVE_WITH_KNOTS((3,3),(-0.271795897845354,-0.218746031477172),
 .UNSPECIFIED.)
CURVE()
GEOMETRIC_REPRESENTATION_ITEM()
RATIONAL_B_SPLINE_CURVE((1.0242816296209,1.02311336089451,1.02147610369984))
REPRESENTATION_ITEM('')
);
#582=(
BOUNDED_CURVE()
B_SPLINE_CURVE(2,(#36717,#36718,#36719),.UNSPECIFIED.,.F.,.F.)
B_SPLINE_CURVE_WITH_KNOTS((3,3),(-0.589144372850593,-0.536094506482412),
 .UNSPECIFIED.)
CURVE()
GEOMETRIC_REPRESENTATION_ITEM()
RATIONAL_B_SPLINE_CURVE((1.02147610369985,1.02311336089452,1.0242816296209))
REPRESENTATION_ITEM('')
);
#583=(
BOUNDED_CURVE()
B_SPLINE_CURVE(2,(#36723,#36724,#36725),.UNSPECIFIED.,.F.,.F.)
B_SPLINE_CURVE_WITH_KNOTS((3,3),(-0.271795897845351,-0.218746031477167),
 .UNSPECIFIED.)
CURVE()
GEOMETRIC_REPRESENTATION_ITEM()
RATIONAL_B_SPLINE_CURVE((1.02428162962095,1.02311336089456,1.02147610369989))
REPRESENTATION_ITEM('')
);
#584=(
BOUNDED_CURVE()
B_SPLINE_CURVE(2,(#36727,#36728,#36729),.UNSPECIFIED.,.F.,.F.)
B_SPLINE_CURVE_WITH_KNOTS((3,3),(-0.589144372850603,-0.536094506482421),
 .UNSPECIFIED.)
CURVE()
GEOMETRIC_REPRESENTATION_ITEM()
RATIONAL_B_SPLINE_CURVE((1.02147610369987,1.02311336089454,1.02428162962092))
REPRESENTATION_ITEM('')
);
#585=(
BOUNDED_CURVE()
B_SPLINE_CURVE(2,(#36733,#36734,#36735),.UNSPECIFIED.,.F.,.F.)
B_SPLINE_CURVE_WITH_KNOTS((3,3),(-0.271795897845345,-0.218746031477162),
 .UNSPECIFIED.)
CURVE()
GEOMETRIC_REPRESENTATION_ITEM()
RATIONAL_B_SPLINE_CURVE((1.02428162962095,1.02311336089456,1.02147610369989))
REPRESENTATION_ITEM('')
);
#586=(
BOUNDED_CURVE()
B_SPLINE_CURVE(2,(#36737,#36738,#36739),.UNSPECIFIED.,.F.,.F.)
B_SPLINE_CURVE_WITH_KNOTS((3,3),(-0.589144372850587,-0.536094506482405),
 .UNSPECIFIED.)
CURVE()
GEOMETRIC_REPRESENTATION_ITEM()
RATIONAL_B_SPLINE_CURVE((1.02147610369987,1.02311336089454,1.02428162962092))
REPRESENTATION_ITEM('')
);
#587=(
BOUNDED_CURVE()
B_SPLINE_CURVE(2,(#36743,#36744,#36745),.UNSPECIFIED.,.F.,.F.)
B_SPLINE_CURVE_WITH_KNOTS((3,3),(-0.271795897845357,-0.218746031477178),
 .UNSPECIFIED.)
CURVE()
GEOMETRIC_REPRESENTATION_ITEM()
RATIONAL_B_SPLINE_CURVE((1.02428162962083,1.02311336089445,1.02147610369978))
REPRESENTATION_ITEM('')
);
#588=(
BOUNDED_CURVE()
B_SPLINE_CURVE(2,(#36747,#36748,#36749),.UNSPECIFIED.,.F.,.F.)
B_SPLINE_CURVE_WITH_KNOTS((3,3),(-0.589144372850587,-0.536094506482403),
 .UNSPECIFIED.)
CURVE()
GEOMETRIC_REPRESENTATION_ITEM()
RATIONAL_B_SPLINE_CURVE((1.02147610369989,1.02311336089456,1.02428162962095))
REPRESENTATION_ITEM('')
);
#589=(
BOUNDED_CURVE()
B_SPLINE_CURVE(2,(#36753,#36754,#36755),.UNSPECIFIED.,.F.,.F.)
B_SPLINE_CURVE_WITH_KNOTS((3,3),(-0.271795897845361,-0.218746031477177),
 .UNSPECIFIED.)
CURVE()
GEOMETRIC_REPRESENTATION_ITEM()
RATIONAL_B_SPLINE_CURVE((1.02428162962093,1.02311336089454,1.02147610369987))
REPRESENTATION_ITEM('')
);
#590=(
BOUNDED_CURVE()
B_SPLINE_CURVE(2,(#36757,#36758,#36759),.UNSPECIFIED.,.F.,.F.)
B_SPLINE_CURVE_WITH_KNOTS((3,3),(-0.589144372850603,-0.536094506482419),
 .UNSPECIFIED.)
CURVE()
GEOMETRIC_REPRESENTATION_ITEM()
RATIONAL_B_SPLINE_CURVE((1.02147610369989,1.02311336089457,1.02428162962095))
REPRESENTATION_ITEM('')
);
#591=(
BOUNDED_CURVE()
B_SPLINE_CURVE(2,(#36763,#36764,#36765),.UNSPECIFIED.,.F.,.F.)
B_SPLINE_CURVE_WITH_KNOTS((3,3),(-0.271795897845354,-0.21874603147717),
 .UNSPECIFIED.)
CURVE()
GEOMETRIC_REPRESENTATION_ITEM()
RATIONAL_B_SPLINE_CURVE((1.02428162962096,1.02311336089457,1.0214761036999))
REPRESENTATION_ITEM('')
);
#592=(
BOUNDED_CURVE()
B_SPLINE_CURVE(2,(#36767,#36768,#36769),.UNSPECIFIED.,.F.,.F.)
B_SPLINE_CURVE_WITH_KNOTS((3,3),(-0.589144372850597,-0.536094506482414),
 .UNSPECIFIED.)
CURVE()
GEOMETRIC_REPRESENTATION_ITEM()
RATIONAL_B_SPLINE_CURVE((1.02147610369986,1.02311336089453,1.02428162962092))
REPRESENTATION_ITEM('')
);
#593=(
BOUNDED_CURVE()
B_SPLINE_CURVE(2,(#36773,#36774,#36775),.UNSPECIFIED.,.F.,.F.)
B_SPLINE_CURVE_WITH_KNOTS((3,3),(-0.271795897845355,-0.218746031477174),
 .UNSPECIFIED.)
CURVE()
GEOMETRIC_REPRESENTATION_ITEM()
RATIONAL_B_SPLINE_CURVE((1.02428162962089,1.0231133608945,1.02147610369983))
REPRESENTATION_ITEM('')
);
#594=(
BOUNDED_CURVE()
B_SPLINE_CURVE(2,(#36777,#36778,#36779),.UNSPECIFIED.,.F.,.F.)
B_SPLINE_CURVE_WITH_KNOTS((3,3),(-0.589144372850588,-0.536094506482404),
 .UNSPECIFIED.)
CURVE()
GEOMETRIC_REPRESENTATION_ITEM()
RATIONAL_B_SPLINE_CURVE((1.02147610369988,1.02311336089455,1.02428162962094))
REPRESENTATION_ITEM('')
);
#595=(
BOUNDED_CURVE()
B_SPLINE_CURVE(2,(#36783,#36784,#36785),.UNSPECIFIED.,.F.,.F.)
B_SPLINE_CURVE_WITH_KNOTS((3,3),(-0.271795897845348,-0.218746031477163),
 .UNSPECIFIED.)
CURVE()
GEOMETRIC_REPRESENTATION_ITEM()
RATIONAL_B_SPLINE_CURVE((1.02428162962099,1.0231133608946,1.02147610369993))
REPRESENTATION_ITEM('')
);
#596=(
BOUNDED_CURVE()
B_SPLINE_CURVE(2,(#36787,#36788,#36789),.UNSPECIFIED.,.F.,.F.)
B_SPLINE_CURVE_WITH_KNOTS((3,3),(-0.589144372850592,-0.536094506482408),
 .UNSPECIFIED.)
CURVE()
GEOMETRIC_REPRESENTATION_ITEM()
RATIONAL_B_SPLINE_CURVE((1.0214761036999,1.02311336089457,1.02428162962096))
REPRESENTATION_ITEM('')
);
#597=(
BOUNDED_CURVE()
B_SPLINE_CURVE(2,(#36793,#36794,#36795),.UNSPECIFIED.,.F.,.F.)
B_SPLINE_CURVE_WITH_KNOTS((3,3),(-0.271795897845357,-0.218746031477176),
 .UNSPECIFIED.)
CURVE()
GEOMETRIC_REPRESENTATION_ITEM()
RATIONAL_B_SPLINE_CURVE((1.02428162962088,1.02311336089449,1.02147610369983))
REPRESENTATION_ITEM('')
);
#598=(
BOUNDED_CURVE()
B_SPLINE_CURVE(2,(#36797,#36798,#36799),.UNSPECIFIED.,.F.,.F.)
B_SPLINE_CURVE_WITH_KNOTS((3,3),(-0.589144372850592,-0.536094506482406),
 .UNSPECIFIED.)
CURVE()
GEOMETRIC_REPRESENTATION_ITEM()
RATIONAL_B_SPLINE_CURVE((1.02147610369992,1.02311336089459,1.02428162962098))
REPRESENTATION_ITEM('')
);
#599=(
BOUNDED_CURVE()
B_SPLINE_CURVE(2,(#36803,#36804,#36805),.UNSPECIFIED.,.F.,.F.)
B_SPLINE_CURVE_WITH_KNOTS((3,3),(-0.27179589784536,-0.218746031477179),
 .UNSPECIFIED.)
CURVE()
GEOMETRIC_REPRESENTATION_ITEM()
RATIONAL_B_SPLINE_CURVE((1.02428162962089,1.0231133608945,1.02147610369984))
REPRESENTATION_ITEM('')
);
#600=(
BOUNDED_CURVE()
B_SPLINE_CURVE(2,(#36807,#36808,#36809),.UNSPECIFIED.,.F.,.F.)
B_SPLINE_CURVE_WITH_KNOTS((3,3),(-0.589144372850584,-0.536094506482402),
 .UNSPECIFIED.)
CURVE()
GEOMETRIC_REPRESENTATION_ITEM()
RATIONAL_B_SPLINE_CURVE((1.02147610369986,1.02311336089453,1.02428162962092))
REPRESENTATION_ITEM('')
);
#601=(
BOUNDED_CURVE()
B_SPLINE_CURVE(2,(#36813,#36814,#36815),.UNSPECIFIED.,.F.,.F.)
B_SPLINE_CURVE_WITH_KNOTS((3,3),(-0.271795897845342,-0.218746031477156),
 .UNSPECIFIED.)
CURVE()
GEOMETRIC_REPRESENTATION_ITEM()
RATIONAL_B_SPLINE_CURVE((1.02428162962101,1.02311336089462,1.02147610369994))
REPRESENTATION_ITEM('')
);
#602=(
BOUNDED_CURVE()
B_SPLINE_CURVE(2,(#36817,#36818,#36819),.UNSPECIFIED.,.F.,.F.)
B_SPLINE_CURVE_WITH_KNOTS((3,3),(-0.589144372850578,-0.536094506482394),
 .UNSPECIFIED.)
CURVE()
GEOMETRIC_REPRESENTATION_ITEM()
RATIONAL_B_SPLINE_CURVE((1.02147610369987,1.02311336089454,1.02428162962093))
REPRESENTATION_ITEM('')
);
#603=(
BOUNDED_CURVE()
B_SPLINE_CURVE(2,(#36823,#36824,#36825),.UNSPECIFIED.,.F.,.F.)
B_SPLINE_CURVE_WITH_KNOTS((3,3),(-0.271795897845354,-0.21874603147717),
 .UNSPECIFIED.)
CURVE()
GEOMETRIC_REPRESENTATION_ITEM()
RATIONAL_B_SPLINE_CURVE((1.02428162962094,1.02311336089455,1.02147610369988))
REPRESENTATION_ITEM('')
);
#604=(
BOUNDED_CURVE()
B_SPLINE_CURVE(2,(#36827,#36828,#36829),.UNSPECIFIED.,.F.,.F.)
B_SPLINE_CURVE_WITH_KNOTS((3,3),(-0.589144372850586,-0.536094506482403),
 .UNSPECIFIED.)
CURVE()
GEOMETRIC_REPRESENTATION_ITEM()
RATIONAL_B_SPLINE_CURVE((1.02147610369988,1.02311336089455,1.02428162962094))
REPRESENTATION_ITEM('')
);
#605=(
BOUNDED_CURVE()
B_SPLINE_CURVE(2,(#36833,#36834,#36835),.UNSPECIFIED.,.F.,.F.)
B_SPLINE_CURVE_WITH_KNOTS((3,3),(-0.271795897845349,-0.218746031477164),
 .UNSPECIFIED.)
CURVE()
GEOMETRIC_REPRESENTATION_ITEM()
RATIONAL_B_SPLINE_CURVE((1.02428162962096,1.02311336089458,1.0214761036999))
REPRESENTATION_ITEM('')
);
#606=(
BOUNDED_CURVE()
B_SPLINE_CURVE(2,(#36837,#36838,#36839),.UNSPECIFIED.,.F.,.F.)
B_SPLINE_CURVE_WITH_KNOTS((3,3),(-0.589144372850588,-0.536094506482402),
 .UNSPECIFIED.)
CURVE()
GEOMETRIC_REPRESENTATION_ITEM()
RATIONAL_B_SPLINE_CURVE((1.02147610369991,1.02311336089459,1.02428162962098))
REPRESENTATION_ITEM('')
);
#607=(
BOUNDED_CURVE()
B_SPLINE_CURVE(2,(#36843,#36844,#36845),.UNSPECIFIED.,.F.,.F.)
B_SPLINE_CURVE_WITH_KNOTS((3,3),(-0.271795897845353,-0.218746031477165),
 .UNSPECIFIED.)
CURVE()
GEOMETRIC_REPRESENTATION_ITEM()
RATIONAL_B_SPLINE_CURVE((1.02428162962104,1.02311336089465,1.02147610369997))
REPRESENTATION_ITEM('')
);
#608=(
BOUNDED_CURVE()
B_SPLINE_CURVE(2,(#36847,#36848,#36849),.UNSPECIFIED.,.F.,.F.)
B_SPLINE_CURVE_WITH_KNOTS((3,3),(-0.589144372850592,-0.536094506482409),
 .UNSPECIFIED.)
CURVE()
GEOMETRIC_REPRESENTATION_ITEM()
RATIONAL_B_SPLINE_CURVE((1.02147610369986,1.02311336089453,1.02428162962092))
REPRESENTATION_ITEM('')
);
#609=(
BOUNDED_CURVE()
B_SPLINE_CURVE(2,(#36853,#36854,#36855),.UNSPECIFIED.,.F.,.F.)
B_SPLINE_CURVE_WITH_KNOTS((3,3),(-0.271795897845343,-0.218746031477159),
 .UNSPECIFIED.)
CURVE()
GEOMETRIC_REPRESENTATION_ITEM()
RATIONAL_B_SPLINE_CURVE((1.02428162962097,1.02311336089458,1.0214761036999))
REPRESENTATION_ITEM('')
);
#610=(
BOUNDED_CURVE()
B_SPLINE_CURVE(2,(#36857,#36858,#36859),.UNSPECIFIED.,.F.,.F.)
B_SPLINE_CURVE_WITH_KNOTS((3,3),(-0.589144372850575,-0.536094506482395),
 .UNSPECIFIED.)
CURVE()
GEOMETRIC_REPRESENTATION_ITEM()
RATIONAL_B_SPLINE_CURVE((1.0214761036998,1.02311336089446,1.02428162962085))
REPRESENTATION_ITEM('')
);
#611=(
BOUNDED_CURVE()
B_SPLINE_CURVE(2,(#36863,#36864,#36865),.UNSPECIFIED.,.F.,.F.)
B_SPLINE_CURVE_WITH_KNOTS((3,3),(-0.271795897845356,-0.218746031477172),
 .UNSPECIFIED.)
CURVE()
GEOMETRIC_REPRESENTATION_ITEM()
RATIONAL_B_SPLINE_CURVE((1.02428162962094,1.02311336089456,1.02147610369988))
REPRESENTATION_ITEM('')
);
#612=(
BOUNDED_CURVE()
B_SPLINE_CURVE(2,(#36867,#36868,#36869),.UNSPECIFIED.,.F.,.F.)
B_SPLINE_CURVE_WITH_KNOTS((3,3),(-0.589144372850588,-0.536094506482404),
 .UNSPECIFIED.)
CURVE()
GEOMETRIC_REPRESENTATION_ITEM()
RATIONAL_B_SPLINE_CURVE((1.02147610369989,1.02311336089456,1.02428162962095))
REPRESENTATION_ITEM('')
);
#613=(
BOUNDED_CURVE()
B_SPLINE_CURVE(2,(#36873,#36874,#36875),.UNSPECIFIED.,.F.,.F.)
B_SPLINE_CURVE_WITH_KNOTS((3,3),(-0.271795897845355,-0.21874603147717),
 .UNSPECIFIED.)
CURVE()
GEOMETRIC_REPRESENTATION_ITEM()
RATIONAL_B_SPLINE_CURVE((1.02428162962098,1.02311336089459,1.02147610369992))
REPRESENTATION_ITEM('')
);
#614=(
BOUNDED_CURVE()
B_SPLINE_CURVE(2,(#36877,#36878,#36879),.UNSPECIFIED.,.F.,.F.)
B_SPLINE_CURVE_WITH_KNOTS((3,3),(-0.589144372850597,-0.536094506482411),
 .UNSPECIFIED.)
CURVE()
GEOMETRIC_REPRESENTATION_ITEM()
RATIONAL_B_SPLINE_CURVE((1.02147610369993,1.0231133608946,1.024281629621))
REPRESENTATION_ITEM('')
);
#615=(
BOUNDED_CURVE()
B_SPLINE_CURVE(2,(#36883,#36884,#36885),.UNSPECIFIED.,.F.,.F.)
B_SPLINE_CURVE_WITH_KNOTS((3,3),(-0.271795897845346,-0.218746031477162),
 .UNSPECIFIED.)
CURVE()
GEOMETRIC_REPRESENTATION_ITEM()
RATIONAL_B_SPLINE_CURVE((1.02428162962096,1.02311336089457,1.0214761036999))
REPRESENTATION_ITEM('')
);
#616=(
BOUNDED_CURVE()
B_SPLINE_CURVE(2,(#36887,#36888,#36889),.UNSPECIFIED.,.F.,.F.)
B_SPLINE_CURVE_WITH_KNOTS((3,3),(-0.589144372850587,-0.536094506482401),
 .UNSPECIFIED.)
CURVE()
GEOMETRIC_REPRESENTATION_ITEM()
RATIONAL_B_SPLINE_CURVE((1.02147610369994,1.02311336089461,1.024281629621))
REPRESENTATION_ITEM('')
);
#617=(
BOUNDED_CURVE()
B_SPLINE_CURVE(2,(#36893,#36894,#36895),.UNSPECIFIED.,.F.,.F.)
B_SPLINE_CURVE_WITH_KNOTS((3,3),(-0.271795897845345,-0.218746031477163),
 .UNSPECIFIED.)
CURVE()
GEOMETRIC_REPRESENTATION_ITEM()
RATIONAL_B_SPLINE_CURVE((1.02428162962093,1.02311336089454,1.02147610369987))
REPRESENTATION_ITEM('')
);
#618=(
BOUNDED_CURVE()
B_SPLINE_CURVE(2,(#36897,#36898,#36899),.UNSPECIFIED.,.F.,.F.)
B_SPLINE_CURVE_WITH_KNOTS((3,3),(-0.589144372850582,-0.5360945064824),
 .UNSPECIFIED.)
CURVE()
GEOMETRIC_REPRESENTATION_ITEM()
RATIONAL_B_SPLINE_CURVE((1.02147610369986,1.02311336089452,1.02428162962091))
REPRESENTATION_ITEM('')
);
#619=(
BOUNDED_CURVE()
B_SPLINE_CURVE(2,(#36903,#36904,#36905),.UNSPECIFIED.,.F.,.F.)
B_SPLINE_CURVE_WITH_KNOTS((3,3),(-0.271795897845348,-0.218746031477163),
 .UNSPECIFIED.)
CURVE()
GEOMETRIC_REPRESENTATION_ITEM()
RATIONAL_B_SPLINE_CURVE((1.02428162962098,1.02311336089459,1.02147610369992))
REPRESENTATION_ITEM('')
);
#620=(
BOUNDED_CURVE()
B_SPLINE_CURVE(2,(#36907,#36908,#36909),.UNSPECIFIED.,.F.,.F.)
B_SPLINE_CURVE_WITH_KNOTS((3,3),(-0.589144372850595,-0.536094506482406),
 .UNSPECIFIED.)
CURVE()
GEOMETRIC_REPRESENTATION_ITEM()
RATIONAL_B_SPLINE_CURVE((1.02147610369997,1.02311336089465,1.02428162962104))
REPRESENTATION_ITEM('')
);
#621=(
BOUNDED_CURVE()
B_SPLINE_CURVE(2,(#36913,#36914,#36915),.UNSPECIFIED.,.F.,.F.)
B_SPLINE_CURVE_WITH_KNOTS((3,3),(-0.271795897845349,-0.218746031477164),
 .UNSPECIFIED.)
CURVE()
GEOMETRIC_REPRESENTATION_ITEM()
RATIONAL_B_SPLINE_CURVE((1.02428162962097,1.02311336089458,1.02147610369991))
REPRESENTATION_ITEM('')
);
#622=(
BOUNDED_CURVE()
B_SPLINE_CURVE(2,(#36917,#36918,#36919),.UNSPECIFIED.,.F.,.F.)
B_SPLINE_CURVE_WITH_KNOTS((3,3),(-0.589144372850605,-0.536094506482415),
 .UNSPECIFIED.)
CURVE()
GEOMETRIC_REPRESENTATION_ITEM()
RATIONAL_B_SPLINE_CURVE((1.02147610369999,1.02311336089467,1.02428162962106))
REPRESENTATION_ITEM('')
);
#623=(
BOUNDED_CURVE()
B_SPLINE_CURVE(2,(#36923,#36924,#36925),.UNSPECIFIED.,.F.,.F.)
B_SPLINE_CURVE_WITH_KNOTS((3,3),(-0.271795897845347,-0.218746031477163),
 .UNSPECIFIED.)
CURVE()
GEOMETRIC_REPRESENTATION_ITEM()
RATIONAL_B_SPLINE_CURVE((1.02428162962095,1.02311336089456,1.02147610369989))
REPRESENTATION_ITEM('')
);
#624=(
BOUNDED_CURVE()
B_SPLINE_CURVE(2,(#36927,#36928,#36929),.UNSPECIFIED.,.F.,.F.)
B_SPLINE_CURVE_WITH_KNOTS((3,3),(-0.589144372850588,-0.53609450648241),
 .UNSPECIFIED.)
CURVE()
GEOMETRIC_REPRESENTATION_ITEM()
RATIONAL_B_SPLINE_CURVE((1.0214761036998,1.02311336089446,1.02428162962085))
REPRESENTATION_ITEM('')
);
#625=(
BOUNDED_CURVE()
B_SPLINE_CURVE(2,(#36933,#36934,#36935),.UNSPECIFIED.,.F.,.F.)
B_SPLINE_CURVE_WITH_KNOTS((3,3),(-0.271795897845344,-0.218746031477158),
 .UNSPECIFIED.)
CURVE()
GEOMETRIC_REPRESENTATION_ITEM()
RATIONAL_B_SPLINE_CURVE((1.024281629621,1.02311336089461,1.02147610369994))
REPRESENTATION_ITEM('')
);
#626=(
BOUNDED_CURVE()
B_SPLINE_CURVE(2,(#36937,#36938,#36939),.UNSPECIFIED.,.F.,.F.)
B_SPLINE_CURVE_WITH_KNOTS((3,3),(-0.589144372850618,-0.536094506482433),
 .UNSPECIFIED.)
CURVE()
GEOMETRIC_REPRESENTATION_ITEM()
RATIONAL_B_SPLINE_CURVE((1.0214761036999,1.02311336089457,1.02428162962096))
REPRESENTATION_ITEM('')
);
#627=(
BOUNDED_CURVE()
B_SPLINE_CURVE(2,(#36943,#36944,#36945),.UNSPECIFIED.,.F.,.F.)
B_SPLINE_CURVE_WITH_KNOTS((3,3),(-0.271795897845356,-0.218746031477172),
 .UNSPECIFIED.)
CURVE()
GEOMETRIC_REPRESENTATION_ITEM()
RATIONAL_B_SPLINE_CURVE((1.02428162962095,1.02311336089456,1.02147610369989))
REPRESENTATION_ITEM('')
);
#628=(
BOUNDED_CURVE()
B_SPLINE_CURVE(2,(#36947,#36948,#36949),.UNSPECIFIED.,.F.,.F.)
B_SPLINE_CURVE_WITH_KNOTS((3,3),(-0.589144372850593,-0.53609450648241),
 .UNSPECIFIED.)
CURVE()
GEOMETRIC_REPRESENTATION_ITEM()
RATIONAL_B_SPLINE_CURVE((1.02147610369989,1.02311336089456,1.02428162962095))
REPRESENTATION_ITEM('')
);
#629=(
BOUNDED_CURVE()
B_SPLINE_CURVE(2,(#36953,#36954,#36955),.UNSPECIFIED.,.F.,.F.)
B_SPLINE_CURVE_WITH_KNOTS((3,3),(-0.271795897845356,-0.27009889353462),
 .UNSPECIFIED.)
CURVE()
GEOMETRIC_REPRESENTATION_ITEM()
RATIONAL_B_SPLINE_CURVE((1.024281629621,1.0242442580459,1.02420640656117))
REPRESENTATION_ITEM('')
);
#630=(
BOUNDED_CURVE()
B_SPLINE_CURVE(2,(#36960,#36961,#36962),.UNSPECIFIED.,.F.,.F.)
B_SPLINE_CURVE_WITH_KNOTS((3,3),(-0.27009889353462,-0.21874603147717),
 .UNSPECIFIED.)
CURVE()
GEOMETRIC_REPRESENTATION_ITEM()
RATIONAL_B_SPLINE_CURVE((1.02420640656117,1.02306098691693,1.02147610369993))
REPRESENTATION_ITEM('')
);
#631=(
BOUNDED_CURVE()
B_SPLINE_CURVE(2,(#36964,#36965,#36966),.UNSPECIFIED.,.F.,.F.)
B_SPLINE_CURVE_WITH_KNOTS((3,3),(-0.589144372850598,-0.536094506482415),
 .UNSPECIFIED.)
CURVE()
GEOMETRIC_REPRESENTATION_ITEM()
RATIONAL_B_SPLINE_CURVE((1.02147610369988,1.02311336089455,1.02428162962093))
REPRESENTATION_ITEM('')
);
#632=(
BOUNDED_CURVE()
B_SPLINE_CURVE(2,(#36970,#36971,#36972),.UNSPECIFIED.,.F.,.F.)
B_SPLINE_CURVE_WITH_KNOTS((3,3),(-0.271795897845352,-0.218746031477165),
 .UNSPECIFIED.)
CURVE()
GEOMETRIC_REPRESENTATION_ITEM()
RATIONAL_B_SPLINE_CURVE((1.02428162962101,1.02311336089462,1.02147610369994))
REPRESENTATION_ITEM('')
);
#633=(
BOUNDED_CURVE()
B_SPLINE_CURVE(2,(#36974,#36975,#36976),.UNSPECIFIED.,.F.,.F.)
B_SPLINE_CURVE_WITH_KNOTS((3,3),(-0.589144372850592,-0.536094506482404),
 .UNSPECIFIED.)
CURVE()
GEOMETRIC_REPRESENTATION_ITEM()
RATIONAL_B_SPLINE_CURVE((1.02147610369997,1.02311336089465,1.02428162962104))
REPRESENTATION_ITEM('')
);
#634=(
BOUNDED_CURVE()
B_SPLINE_CURVE(2,(#36980,#36981,#36982),.UNSPECIFIED.,.F.,.F.)
B_SPLINE_CURVE_WITH_KNOTS((3,3),(-0.27179589784535,-0.218746031477166),
 .UNSPECIFIED.)
CURVE()
GEOMETRIC_REPRESENTATION_ITEM()
RATIONAL_B_SPLINE_CURVE((1.02428162962095,1.02311336089456,1.02147610369989))
REPRESENTATION_ITEM('')
);
#635=(
BOUNDED_CURVE()
B_SPLINE_CURVE(2,(#36984,#36985,#36986),.UNSPECIFIED.,.F.,.F.)
B_SPLINE_CURVE_WITH_KNOTS((3,3),(-0.589144372850593,-0.536094506482409),
 .UNSPECIFIED.)
CURVE()
GEOMETRIC_REPRESENTATION_ITEM()
RATIONAL_B_SPLINE_CURVE((1.02147610369989,1.02311336089456,1.02428162962095))
REPRESENTATION_ITEM('')
);
#636=(
BOUNDED_CURVE()
B_SPLINE_CURVE(2,(#36990,#36991,#36992),.UNSPECIFIED.,.F.,.F.)
B_SPLINE_CURVE_WITH_KNOTS((3,3),(-0.27179589784535,-0.218746031477166),
 .UNSPECIFIED.)
CURVE()
GEOMETRIC_REPRESENTATION_ITEM()
RATIONAL_B_SPLINE_CURVE((1.02428162962097,1.02311336089458,1.02147610369991))
REPRESENTATION_ITEM('')
);
#637=(
BOUNDED_CURVE()
B_SPLINE_CURVE(2,(#36994,#36995,#36996),.UNSPECIFIED.,.F.,.F.)
B_SPLINE_CURVE_WITH_KNOTS((3,3),(-0.589144372850588,-0.536094506482405),
 .UNSPECIFIED.)
CURVE()
GEOMETRIC_REPRESENTATION_ITEM()
RATIONAL_B_SPLINE_CURVE((1.02147610369989,1.02311336089456,1.02428162962095))
REPRESENTATION_ITEM('')
);
#638=(
BOUNDED_CURVE()
B_SPLINE_CURVE(2,(#37000,#37001,#37002),.UNSPECIFIED.,.F.,.F.)
B_SPLINE_CURVE_WITH_KNOTS((3,3),(-0.271795897845364,-0.218746031477175),
 .UNSPECIFIED.)
CURVE()
GEOMETRIC_REPRESENTATION_ITEM()
RATIONAL_B_SPLINE_CURVE((1.02428162962103,1.02311336089464,1.02147610369996))
REPRESENTATION_ITEM('')
);
#639=(
BOUNDED_CURVE()
B_SPLINE_CURVE(2,(#37004,#37005,#37006),.UNSPECIFIED.,.F.,.F.)
B_SPLINE_CURVE_WITH_KNOTS((3,3),(-0.589144372850586,-0.5360945064824),
 .UNSPECIFIED.)
CURVE()
GEOMETRIC_REPRESENTATION_ITEM()
RATIONAL_B_SPLINE_CURVE((1.02147610369993,1.0231133608946,1.02428162962099))
REPRESENTATION_ITEM('')
);
#640=(
BOUNDED_CURVE()
B_SPLINE_CURVE(2,(#37010,#37011,#37012),.UNSPECIFIED.,.F.,.F.)
B_SPLINE_CURVE_WITH_KNOTS((3,3),(-0.271795897845344,-0.218746031477157),
 .UNSPECIFIED.)
CURVE()
GEOMETRIC_REPRESENTATION_ITEM()
RATIONAL_B_SPLINE_CURVE((1.02428162962104,1.02311336089464,1.02147610369997))
REPRESENTATION_ITEM('')
);
#641=(
BOUNDED_CURVE()
B_SPLINE_CURVE(2,(#37014,#37015,#37016),.UNSPECIFIED.,.F.,.F.)
B_SPLINE_CURVE_WITH_KNOTS((3,3),(-0.589144372850594,-0.536094506482411),
 .UNSPECIFIED.)
CURVE()
GEOMETRIC_REPRESENTATION_ITEM()
RATIONAL_B_SPLINE_CURVE((1.02147610369987,1.02311336089454,1.02428162962093))
REPRESENTATION_ITEM('')
);
#642=(
BOUNDED_CURVE()
B_SPLINE_CURVE(2,(#37020,#37021,#37022),.UNSPECIFIED.,.F.,.F.)
B_SPLINE_CURVE_WITH_KNOTS((3,3),(-0.271795897845363,-0.218746031477177),
 .UNSPECIFIED.)
CURVE()
GEOMETRIC_REPRESENTATION_ITEM()
RATIONAL_B_SPLINE_CURVE((1.02428162962096,1.02311336089457,1.0214761036999))
REPRESENTATION_ITEM('')
);
#643=(
BOUNDED_CURVE()
B_SPLINE_CURVE(2,(#37024,#37025,#37026),.UNSPECIFIED.,.F.,.F.)
B_SPLINE_CURVE_WITH_KNOTS((3,3),(-0.589144372850603,-0.536094506482417),
 .UNSPECIFIED.)
CURVE()
GEOMETRIC_REPRESENTATION_ITEM()
RATIONAL_B_SPLINE_CURVE((1.02147610369994,1.02311336089461,1.024281629621))
REPRESENTATION_ITEM('')
);
#644=(
BOUNDED_CURVE()
B_SPLINE_CURVE(2,(#37030,#37031,#37032),.UNSPECIFIED.,.F.,.F.)
B_SPLINE_CURVE_WITH_KNOTS((3,3),(-0.271795897845351,-0.218746031477165),
 .UNSPECIFIED.)
CURVE()
GEOMETRIC_REPRESENTATION_ITEM()
RATIONAL_B_SPLINE_CURVE((1.024281629621,1.02311336089461,1.02147610369993))
REPRESENTATION_ITEM('')
);
#645=(
BOUNDED_CURVE()
B_SPLINE_CURVE(2,(#37034,#37035,#37036),.UNSPECIFIED.,.F.,.F.)
B_SPLINE_CURVE_WITH_KNOTS((3,3),(-0.589144372850587,-0.536094506482401),
 .UNSPECIFIED.)
CURVE()
GEOMETRIC_REPRESENTATION_ITEM()
RATIONAL_B_SPLINE_CURVE((1.02147610369992,1.02311336089459,1.02428162962098))
REPRESENTATION_ITEM('')
);
#646=(
BOUNDED_CURVE()
B_SPLINE_CURVE(2,(#37040,#37041,#37042),.UNSPECIFIED.,.F.,.F.)
B_SPLINE_CURVE_WITH_KNOTS((3,3),(-0.271795897845358,-0.218746031477172),
 .UNSPECIFIED.)
CURVE()
GEOMETRIC_REPRESENTATION_ITEM()
RATIONAL_B_SPLINE_CURVE((1.02428162962097,1.02311336089458,1.02147610369991))
REPRESENTATION_ITEM('')
);
#647=(
BOUNDED_CURVE()
B_SPLINE_CURVE(2,(#37044,#37045,#37046),.UNSPECIFIED.,.F.,.F.)
B_SPLINE_CURVE_WITH_KNOTS((3,3),(-0.589144372850593,-0.536094506482406),
 .UNSPECIFIED.)
CURVE()
GEOMETRIC_REPRESENTATION_ITEM()
RATIONAL_B_SPLINE_CURVE((1.02147610369993,1.02311336089461,1.024281629621))
REPRESENTATION_ITEM('')
);
#648=(
BOUNDED_CURVE()
B_SPLINE_CURVE(2,(#37050,#37051,#37052),.UNSPECIFIED.,.F.,.F.)
B_SPLINE_CURVE_WITH_KNOTS((3,3),(-0.271795897845347,-0.218746031477162),
 .UNSPECIFIED.)
CURVE()
GEOMETRIC_REPRESENTATION_ITEM()
RATIONAL_B_SPLINE_CURVE((1.02428162962098,1.02311336089459,1.02147610369992))
REPRESENTATION_ITEM('')
);
#649=(
BOUNDED_CURVE()
B_SPLINE_CURVE(2,(#37054,#37055,#37056),.UNSPECIFIED.,.F.,.F.)
B_SPLINE_CURVE_WITH_KNOTS((3,3),(-0.5891443728506,-0.536094506482414),
 .UNSPECIFIED.)
CURVE()
GEOMETRIC_REPRESENTATION_ITEM()
RATIONAL_B_SPLINE_CURVE((1.02147610369995,1.02311336089463,1.02428162962102))
REPRESENTATION_ITEM('')
);
#650=(
BOUNDED_CURVE()
B_SPLINE_CURVE(2,(#37060,#37061,#37062),.UNSPECIFIED.,.F.,.F.)
B_SPLINE_CURVE_WITH_KNOTS((3,3),(-0.271795897845356,-0.218746031477171),
 .UNSPECIFIED.)
CURVE()
GEOMETRIC_REPRESENTATION_ITEM()
RATIONAL_B_SPLINE_CURVE((1.02428162962096,1.02311336089457,1.0214761036999))
REPRESENTATION_ITEM('')
);
#651=(
BOUNDED_CURVE()
B_SPLINE_CURVE(2,(#37064,#37065,#37066),.UNSPECIFIED.,.F.,.F.)
B_SPLINE_CURVE_WITH_KNOTS((3,3),(-0.589144372850587,-0.536094506482402),
 .UNSPECIFIED.)
CURVE()
GEOMETRIC_REPRESENTATION_ITEM()
RATIONAL_B_SPLINE_CURVE((1.02147610369992,1.02311336089459,1.02428162962098))
REPRESENTATION_ITEM('')
);
#652=(
BOUNDED_CURVE()
B_SPLINE_CURVE(2,(#37070,#37071,#37072),.UNSPECIFIED.,.F.,.F.)
B_SPLINE_CURVE_WITH_KNOTS((3,3),(-0.271795897845355,-0.21874603147717),
 .UNSPECIFIED.)
CURVE()
GEOMETRIC_REPRESENTATION_ITEM()
RATIONAL_B_SPLINE_CURVE((1.02428162962097,1.02311336089458,1.0214761036999))
REPRESENTATION_ITEM('')
);
#653=(
BOUNDED_CURVE()
B_SPLINE_CURVE(2,(#37074,#37075,#37076),.UNSPECIFIED.,.F.,.F.)
B_SPLINE_CURVE_WITH_KNOTS((3,3),(-0.589144372850594,-0.53609450648241),
 .UNSPECIFIED.)
CURVE()
GEOMETRIC_REPRESENTATION_ITEM()
RATIONAL_B_SPLINE_CURVE((1.0214761036999,1.02311336089457,1.02428162962096))
REPRESENTATION_ITEM('')
);
#654=(
BOUNDED_CURVE()
B_SPLINE_CURVE(2,(#37080,#37081,#37082),.UNSPECIFIED.,.F.,.F.)
B_SPLINE_CURVE_WITH_KNOTS((3,3),(-0.271795897845353,-0.218746031477171),
 .UNSPECIFIED.)
CURVE()
GEOMETRIC_REPRESENTATION_ITEM()
RATIONAL_B_SPLINE_CURVE((1.02428162962091,1.02311336089453,1.02147610369986))
REPRESENTATION_ITEM('')
);
#655=(
BOUNDED_CURVE()
B_SPLINE_CURVE(2,(#37084,#37085,#37086),.UNSPECIFIED.,.F.,.F.)
B_SPLINE_CURVE_WITH_KNOTS((3,3),(-0.589144372850593,-0.536094506482411),
 .UNSPECIFIED.)
CURVE()
GEOMETRIC_REPRESENTATION_ITEM()
RATIONAL_B_SPLINE_CURVE((1.02147610369985,1.02311336089452,1.0242816296209))
REPRESENTATION_ITEM('')
);
#656=(
BOUNDED_CURVE()
B_SPLINE_CURVE(2,(#37090,#37091,#37092),.UNSPECIFIED.,.F.,.F.)
B_SPLINE_CURVE_WITH_KNOTS((3,3),(-0.27179589784535,-0.218746031477166),
 .UNSPECIFIED.)
CURVE()
GEOMETRIC_REPRESENTATION_ITEM()
RATIONAL_B_SPLINE_CURVE((1.02428162962095,1.02311336089457,1.02147610369989))
REPRESENTATION_ITEM('')
);
#657=(
BOUNDED_CURVE()
B_SPLINE_CURVE(2,(#37094,#37095,#37096),.UNSPECIFIED.,.F.,.F.)
B_SPLINE_CURVE_WITH_KNOTS((3,3),(-0.589144372850597,-0.536094506482411),
 .UNSPECIFIED.)
CURVE()
GEOMETRIC_REPRESENTATION_ITEM()
RATIONAL_B_SPLINE_CURVE((1.02147610369993,1.0231133608946,1.02428162962099))
REPRESENTATION_ITEM('')
);
#658=(
BOUNDED_CURVE()
B_SPLINE_CURVE(2,(#37100,#37101,#37102),.UNSPECIFIED.,.F.,.F.)
B_SPLINE_CURVE_WITH_KNOTS((3,3),(-0.271795897845352,-0.218746031477167),
 .UNSPECIFIED.)
CURVE()
GEOMETRIC_REPRESENTATION_ITEM()
RATIONAL_B_SPLINE_CURVE((1.02428162962097,1.02311336089458,1.02147610369991))
REPRESENTATION_ITEM('')
);
#659=(
BOUNDED_CURVE()
B_SPLINE_CURVE(2,(#37104,#37105,#37106),.UNSPECIFIED.,.F.,.F.)
B_SPLINE_CURVE_WITH_KNOTS((3,3),(-0.589144372850601,-0.536094506482415),
 .UNSPECIFIED.)
CURVE()
GEOMETRIC_REPRESENTATION_ITEM()
RATIONAL_B_SPLINE_CURVE((1.02147610369994,1.02311336089461,1.024281629621))
REPRESENTATION_ITEM('')
);
#660=(
BOUNDED_CURVE()
B_SPLINE_CURVE(2,(#37110,#37111,#37112),.UNSPECIFIED.,.F.,.F.)
B_SPLINE_CURVE_WITH_KNOTS((3,3),(-0.271795897845354,-0.21874603147717),
 .UNSPECIFIED.)
CURVE()
GEOMETRIC_REPRESENTATION_ITEM()
RATIONAL_B_SPLINE_CURVE((1.02428162962094,1.02311336089455,1.02147610369988))
REPRESENTATION_ITEM('')
);
#661=(
BOUNDED_CURVE()
B_SPLINE_CURVE(2,(#37114,#37115,#37116),.UNSPECIFIED.,.F.,.F.)
B_SPLINE_CURVE_WITH_KNOTS((3,3),(-0.589144372850587,-0.536094506482405),
 .UNSPECIFIED.)
CURVE()
GEOMETRIC_REPRESENTATION_ITEM()
RATIONAL_B_SPLINE_CURVE((1.02147610369984,1.02311336089451,1.02428162962089))
REPRESENTATION_ITEM('')
);
#662=(
BOUNDED_CURVE()
B_SPLINE_CURVE(2,(#37120,#37121,#37122),.UNSPECIFIED.,.F.,.F.)
B_SPLINE_CURVE_WITH_KNOTS((3,3),(-0.271795897845346,-0.218746031477161),
 .UNSPECIFIED.)
CURVE()
GEOMETRIC_REPRESENTATION_ITEM()
RATIONAL_B_SPLINE_CURVE((1.02428162962098,1.02311336089459,1.02147610369992))
REPRESENTATION_ITEM('')
);
#663=(
BOUNDED_CURVE()
B_SPLINE_CURVE(2,(#37124,#37125,#37126),.UNSPECIFIED.,.F.,.F.)
B_SPLINE_CURVE_WITH_KNOTS((3,3),(-0.589144372850597,-0.536094506482412),
 .UNSPECIFIED.)
CURVE()
GEOMETRIC_REPRESENTATION_ITEM()
RATIONAL_B_SPLINE_CURVE((1.02147610369992,1.02311336089459,1.02428162962098))
REPRESENTATION_ITEM('')
);
#664=(
BOUNDED_CURVE()
B_SPLINE_CURVE(2,(#37130,#37131,#37132),.UNSPECIFIED.,.F.,.F.)
B_SPLINE_CURVE_WITH_KNOTS((3,3),(-0.271795897845346,-0.218746031477161),
 .UNSPECIFIED.)
CURVE()
GEOMETRIC_REPRESENTATION_ITEM()
RATIONAL_B_SPLINE_CURVE((1.02428162962099,1.0231133608946,1.02147610369993))
REPRESENTATION_ITEM('')
);
#665=(
BOUNDED_CURVE()
B_SPLINE_CURVE(2,(#37134,#37135,#37136),.UNSPECIFIED.,.F.,.F.)
B_SPLINE_CURVE_WITH_KNOTS((3,3),(-0.589144372850585,-0.536094506482398),
 .UNSPECIFIED.)
CURVE()
GEOMETRIC_REPRESENTATION_ITEM()
RATIONAL_B_SPLINE_CURVE((1.02147610369994,1.02311336089461,1.024281629621))
REPRESENTATION_ITEM('')
);
#666=(
BOUNDED_CURVE()
B_SPLINE_CURVE(2,(#37140,#37141,#37142),.UNSPECIFIED.,.F.,.F.)
B_SPLINE_CURVE_WITH_KNOTS((3,3),(-0.271795897845348,-0.218746031477163),
 .UNSPECIFIED.)
CURVE()
GEOMETRIC_REPRESENTATION_ITEM()
RATIONAL_B_SPLINE_CURVE((1.02428162962098,1.02311336089459,1.02147610369992))
REPRESENTATION_ITEM('')
);
#667=(
BOUNDED_CURVE()
B_SPLINE_CURVE(2,(#37144,#37145,#37146),.UNSPECIFIED.,.F.,.F.)
B_SPLINE_CURVE_WITH_KNOTS((3,3),(-0.589144372850599,-0.536094506482412),
 .UNSPECIFIED.)
CURVE()
GEOMETRIC_REPRESENTATION_ITEM()
RATIONAL_B_SPLINE_CURVE((1.02147610369994,1.02311336089462,1.02428162962101))
REPRESENTATION_ITEM('')
);
#668=(
BOUNDED_CURVE()
B_SPLINE_CURVE(2,(#37150,#37151,#37152),.UNSPECIFIED.,.F.,.F.)
B_SPLINE_CURVE_WITH_KNOTS((3,3),(-0.271795897845354,-0.21874603147717),
 .UNSPECIFIED.)
CURVE()
GEOMETRIC_REPRESENTATION_ITEM()
RATIONAL_B_SPLINE_CURVE((1.02428162962095,1.02311336089456,1.02147610369989))
REPRESENTATION_ITEM('')
);
#669=(
BOUNDED_CURVE()
B_SPLINE_CURVE(2,(#37154,#37155,#37156),.UNSPECIFIED.,.F.,.F.)
B_SPLINE_CURVE_WITH_KNOTS((3,3),(-0.589144372850593,-0.536094506482408),
 .UNSPECIFIED.)
CURVE()
GEOMETRIC_REPRESENTATION_ITEM()
RATIONAL_B_SPLINE_CURVE((1.0214761036999,1.02311336089457,1.02428162962096))
REPRESENTATION_ITEM('')
);
#670=(
BOUNDED_CURVE()
B_SPLINE_CURVE(2,(#37160,#37161,#37162),.UNSPECIFIED.,.F.,.F.)
B_SPLINE_CURVE_WITH_KNOTS((3,3),(-0.271795897845352,-0.218746031477169),
 .UNSPECIFIED.)
CURVE()
GEOMETRIC_REPRESENTATION_ITEM()
RATIONAL_B_SPLINE_CURVE((1.02428162962095,1.02311336089456,1.02147610369989))
REPRESENTATION_ITEM('')
);
#671=(
BOUNDED_CURVE()
B_SPLINE_CURVE(2,(#37164,#37165,#37166),.UNSPECIFIED.,.F.,.F.)
B_SPLINE_CURVE_WITH_KNOTS((3,3),(-0.589144372850587,-0.536094506482401),
 .UNSPECIFIED.)
CURVE()
GEOMETRIC_REPRESENTATION_ITEM()
RATIONAL_B_SPLINE_CURVE((1.02147610369991,1.02311336089458,1.02428162962097))
REPRESENTATION_ITEM('')
);
#672=(
BOUNDED_CURVE()
B_SPLINE_CURVE(2,(#37170,#37171,#37172),.UNSPECIFIED.,.F.,.F.)
B_SPLINE_CURVE_WITH_KNOTS((3,3),(-0.271795897845353,-0.218746031477167),
 .UNSPECIFIED.)
CURVE()
GEOMETRIC_REPRESENTATION_ITEM()
RATIONAL_B_SPLINE_CURVE((1.02428162962099,1.0231133608946,1.02147610369993))
REPRESENTATION_ITEM('')
);
#673=(
BOUNDED_CURVE()
B_SPLINE_CURVE(2,(#37174,#37175,#37176),.UNSPECIFIED.,.F.,.F.)
B_SPLINE_CURVE_WITH_KNOTS((3,3),(-0.589144372850597,-0.536094506482414),
 .UNSPECIFIED.)
CURVE()
GEOMETRIC_REPRESENTATION_ITEM()
RATIONAL_B_SPLINE_CURVE((1.02147610369988,1.02311336089455,1.02428162962094))
REPRESENTATION_ITEM('')
);
#674=(
BOUNDED_CURVE()
B_SPLINE_CURVE(2,(#37180,#37181,#37182),.UNSPECIFIED.,.F.,.F.)
B_SPLINE_CURVE_WITH_KNOTS((3,3),(-0.271795897845353,-0.218746031477168),
 .UNSPECIFIED.)
CURVE()
GEOMETRIC_REPRESENTATION_ITEM()
RATIONAL_B_SPLINE_CURVE((1.02428162962097,1.02311336089458,1.02147610369991))
REPRESENTATION_ITEM('')
);
#675=(
BOUNDED_CURVE()
B_SPLINE_CURVE(2,(#37184,#37185,#37186),.UNSPECIFIED.,.F.,.F.)
B_SPLINE_CURVE_WITH_KNOTS((3,3),(-0.589144372850594,-0.536094506482409),
 .UNSPECIFIED.)
CURVE()
GEOMETRIC_REPRESENTATION_ITEM()
RATIONAL_B_SPLINE_CURVE((1.02147610369993,1.0231133608946,1.024281629621))
REPRESENTATION_ITEM('')
);
#676=(
BOUNDED_CURVE()
B_SPLINE_CURVE(2,(#37190,#37191,#37192),.UNSPECIFIED.,.F.,.F.)
B_SPLINE_CURVE_WITH_KNOTS((3,3),(-0.271795897845345,-0.21874603147716),
 .UNSPECIFIED.)
CURVE()
GEOMETRIC_REPRESENTATION_ITEM()
RATIONAL_B_SPLINE_CURVE((1.02428162962099,1.0231133608946,1.02147610369993))
REPRESENTATION_ITEM('')
);
#677=(
BOUNDED_CURVE()
B_SPLINE_CURVE(2,(#37194,#37195,#37196),.UNSPECIFIED.,.F.,.F.)
B_SPLINE_CURVE_WITH_KNOTS((3,3),(-0.589144372850594,-0.536094506482408),
 .UNSPECIFIED.)
CURVE()
GEOMETRIC_REPRESENTATION_ITEM()
RATIONAL_B_SPLINE_CURVE((1.02147610369992,1.0231133608946,1.02428162962099))
REPRESENTATION_ITEM('')
);
#678=(
BOUNDED_CURVE()
B_SPLINE_CURVE(2,(#37200,#37201,#37202),.UNSPECIFIED.,.F.,.F.)
B_SPLINE_CURVE_WITH_KNOTS((3,3),(-0.271795897845356,-0.218746031477171),
 .UNSPECIFIED.)
CURVE()
GEOMETRIC_REPRESENTATION_ITEM()
RATIONAL_B_SPLINE_CURVE((1.02428162962096,1.02311336089457,1.0214761036999))
REPRESENTATION_ITEM('')
);
#679=(
BOUNDED_CURVE()
B_SPLINE_CURVE(2,(#37204,#37205,#37206),.UNSPECIFIED.,.F.,.F.)
B_SPLINE_CURVE_WITH_KNOTS((3,3),(-0.58914437285058,-0.536094506482397),
 .UNSPECIFIED.)
CURVE()
GEOMETRIC_REPRESENTATION_ITEM()
RATIONAL_B_SPLINE_CURVE((1.02147610369986,1.02311336089452,1.02428162962091))
REPRESENTATION_ITEM('')
);
#680=(
BOUNDED_CURVE()
B_SPLINE_CURVE(2,(#37210,#37211,#37212),.UNSPECIFIED.,.F.,.F.)
B_SPLINE_CURVE_WITH_KNOTS((3,3),(-0.271795897845352,-0.218746031477169),
 .UNSPECIFIED.)
CURVE()
GEOMETRIC_REPRESENTATION_ITEM()
RATIONAL_B_SPLINE_CURVE((1.02428162962094,1.02311336089455,1.02147610369988))
REPRESENTATION_ITEM('')
);
#681=(
BOUNDED_CURVE()
B_SPLINE_CURVE(2,(#37214,#37215,#37216),.UNSPECIFIED.,.F.,.F.)
B_SPLINE_CURVE_WITH_KNOTS((3,3),(-0.589144372850582,-0.536094506482401),
 .UNSPECIFIED.)
CURVE()
GEOMETRIC_REPRESENTATION_ITEM()
RATIONAL_B_SPLINE_CURVE((1.02147610369982,1.02311336089448,1.02428162962087))
REPRESENTATION_ITEM('')
);
#682=(
BOUNDED_CURVE()
B_SPLINE_CURVE(2,(#37220,#37221,#37222),.UNSPECIFIED.,.F.,.F.)
B_SPLINE_CURVE_WITH_KNOTS((3,3),(-0.271795897845355,-0.218746031477168),
 .UNSPECIFIED.)
CURVE()
GEOMETRIC_REPRESENTATION_ITEM()
RATIONAL_B_SPLINE_CURVE((1.02428162962102,1.02311336089462,1.02147610369995))
REPRESENTATION_ITEM('')
);
#683=(
BOUNDED_CURVE()
B_SPLINE_CURVE(2,(#37224,#37225,#37226),.UNSPECIFIED.,.F.,.F.)
B_SPLINE_CURVE_WITH_KNOTS((3,3),(-0.589144372850599,-0.536094506482414),
 .UNSPECIFIED.)
CURVE()
GEOMETRIC_REPRESENTATION_ITEM()
RATIONAL_B_SPLINE_CURVE((1.02147610369993,1.0231133608946,1.02428162962099))
REPRESENTATION_ITEM('')
);
#684=(
BOUNDED_CURVE()
B_SPLINE_CURVE(2,(#37230,#37231,#37232),.UNSPECIFIED.,.F.,.F.)
B_SPLINE_CURVE_WITH_KNOTS((3,3),(-0.271795897845353,-0.218746031477169),
 .UNSPECIFIED.)
CURVE()
GEOMETRIC_REPRESENTATION_ITEM()
RATIONAL_B_SPLINE_CURVE((1.02428162962096,1.02311336089457,1.0214761036999))
REPRESENTATION_ITEM('')
);
#685=(
BOUNDED_CURVE()
B_SPLINE_CURVE(2,(#37234,#37235,#37236),.UNSPECIFIED.,.F.,.F.)
B_SPLINE_CURVE_WITH_KNOTS((3,3),(-0.589144372850601,-0.536094506482415),
 .UNSPECIFIED.)
CURVE()
GEOMETRIC_REPRESENTATION_ITEM()
RATIONAL_B_SPLINE_CURVE((1.02147610369991,1.02311336089458,1.02428162962097))
REPRESENTATION_ITEM('')
);
#686=(
BOUNDED_CURVE()
B_SPLINE_CURVE(2,(#37240,#37241,#37242),.UNSPECIFIED.,.F.,.F.)
B_SPLINE_CURVE_WITH_KNOTS((3,3),(-0.271795897845357,-0.218746031477176),
 .UNSPECIFIED.)
CURVE()
GEOMETRIC_REPRESENTATION_ITEM()
RATIONAL_B_SPLINE_CURVE((1.02428162962087,1.02311336089448,1.02147610369982))
REPRESENTATION_ITEM('')
);
#687=(
BOUNDED_CURVE()
B_SPLINE_CURVE(2,(#37244,#37245,#37246),.UNSPECIFIED.,.F.,.F.)
B_SPLINE_CURVE_WITH_KNOTS((3,3),(-0.589144372850592,-0.536094506482409),
 .UNSPECIFIED.)
CURVE()
GEOMETRIC_REPRESENTATION_ITEM()
RATIONAL_B_SPLINE_CURVE((1.02147610369983,1.0231133608945,1.02428162962089))
REPRESENTATION_ITEM('')
);
#688=(
BOUNDED_CURVE()
B_SPLINE_CURVE(2,(#37250,#37251,#37252),.UNSPECIFIED.,.F.,.F.)
B_SPLINE_CURVE_WITH_KNOTS((3,3),(-0.271795897845353,-0.218746031477169),
 .UNSPECIFIED.)
CURVE()
GEOMETRIC_REPRESENTATION_ITEM()
RATIONAL_B_SPLINE_CURVE((1.02428162962096,1.02311336089457,1.0214761036999))
REPRESENTATION_ITEM('')
);
#689=(
BOUNDED_CURVE()
B_SPLINE_CURVE(2,(#37254,#37255,#37256),.UNSPECIFIED.,.F.,.F.)
B_SPLINE_CURVE_WITH_KNOTS((3,3),(-0.589144372850606,-0.536094506482418),
 .UNSPECIFIED.)
CURVE()
GEOMETRIC_REPRESENTATION_ITEM()
RATIONAL_B_SPLINE_CURVE((1.02147610369997,1.02311336089464,1.02428162962104))
REPRESENTATION_ITEM('')
);
#690=(
BOUNDED_CURVE()
B_SPLINE_CURVE(2,(#37260,#37261,#37262),.UNSPECIFIED.,.F.,.F.)
B_SPLINE_CURVE_WITH_KNOTS((3,3),(-0.271795897845354,-0.218746031477167),
 .UNSPECIFIED.)
CURVE()
GEOMETRIC_REPRESENTATION_ITEM()
RATIONAL_B_SPLINE_CURVE((1.02428162962102,1.02311336089463,1.02147610369995))
REPRESENTATION_ITEM('')
);
#691=(
BOUNDED_CURVE()
B_SPLINE_CURVE(2,(#37264,#37265,#37266),.UNSPECIFIED.,.F.,.F.)
B_SPLINE_CURVE_WITH_KNOTS((3,3),(-0.589144372850594,-0.536094506482407),
 .UNSPECIFIED.)
CURVE()
GEOMETRIC_REPRESENTATION_ITEM()
RATIONAL_B_SPLINE_CURVE((1.02147610369996,1.02311336089464,1.02428162962103))
REPRESENTATION_ITEM('')
);
#692=(
BOUNDED_CURVE()
B_SPLINE_CURVE(2,(#37270,#37271,#37272),.UNSPECIFIED.,.F.,.F.)
B_SPLINE_CURVE_WITH_KNOTS((3,3),(-0.271795897845348,-0.218746031477164),
 .UNSPECIFIED.)
CURVE()
GEOMETRIC_REPRESENTATION_ITEM()
RATIONAL_B_SPLINE_CURVE((1.02428162962097,1.02311336089458,1.02147610369991))
REPRESENTATION_ITEM('')
);
#693=(
BOUNDED_CURVE()
B_SPLINE_CURVE(2,(#37274,#37275,#37276),.UNSPECIFIED.,.F.,.F.)
B_SPLINE_CURVE_WITH_KNOTS((3,3),(-0.58914437285059,-0.536094506482404),
 .UNSPECIFIED.)
CURVE()
GEOMETRIC_REPRESENTATION_ITEM()
RATIONAL_B_SPLINE_CURVE((1.02147610369992,1.0231133608946,1.02428162962099))
REPRESENTATION_ITEM('')
);
#694=(
BOUNDED_CURVE()
B_SPLINE_CURVE(2,(#37280,#37281,#37282),.UNSPECIFIED.,.F.,.F.)
B_SPLINE_CURVE_WITH_KNOTS((3,3),(-0.271795897845347,-0.218746031477164),
 .UNSPECIFIED.)
CURVE()
GEOMETRIC_REPRESENTATION_ITEM()
RATIONAL_B_SPLINE_CURVE((1.02428162962094,1.02311336089455,1.02147610369988))
REPRESENTATION_ITEM('')
);
#695=(
BOUNDED_CURVE()
B_SPLINE_CURVE(2,(#37284,#37285,#37286),.UNSPECIFIED.,.F.,.F.)
B_SPLINE_CURVE_WITH_KNOTS((3,3),(-0.589144372850593,-0.536094506482406),
 .UNSPECIFIED.)
CURVE()
GEOMETRIC_REPRESENTATION_ITEM()
RATIONAL_B_SPLINE_CURVE((1.02147610369994,1.02311336089461,1.024281629621))
REPRESENTATION_ITEM('')
);
#696=(
BOUNDED_CURVE()
B_SPLINE_CURVE(2,(#37290,#37291,#37292),.UNSPECIFIED.,.F.,.F.)
B_SPLINE_CURVE_WITH_KNOTS((3,3),(-0.271795897845356,-0.218746031477165),
 .UNSPECIFIED.)
CURVE()
GEOMETRIC_REPRESENTATION_ITEM()
RATIONAL_B_SPLINE_CURVE((1.02428162962109,1.02311336089469,1.02147610370001))
REPRESENTATION_ITEM('')
);
#697=(
BOUNDED_CURVE()
B_SPLINE_CURVE(2,(#37294,#37295,#37296),.UNSPECIFIED.,.F.,.F.)
B_SPLINE_CURVE_WITH_KNOTS((3,3),(-0.589144372850608,-0.536094506482421),
 .UNSPECIFIED.)
CURVE()
GEOMETRIC_REPRESENTATION_ITEM()
RATIONAL_B_SPLINE_CURVE((1.02147610369995,1.02311336089463,1.02428162962102))
REPRESENTATION_ITEM('')
);
#698=(
BOUNDED_CURVE()
B_SPLINE_CURVE(2,(#37300,#37301,#37302),.UNSPECIFIED.,.F.,.F.)
B_SPLINE_CURVE_WITH_KNOTS((3,3),(-0.271795897845346,-0.218746031477161),
 .UNSPECIFIED.)
CURVE()
GEOMETRIC_REPRESENTATION_ITEM()
RATIONAL_B_SPLINE_CURVE((1.02428162962098,1.02311336089459,1.02147610369992))
REPRESENTATION_ITEM('')
);
#699=(
BOUNDED_CURVE()
B_SPLINE_CURVE(2,(#37304,#37305,#37306),.UNSPECIFIED.,.F.,.F.)
B_SPLINE_CURVE_WITH_KNOTS((3,3),(-0.589144372850605,-0.536094506482414),
 .UNSPECIFIED.)
CURVE()
GEOMETRIC_REPRESENTATION_ITEM()
RATIONAL_B_SPLINE_CURVE((1.02147610370001,1.02311336089469,1.02428162962109))
REPRESENTATION_ITEM('')
);
#700=(
BOUNDED_CURVE()
B_SPLINE_CURVE(2,(#37310,#37311,#37312),.UNSPECIFIED.,.F.,.F.)
B_SPLINE_CURVE_WITH_KNOTS((3,3),(-0.271795897845354,-0.218746031477166),
 .UNSPECIFIED.)
CURVE()
GEOMETRIC_REPRESENTATION_ITEM()
RATIONAL_B_SPLINE_CURVE((1.02428162962102,1.02311336089463,1.02147610369995))
REPRESENTATION_ITEM('')
);
#701=(
BOUNDED_CURVE()
B_SPLINE_CURVE(2,(#37314,#37315,#37316),.UNSPECIFIED.,.F.,.F.)
B_SPLINE_CURVE_WITH_KNOTS((3,3),(-0.589144372850611,-0.536094506482426),
 .UNSPECIFIED.)
CURVE()
GEOMETRIC_REPRESENTATION_ITEM()
RATIONAL_B_SPLINE_CURVE((1.0214761036999,1.02311336089457,1.02428162962096))
REPRESENTATION_ITEM('')
);
#702=(
BOUNDED_CURVE()
B_SPLINE_CURVE(2,(#37320,#37321,#37322),.UNSPECIFIED.,.F.,.F.)
B_SPLINE_CURVE_WITH_KNOTS((3,3),(-0.271795897845362,-0.218746031477177),
 .UNSPECIFIED.)
CURVE()
GEOMETRIC_REPRESENTATION_ITEM()
RATIONAL_B_SPLINE_CURVE((1.02428162962094,1.02311336089455,1.02147610369988))
REPRESENTATION_ITEM('')
);
#703=(
BOUNDED_CURVE()
B_SPLINE_CURVE(2,(#37324,#37325,#37326),.UNSPECIFIED.,.F.,.F.)
B_SPLINE_CURVE_WITH_KNOTS((3,3),(-0.589144372850586,-0.536094506482399),
 .UNSPECIFIED.)
CURVE()
GEOMETRIC_REPRESENTATION_ITEM()
RATIONAL_B_SPLINE_CURVE((1.02147610369992,1.0231133608946,1.02428162962099))
REPRESENTATION_ITEM('')
);
#704=(
BOUNDED_CURVE()
B_SPLINE_CURVE(2,(#37330,#37331,#37332),.UNSPECIFIED.,.F.,.F.)
B_SPLINE_CURVE_WITH_KNOTS((3,3),(-0.27179589784536,-0.218746031477171),
 .UNSPECIFIED.)
CURVE()
GEOMETRIC_REPRESENTATION_ITEM()
RATIONAL_B_SPLINE_CURVE((1.02428162962107,1.02311336089468,1.0214761037))
REPRESENTATION_ITEM('')
);
#705=(
BOUNDED_CURVE()
B_SPLINE_CURVE(2,(#37334,#37335,#37336),.UNSPECIFIED.,.F.,.F.)
B_SPLINE_CURVE_WITH_KNOTS((3,3),(-0.589144372850591,-0.536094506482411),
 .UNSPECIFIED.)
CURVE()
GEOMETRIC_REPRESENTATION_ITEM()
RATIONAL_B_SPLINE_CURVE((1.02147610369983,1.02311336089449,1.02428162962088))
REPRESENTATION_ITEM('')
);
#706=(
BOUNDED_CURVE()
B_SPLINE_CURVE(2,(#37339,#37340,#37341),.UNSPECIFIED.,.F.,.F.)
B_SPLINE_CURVE_WITH_KNOTS((3,3),(-0.271795897845348,-0.21874603147716),
 .UNSPECIFIED.)
CURVE()
GEOMETRIC_REPRESENTATION_ITEM()
RATIONAL_B_SPLINE_CURVE((1.02428162962105,1.02311336089466,1.02147610369998))
REPRESENTATION_ITEM('')
);
#707=(
BOUNDED_CURVE()
B_SPLINE_CURVE(2,(#37345,#37346,#37347),.UNSPECIFIED.,.F.,.F.)
B_SPLINE_CURVE_WITH_KNOTS((3,3),(0.536094506482406,0.589144372850591),
 .UNSPECIFIED.)
CURVE()
GEOMETRIC_REPRESENTATION_ITEM()
RATIONAL_B_SPLINE_CURVE((1.02428162962096,1.02311336089457,1.0214761036999))
REPRESENTATION_ITEM('')
);
#708=(
BOUNDED_CURVE()
B_SPLINE_CURVE(2,(#37351,#37352,#37353),.UNSPECIFIED.,.F.,.F.)
B_SPLINE_CURVE_WITH_KNOTS((3,3),(0.218746031477159,0.271795897845346),
 .UNSPECIFIED.)
CURVE()
GEOMETRIC_REPRESENTATION_ITEM()
RATIONAL_B_SPLINE_CURVE((1.02147610369995,1.02311336089463,1.02428162962102))
REPRESENTATION_ITEM('')
);
#709=(
BOUNDED_CURVE()
B_SPLINE_CURVE(2,(#37355,#37356,#37357),.UNSPECIFIED.,.F.,.F.)
B_SPLINE_CURVE_WITH_KNOTS((3,3),(0.536094506482412,0.589144372850603),
 .UNSPECIFIED.)
CURVE()
GEOMETRIC_REPRESENTATION_ITEM()
RATIONAL_B_SPLINE_CURVE((1.02428162962111,1.02311336089471,1.02147610370003))
REPRESENTATION_ITEM('')
);
#710=(
BOUNDED_CURVE()
B_SPLINE_CURVE(2,(#37361,#37362,#37363),.UNSPECIFIED.,.F.,.F.)
B_SPLINE_CURVE_WITH_KNOTS((3,3),(0.218746031477155,0.271795897845339),
 .UNSPECIFIED.)
CURVE()
GEOMETRIC_REPRESENTATION_ITEM()
RATIONAL_B_SPLINE_CURVE((1.02147610369993,1.0231133608946,1.02428162962099))
REPRESENTATION_ITEM('')
);
#711=(
BOUNDED_CURVE()
B_SPLINE_CURVE(2,(#37365,#37366,#37367),.UNSPECIFIED.,.F.,.F.)
B_SPLINE_CURVE_WITH_KNOTS((3,3),(0.536094506482406,0.589144372850597),
 .UNSPECIFIED.)
CURVE()
GEOMETRIC_REPRESENTATION_ITEM()
RATIONAL_B_SPLINE_CURVE((1.02428162962112,1.02311336089472,1.02147610370004))
REPRESENTATION_ITEM('')
);
#712=(
BOUNDED_CURVE()
B_SPLINE_CURVE(2,(#37371,#37372,#37373),.UNSPECIFIED.,.F.,.F.)
B_SPLINE_CURVE_WITH_KNOTS((3,3),(0.218746031477162,0.27179589784535),
 .UNSPECIFIED.)
CURVE()
GEOMETRIC_REPRESENTATION_ITEM()
RATIONAL_B_SPLINE_CURVE((1.02147610369998,1.02311336089466,1.02428162962105))
REPRESENTATION_ITEM('')
);
#713=(
BOUNDED_CURVE()
B_SPLINE_CURVE(2,(#37375,#37376,#37377),.UNSPECIFIED.,.F.,.F.)
B_SPLINE_CURVE_WITH_KNOTS((3,3),(0.536094506482404,0.589144372850595),
 .UNSPECIFIED.)
CURVE()
GEOMETRIC_REPRESENTATION_ITEM()
RATIONAL_B_SPLINE_CURVE((1.02428162962109,1.0231133608947,1.02147610370002))
REPRESENTATION_ITEM('')
);
#714=(
BOUNDED_CURVE()
B_SPLINE_CURVE(2,(#37381,#37382,#37383),.UNSPECIFIED.,.F.,.F.)
B_SPLINE_CURVE_WITH_KNOTS((3,3),(0.218746031477156,0.271795897845341),
 .UNSPECIFIED.)
CURVE()
GEOMETRIC_REPRESENTATION_ITEM()
RATIONAL_B_SPLINE_CURVE((1.02147610369992,1.02311336089459,1.02428162962098))
REPRESENTATION_ITEM('')
);
#715=(
BOUNDED_CURVE()
B_SPLINE_CURVE(2,(#37385,#37386,#37387),.UNSPECIFIED.,.F.,.F.)
B_SPLINE_CURVE_WITH_KNOTS((3,3),(0.536094506482416,0.589144372850602),
 .UNSPECIFIED.)
CURVE()
GEOMETRIC_REPRESENTATION_ITEM()
RATIONAL_B_SPLINE_CURVE((1.02428162962101,1.02311336089462,1.02147610369994))
REPRESENTATION_ITEM('')
);
#716=(
BOUNDED_CURVE()
B_SPLINE_CURVE(2,(#37391,#37392,#37393),.UNSPECIFIED.,.F.,.F.)
B_SPLINE_CURVE_WITH_KNOTS((3,3),(0.218746031477164,0.271795897845351),
 .UNSPECIFIED.)
CURVE()
GEOMETRIC_REPRESENTATION_ITEM()
RATIONAL_B_SPLINE_CURVE((1.02147610369995,1.02311336089463,1.02428162962102))
REPRESENTATION_ITEM('')
);
#717=(
BOUNDED_CURVE()
B_SPLINE_CURVE(2,(#37395,#37396,#37397),.UNSPECIFIED.,.F.,.F.)
B_SPLINE_CURVE_WITH_KNOTS((3,3),(0.536094506482411,0.589144372850598),
 .UNSPECIFIED.)
CURVE()
GEOMETRIC_REPRESENTATION_ITEM()
RATIONAL_B_SPLINE_CURVE((1.024281629621,1.02311336089461,1.02147610369994))
REPRESENTATION_ITEM('')
);
#718=(
BOUNDED_CURVE()
B_SPLINE_CURVE(2,(#37401,#37402,#37403),.UNSPECIFIED.,.F.,.F.)
B_SPLINE_CURVE_WITH_KNOTS((3,3),(0.218746031477161,0.271795897845348),
 .UNSPECIFIED.)
CURVE()
GEOMETRIC_REPRESENTATION_ITEM()
RATIONAL_B_SPLINE_CURVE((1.02147610369997,1.02311336089465,1.02428162962104))
REPRESENTATION_ITEM('')
);
#719=(
BOUNDED_CURVE()
B_SPLINE_CURVE(2,(#37405,#37406,#37407),.UNSPECIFIED.,.F.,.F.)
B_SPLINE_CURVE_WITH_KNOTS((3,3),(0.536094506482405,0.589144372850593),
 .UNSPECIFIED.)
CURVE()
GEOMETRIC_REPRESENTATION_ITEM()
RATIONAL_B_SPLINE_CURVE((1.02428162962104,1.02311336089464,1.02147610369997))
REPRESENTATION_ITEM('')
);
#720=(
BOUNDED_CURVE()
B_SPLINE_CURVE(2,(#37411,#37412,#37413),.UNSPECIFIED.,.F.,.F.)
B_SPLINE_CURVE_WITH_KNOTS((3,3),(0.218746031477169,0.271795897845355),
 .UNSPECIFIED.)
CURVE()
GEOMETRIC_REPRESENTATION_ITEM()
RATIONAL_B_SPLINE_CURVE((1.02147610369994,1.02311336089461,1.02428162962101))
REPRESENTATION_ITEM('')
);
#721=(
BOUNDED_CURVE()
B_SPLINE_CURVE(2,(#37415,#37416,#37417),.UNSPECIFIED.,.F.,.F.)
B_SPLINE_CURVE_WITH_KNOTS((3,3),(0.536094506482416,0.589144372850604),
 .UNSPECIFIED.)
CURVE()
GEOMETRIC_REPRESENTATION_ITEM()
RATIONAL_B_SPLINE_CURVE((1.02428162962105,1.02311336089466,1.02147610369998))
REPRESENTATION_ITEM('')
);
#722=(
BOUNDED_CURVE()
B_SPLINE_CURVE(2,(#37421,#37422,#37423),.UNSPECIFIED.,.F.,.F.)
B_SPLINE_CURVE_WITH_KNOTS((3,3),(0.218746031477159,0.271795897845341),
 .UNSPECIFIED.)
CURVE()
GEOMETRIC_REPRESENTATION_ITEM()
RATIONAL_B_SPLINE_CURVE((1.02147610369987,1.02311336089454,1.02428162962093))
REPRESENTATION_ITEM('')
);
#723=(
BOUNDED_CURVE()
B_SPLINE_CURVE(2,(#37425,#37426,#37427),.UNSPECIFIED.,.F.,.F.)
B_SPLINE_CURVE_WITH_KNOTS((3,3),(0.536094506482407,0.589144372850592),
 .UNSPECIFIED.)
CURVE()
GEOMETRIC_REPRESENTATION_ITEM()
RATIONAL_B_SPLINE_CURVE((1.02428162962098,1.02311336089459,1.02147610369991))
REPRESENTATION_ITEM('')
);
#724=(
BOUNDED_CURVE()
B_SPLINE_CURVE(2,(#37431,#37432,#37433),.UNSPECIFIED.,.F.,.F.)
B_SPLINE_CURVE_WITH_KNOTS((3,3),(0.218746031477156,0.271795897845344),
 .UNSPECIFIED.)
CURVE()
GEOMETRIC_REPRESENTATION_ITEM()
RATIONAL_B_SPLINE_CURVE((1.02147610369997,1.02311336089464,1.02428162962104))
REPRESENTATION_ITEM('')
);
#725=(
BOUNDED_CURVE()
B_SPLINE_CURVE(2,(#37435,#37436,#37437),.UNSPECIFIED.,.F.,.F.)
B_SPLINE_CURVE_WITH_KNOTS((3,3),(0.536094506482407,0.589144372850596),
 .UNSPECIFIED.)
CURVE()
GEOMETRIC_REPRESENTATION_ITEM()
RATIONAL_B_SPLINE_CURVE((1.02428162962105,1.02311336089465,1.02147610369998))
REPRESENTATION_ITEM('')
);
#726=(
BOUNDED_CURVE()
B_SPLINE_CURVE(2,(#37441,#37442,#37443),.UNSPECIFIED.,.F.,.F.)
B_SPLINE_CURVE_WITH_KNOTS((3,3),(0.218746031477169,0.271795897845356),
 .UNSPECIFIED.)
CURVE()
GEOMETRIC_REPRESENTATION_ITEM()
RATIONAL_B_SPLINE_CURVE((1.02147610369994,1.02311336089461,1.024281629621))
REPRESENTATION_ITEM('')
);
#727=(
BOUNDED_CURVE()
B_SPLINE_CURVE(2,(#37445,#37446,#37447),.UNSPECIFIED.,.F.,.F.)
B_SPLINE_CURVE_WITH_KNOTS((3,3),(0.536094506482405,0.589144372850591),
 .UNSPECIFIED.)
CURVE()
GEOMETRIC_REPRESENTATION_ITEM()
RATIONAL_B_SPLINE_CURVE((1.02428162962096,1.02311336089457,1.0214761036999))
REPRESENTATION_ITEM('')
);
#728=(
BOUNDED_CURVE()
B_SPLINE_CURVE(2,(#37451,#37452,#37453),.UNSPECIFIED.,.F.,.F.)
B_SPLINE_CURVE_WITH_KNOTS((3,3),(0.21874603147717,0.271795897845356),
 .UNSPECIFIED.)
CURVE()
GEOMETRIC_REPRESENTATION_ITEM()
RATIONAL_B_SPLINE_CURVE((1.02147610369993,1.0231133608946,1.02428162962099))
REPRESENTATION_ITEM('')
);
#729=(
BOUNDED_CURVE()
B_SPLINE_CURVE(2,(#37455,#37456,#37457),.UNSPECIFIED.,.F.,.F.)
B_SPLINE_CURVE_WITH_KNOTS((3,3),(0.536094506482407,0.589144372850593),
 .UNSPECIFIED.)
CURVE()
GEOMETRIC_REPRESENTATION_ITEM()
RATIONAL_B_SPLINE_CURVE((1.02428162962098,1.02311336089459,1.02147610369992))
REPRESENTATION_ITEM('')
);
#730=(
BOUNDED_CURVE()
B_SPLINE_CURVE(2,(#37461,#37462,#37463),.UNSPECIFIED.,.F.,.F.)
B_SPLINE_CURVE_WITH_KNOTS((3,3),(0.218746031477165,0.271795897845348),
 .UNSPECIFIED.)
CURVE()
GEOMETRIC_REPRESENTATION_ITEM()
RATIONAL_B_SPLINE_CURVE((1.02147610369988,1.02311336089455,1.02428162962093))
REPRESENTATION_ITEM('')
);
#731=(
BOUNDED_CURVE()
B_SPLINE_CURVE(2,(#37465,#37466,#37467),.UNSPECIFIED.,.F.,.F.)
B_SPLINE_CURVE_WITH_KNOTS((3,3),(0.53609450648242,0.589144372850606),
 .UNSPECIFIED.)
CURVE()
GEOMETRIC_REPRESENTATION_ITEM()
RATIONAL_B_SPLINE_CURVE((1.024281629621,1.02311336089461,1.02147610369994))
REPRESENTATION_ITEM('')
);
#732=(
BOUNDED_CURVE()
B_SPLINE_CURVE(2,(#37471,#37472,#37473),.UNSPECIFIED.,.F.,.F.)
B_SPLINE_CURVE_WITH_KNOTS((3,3),(0.218746031477168,0.271795897845355),
 .UNSPECIFIED.)
CURVE()
GEOMETRIC_REPRESENTATION_ITEM()
RATIONAL_B_SPLINE_CURVE((1.02147610369993,1.02311336089461,1.024281629621))
REPRESENTATION_ITEM('')
);
#733=(
BOUNDED_CURVE()
B_SPLINE_CURVE(2,(#37475,#37476,#37477),.UNSPECIFIED.,.F.,.F.)
B_SPLINE_CURVE_WITH_KNOTS((3,3),(0.536094506482407,0.589144372850592),
 .UNSPECIFIED.)
CURVE()
GEOMETRIC_REPRESENTATION_ITEM()
RATIONAL_B_SPLINE_CURVE((1.02428162962095,1.02311336089456,1.02147610369989))
REPRESENTATION_ITEM('')
);
#734=(
BOUNDED_CURVE()
B_SPLINE_CURVE(2,(#37481,#37482,#37483),.UNSPECIFIED.,.F.,.F.)
B_SPLINE_CURVE_WITH_KNOTS((3,3),(0.218746031477166,0.271795897845353),
 .UNSPECIFIED.)
CURVE()
GEOMETRIC_REPRESENTATION_ITEM()
RATIONAL_B_SPLINE_CURVE((1.02147610369992,1.0231133608946,1.02428162962099))
REPRESENTATION_ITEM('')
);
#735=(
BOUNDED_CURVE()
B_SPLINE_CURVE(2,(#37485,#37486,#37487),.UNSPECIFIED.,.F.,.F.)
B_SPLINE_CURVE_WITH_KNOTS((3,3),(0.536094506482401,0.589144372850589),
 .UNSPECIFIED.)
CURVE()
GEOMETRIC_REPRESENTATION_ITEM()
RATIONAL_B_SPLINE_CURVE((1.02428162962102,1.02311336089463,1.02147610369996))
REPRESENTATION_ITEM('')
);
#736=(
BOUNDED_CURVE()
B_SPLINE_CURVE(2,(#37491,#37492,#37493),.UNSPECIFIED.,.F.,.F.)
B_SPLINE_CURVE_WITH_KNOTS((3,3),(0.218746031477163,0.271795897845347),
 .UNSPECIFIED.)
CURVE()
GEOMETRIC_REPRESENTATION_ITEM()
RATIONAL_B_SPLINE_CURVE((1.0214761036999,1.02311336089457,1.02428162962096))
REPRESENTATION_ITEM('')
);
#737=(
BOUNDED_CURVE()
B_SPLINE_CURVE(2,(#37495,#37496,#37497),.UNSPECIFIED.,.F.,.F.)
B_SPLINE_CURVE_WITH_KNOTS((3,3),(0.536094506482403,0.58914437285059),
 .UNSPECIFIED.)
CURVE()
GEOMETRIC_REPRESENTATION_ITEM()
RATIONAL_B_SPLINE_CURVE((1.02428162962101,1.02311336089462,1.02147610369994))
REPRESENTATION_ITEM('')
);
#738=(
BOUNDED_CURVE()
B_SPLINE_CURVE(2,(#37501,#37502,#37503),.UNSPECIFIED.,.F.,.F.)
B_SPLINE_CURVE_WITH_KNOTS((3,3),(0.218746031477163,0.271795897845349),
 .UNSPECIFIED.)
CURVE()
GEOMETRIC_REPRESENTATION_ITEM()
RATIONAL_B_SPLINE_CURVE((1.02147610369993,1.02311336089461,1.024281629621))
REPRESENTATION_ITEM('')
);
#739=(
BOUNDED_CURVE()
B_SPLINE_CURVE(2,(#37505,#37506,#37507),.UNSPECIFIED.,.F.,.F.)
B_SPLINE_CURVE_WITH_KNOTS((3,3),(0.536094506482407,0.589144372850591),
 .UNSPECIFIED.)
CURVE()
GEOMETRIC_REPRESENTATION_ITEM()
RATIONAL_B_SPLINE_CURVE((1.02428162962096,1.02311336089457,1.0214761036999))
REPRESENTATION_ITEM('')
);
#740=(
BOUNDED_CURVE()
B_SPLINE_CURVE(2,(#37511,#37512,#37513),.UNSPECIFIED.,.F.,.F.)
B_SPLINE_CURVE_WITH_KNOTS((3,3),(0.218746031477169,0.271795897845354),
 .UNSPECIFIED.)
CURVE()
GEOMETRIC_REPRESENTATION_ITEM()
RATIONAL_B_SPLINE_CURVE((1.0214761036999,1.02311336089457,1.02428162962096))
REPRESENTATION_ITEM('')
);
#741=(
BOUNDED_CURVE()
B_SPLINE_CURVE(2,(#37515,#37516,#37517),.UNSPECIFIED.,.F.,.F.)
B_SPLINE_CURVE_WITH_KNOTS((3,3),(0.536094506482406,0.589144372850594),
 .UNSPECIFIED.)
CURVE()
GEOMETRIC_REPRESENTATION_ITEM()
RATIONAL_B_SPLINE_CURVE((1.02428162962102,1.02311336089463,1.02147610369995))
REPRESENTATION_ITEM('')
);
#742=(
BOUNDED_CURVE()
B_SPLINE_CURVE(2,(#37521,#37522,#37523),.UNSPECIFIED.,.F.,.F.)
B_SPLINE_CURVE_WITH_KNOTS((3,3),(0.218746031477168,0.271795897845353),
 .UNSPECIFIED.)
CURVE()
GEOMETRIC_REPRESENTATION_ITEM()
RATIONAL_B_SPLINE_CURVE((1.02147610369991,1.02311336089458,1.02428162962097))
REPRESENTATION_ITEM('')
);
#743=(
BOUNDED_CURVE()
B_SPLINE_CURVE(2,(#37525,#37526,#37527),.UNSPECIFIED.,.F.,.F.)
B_SPLINE_CURVE_WITH_KNOTS((3,3),(0.536094506482413,0.589144372850603),
 .UNSPECIFIED.)
CURVE()
GEOMETRIC_REPRESENTATION_ITEM()
RATIONAL_B_SPLINE_CURVE((1.02428162962108,1.02311336089468,1.0214761037))
REPRESENTATION_ITEM('')
);
#744=(
BOUNDED_CURVE()
B_SPLINE_CURVE(2,(#37531,#37532,#37533),.UNSPECIFIED.,.F.,.F.)
B_SPLINE_CURVE_WITH_KNOTS((3,3),(0.218746031477166,0.27179589784535),
 .UNSPECIFIED.)
CURVE()
GEOMETRIC_REPRESENTATION_ITEM()
RATIONAL_B_SPLINE_CURVE((1.02147610369991,1.02311336089458,1.02428162962097))
REPRESENTATION_ITEM('')
);
#745=(
BOUNDED_CURVE()
B_SPLINE_CURVE(2,(#37535,#37536,#37537),.UNSPECIFIED.,.F.,.F.)
B_SPLINE_CURVE_WITH_KNOTS((3,3),(0.536094506482411,0.589144372850594),
 .UNSPECIFIED.)
CURVE()
GEOMETRIC_REPRESENTATION_ITEM()
RATIONAL_B_SPLINE_CURVE((1.02428162962096,1.02311336089457,1.0214761036999))
REPRESENTATION_ITEM('')
);
#746=(
BOUNDED_CURVE()
B_SPLINE_CURVE(2,(#37541,#37542,#37543),.UNSPECIFIED.,.F.,.F.)
B_SPLINE_CURVE_WITH_KNOTS((3,3),(0.218746031477168,0.271795897845354),
 .UNSPECIFIED.)
CURVE()
GEOMETRIC_REPRESENTATION_ITEM()
RATIONAL_B_SPLINE_CURVE((1.02147610369994,1.02311336089461,1.024281629621))
REPRESENTATION_ITEM('')
);
#747=(
BOUNDED_CURVE()
B_SPLINE_CURVE(2,(#37545,#37546,#37547),.UNSPECIFIED.,.F.,.F.)
B_SPLINE_CURVE_WITH_KNOTS((3,3),(0.536094506482396,0.589144372850584),
 .UNSPECIFIED.)
CURVE()
GEOMETRIC_REPRESENTATION_ITEM()
RATIONAL_B_SPLINE_CURVE((1.02428162962101,1.02311336089462,1.02147610369994))
REPRESENTATION_ITEM('')
);
#748=(
BOUNDED_CURVE()
B_SPLINE_CURVE(2,(#37551,#37552,#37553),.UNSPECIFIED.,.F.,.F.)
B_SPLINE_CURVE_WITH_KNOTS((3,3),(0.21874603147717,0.271795897845356),
 .UNSPECIFIED.)
CURVE()
GEOMETRIC_REPRESENTATION_ITEM()
RATIONAL_B_SPLINE_CURVE((1.02147610369993,1.0231133608946,1.024281629621))
REPRESENTATION_ITEM('')
);
#749=(
BOUNDED_CURVE()
B_SPLINE_CURVE(2,(#37555,#37556,#37557),.UNSPECIFIED.,.F.,.F.)
B_SPLINE_CURVE_WITH_KNOTS((3,3),(0.536094506482412,0.589144372850595),
 .UNSPECIFIED.)
CURVE()
GEOMETRIC_REPRESENTATION_ITEM()
RATIONAL_B_SPLINE_CURVE((1.02428162962094,1.02311336089456,1.02147610369989))
REPRESENTATION_ITEM('')
);
#750=(
BOUNDED_CURVE()
B_SPLINE_CURVE(2,(#37561,#37562,#37563),.UNSPECIFIED.,.F.,.F.)
B_SPLINE_CURVE_WITH_KNOTS((3,3),(0.218746031477162,0.271795897845349),
 .UNSPECIFIED.)
CURVE()
GEOMETRIC_REPRESENTATION_ITEM()
RATIONAL_B_SPLINE_CURVE((1.02147610369997,1.02311336089465,1.02428162962104))
REPRESENTATION_ITEM('')
);
#751=(
BOUNDED_CURVE()
B_SPLINE_CURVE(2,(#37565,#37566,#37567),.UNSPECIFIED.,.F.,.F.)
B_SPLINE_CURVE_WITH_KNOTS((3,3),(0.536094506482409,0.589144372850593),
 .UNSPECIFIED.)
CURVE()
GEOMETRIC_REPRESENTATION_ITEM()
RATIONAL_B_SPLINE_CURVE((1.02428162962095,1.02311336089457,1.02147610369989))
REPRESENTATION_ITEM('')
);
#752=(
BOUNDED_CURVE()
B_SPLINE_CURVE(2,(#37571,#37572,#37573),.UNSPECIFIED.,.F.,.F.)
B_SPLINE_CURVE_WITH_KNOTS((3,3),(0.218746031477157,0.271795897845344),
 .UNSPECIFIED.)
CURVE()
GEOMETRIC_REPRESENTATION_ITEM()
RATIONAL_B_SPLINE_CURVE((1.02147610369996,1.02311336089464,1.02428162962103))
REPRESENTATION_ITEM('')
);
#753=(
BOUNDED_CURVE()
B_SPLINE_CURVE(2,(#37575,#37576,#37577),.UNSPECIFIED.,.F.,.F.)
B_SPLINE_CURVE_WITH_KNOTS((3,3),(0.536094506482406,0.589144372850595),
 .UNSPECIFIED.)
CURVE()
GEOMETRIC_REPRESENTATION_ITEM()
RATIONAL_B_SPLINE_CURVE((1.02428162962104,1.02311336089464,1.02147610369997))
REPRESENTATION_ITEM('')
);
#754=(
BOUNDED_CURVE()
B_SPLINE_CURVE(2,(#37581,#37582,#37583),.UNSPECIFIED.,.F.,.F.)
B_SPLINE_CURVE_WITH_KNOTS((3,3),(0.21874603147716,0.271795897845345),
 .UNSPECIFIED.)
CURVE()
GEOMETRIC_REPRESENTATION_ITEM()
RATIONAL_B_SPLINE_CURVE((1.02147610369992,1.02311336089459,1.02428162962098))
REPRESENTATION_ITEM('')
);
#755=(
BOUNDED_CURVE()
B_SPLINE_CURVE(2,(#37585,#37586,#37587),.UNSPECIFIED.,.F.,.F.)
B_SPLINE_CURVE_WITH_KNOTS((3,3),(0.536094506482396,0.589144372850584),
 .UNSPECIFIED.)
CURVE()
GEOMETRIC_REPRESENTATION_ITEM()
RATIONAL_B_SPLINE_CURVE((1.024281629621,1.02311336089461,1.02147610369993))
REPRESENTATION_ITEM('')
);
#756=(
BOUNDED_CURVE()
B_SPLINE_CURVE(2,(#37591,#37592,#37593),.UNSPECIFIED.,.F.,.F.)
B_SPLINE_CURVE_WITH_KNOTS((3,3),(0.218746031477161,0.271795897845347),
 .UNSPECIFIED.)
CURVE()
GEOMETRIC_REPRESENTATION_ITEM()
RATIONAL_B_SPLINE_CURVE((1.02147610369993,1.02311336089461,1.024281629621))
REPRESENTATION_ITEM('')
);
#757=(
BOUNDED_CURVE()
B_SPLINE_CURVE(2,(#37595,#37596,#37597),.UNSPECIFIED.,.F.,.F.)
B_SPLINE_CURVE_WITH_KNOTS((3,3),(0.536094506482403,0.58914437285059),
 .UNSPECIFIED.)
CURVE()
GEOMETRIC_REPRESENTATION_ITEM()
RATIONAL_B_SPLINE_CURVE((1.02428162962099,1.0231133608946,1.02147610369993))
REPRESENTATION_ITEM('')
);
#758=(
BOUNDED_CURVE()
B_SPLINE_CURVE(2,(#37601,#37602,#37603),.UNSPECIFIED.,.F.,.F.)
B_SPLINE_CURVE_WITH_KNOTS((3,3),(0.218746031477149,0.271795897845334),
 .UNSPECIFIED.)
CURVE()
GEOMETRIC_REPRESENTATION_ITEM()
RATIONAL_B_SPLINE_CURVE((1.02147610369993,1.0231133608946,1.02428162962099))
REPRESENTATION_ITEM('')
);
#759=(
BOUNDED_CURVE()
B_SPLINE_CURVE(2,(#37605,#37606,#37607),.UNSPECIFIED.,.F.,.F.)
B_SPLINE_CURVE_WITH_KNOTS((3,3),(0.536094506482409,0.589144372850597),
 .UNSPECIFIED.)
CURVE()
GEOMETRIC_REPRESENTATION_ITEM()
RATIONAL_B_SPLINE_CURVE((1.02428162962102,1.02311336089463,1.02147610369995))
REPRESENTATION_ITEM('')
);
#760=(
BOUNDED_CURVE()
B_SPLINE_CURVE(2,(#37611,#37612,#37613),.UNSPECIFIED.,.F.,.F.)
B_SPLINE_CURVE_WITH_KNOTS((3,3),(0.218746031477158,0.271795897845347),
 .UNSPECIFIED.)
CURVE()
GEOMETRIC_REPRESENTATION_ITEM()
RATIONAL_B_SPLINE_CURVE((1.02147610370001,1.02311336089469,1.02428162962108))
REPRESENTATION_ITEM('')
);
#761=(
BOUNDED_CURVE()
B_SPLINE_CURVE(2,(#37615,#37616,#37617),.UNSPECIFIED.,.F.,.F.)
B_SPLINE_CURVE_WITH_KNOTS((3,3),(0.536094506482415,0.589144372850599),
 .UNSPECIFIED.)
CURVE()
GEOMETRIC_REPRESENTATION_ITEM()
RATIONAL_B_SPLINE_CURVE((1.02428162962096,1.02311336089458,1.0214761036999))
REPRESENTATION_ITEM('')
);
#762=(
BOUNDED_CURVE()
B_SPLINE_CURVE(2,(#37621,#37622,#37623),.UNSPECIFIED.,.F.,.F.)
B_SPLINE_CURVE_WITH_KNOTS((3,3),(0.218746031477152,0.271795897845339),
 .UNSPECIFIED.)
CURVE()
GEOMETRIC_REPRESENTATION_ITEM()
RATIONAL_B_SPLINE_CURVE((1.02147610369995,1.02311336089463,1.02428162962102))
REPRESENTATION_ITEM('')
);
#763=(
BOUNDED_CURVE()
B_SPLINE_CURVE(2,(#37625,#37626,#37627),.UNSPECIFIED.,.F.,.F.)
B_SPLINE_CURVE_WITH_KNOTS((3,3),(0.536094506482415,0.589144372850599),
 .UNSPECIFIED.)
CURVE()
GEOMETRIC_REPRESENTATION_ITEM()
RATIONAL_B_SPLINE_CURVE((1.02428162962096,1.02311336089457,1.0214761036999))
REPRESENTATION_ITEM('')
);
#764=(
BOUNDED_CURVE()
B_SPLINE_CURVE(2,(#37631,#37632,#37633),.UNSPECIFIED.,.F.,.F.)
B_SPLINE_CURVE_WITH_KNOTS((3,3),(0.218746031477149,0.271795897845338),
 .UNSPECIFIED.)
CURVE()
GEOMETRIC_REPRESENTATION_ITEM()
RATIONAL_B_SPLINE_CURVE((1.02147610370001,1.02311336089469,1.02428162962109))
REPRESENTATION_ITEM('')
);
#765=(
BOUNDED_CURVE()
B_SPLINE_CURVE(2,(#37635,#37636,#37637),.UNSPECIFIED.,.F.,.F.)
B_SPLINE_CURVE_WITH_KNOTS((3,3),(0.536094506482408,0.589144372850593),
 .UNSPECIFIED.)
CURVE()
GEOMETRIC_REPRESENTATION_ITEM()
RATIONAL_B_SPLINE_CURVE((1.02428162962098,1.02311336089459,1.02147610369992))
REPRESENTATION_ITEM('')
);
#766=(
BOUNDED_CURVE()
B_SPLINE_CURVE(2,(#37641,#37642,#37643),.UNSPECIFIED.,.F.,.F.)
B_SPLINE_CURVE_WITH_KNOTS((3,3),(0.218746031477164,0.271795897845349),
 .UNSPECIFIED.)
CURVE()
GEOMETRIC_REPRESENTATION_ITEM()
RATIONAL_B_SPLINE_CURVE((1.02147610369991,1.02311336089459,1.02428162962098))
REPRESENTATION_ITEM('')
);
#767=(
BOUNDED_CURVE()
B_SPLINE_CURVE(2,(#37645,#37646,#37647),.UNSPECIFIED.,.F.,.F.)
B_SPLINE_CURVE_WITH_KNOTS((3,3),(0.536094506482405,0.589144372850592),
 .UNSPECIFIED.)
CURVE()
GEOMETRIC_REPRESENTATION_ITEM()
RATIONAL_B_SPLINE_CURVE((1.02428162962101,1.02311336089462,1.02147610369994))
REPRESENTATION_ITEM('')
);
#768=(
BOUNDED_CURVE()
B_SPLINE_CURVE(2,(#37651,#37652,#37653),.UNSPECIFIED.,.F.,.F.)
B_SPLINE_CURVE_WITH_KNOTS((3,3),(0.218746031477147,0.271795897845335),
 .UNSPECIFIED.)
CURVE()
GEOMETRIC_REPRESENTATION_ITEM()
RATIONAL_B_SPLINE_CURVE((1.02147610369998,1.02311336089466,1.02428162962105))
REPRESENTATION_ITEM('')
);
#769=(
BOUNDED_CURVE()
B_SPLINE_CURVE(2,(#37655,#37656,#37657),.UNSPECIFIED.,.F.,.F.)
B_SPLINE_CURVE_WITH_KNOTS((3,3),(0.536094506482405,0.589144372850589),
 .UNSPECIFIED.)
CURVE()
GEOMETRIC_REPRESENTATION_ITEM()
RATIONAL_B_SPLINE_CURVE((1.02428162962092,1.02311336089453,1.02147610369986))
REPRESENTATION_ITEM('')
);
#770=(
BOUNDED_CURVE()
B_SPLINE_CURVE(2,(#37661,#37662,#37663),.UNSPECIFIED.,.F.,.F.)
B_SPLINE_CURVE_WITH_KNOTS((3,3),(0.218746031477157,0.271795897845349),
 .UNSPECIFIED.)
CURVE()
GEOMETRIC_REPRESENTATION_ITEM()
RATIONAL_B_SPLINE_CURVE((1.02147610370005,1.02311336089473,1.02428162962113))
REPRESENTATION_ITEM('')
);
#771=(
BOUNDED_CURVE()
B_SPLINE_CURVE(2,(#37665,#37666,#37667),.UNSPECIFIED.,.F.,.F.)
B_SPLINE_CURVE_WITH_KNOTS((3,3),(0.536094506482405,0.589144372850593),
 .UNSPECIFIED.)
CURVE()
GEOMETRIC_REPRESENTATION_ITEM()
RATIONAL_B_SPLINE_CURVE((1.02428162962104,1.02311336089464,1.02147610369997))
REPRESENTATION_ITEM('')
);
#772=(
BOUNDED_CURVE()
B_SPLINE_CURVE(2,(#37671,#37672,#37673),.UNSPECIFIED.,.F.,.F.)
B_SPLINE_CURVE_WITH_KNOTS((3,3),(0.218746031477155,0.271795897845342),
 .UNSPECIFIED.)
CURVE()
GEOMETRIC_REPRESENTATION_ITEM()
RATIONAL_B_SPLINE_CURVE((1.02147610369998,1.02311336089466,1.02428162962105))
REPRESENTATION_ITEM('')
);
#773=(
BOUNDED_CURVE()
B_SPLINE_CURVE(2,(#37675,#37676,#37677),.UNSPECIFIED.,.F.,.F.)
B_SPLINE_CURVE_WITH_KNOTS((3,3),(0.536094506482402,0.589144372850587),
 .UNSPECIFIED.)
CURVE()
GEOMETRIC_REPRESENTATION_ITEM()
RATIONAL_B_SPLINE_CURVE((1.02428162962096,1.02311336089458,1.0214761036999))
REPRESENTATION_ITEM('')
);
#774=(
BOUNDED_CURVE()
B_SPLINE_CURVE(2,(#37681,#37682,#37683),.UNSPECIFIED.,.F.,.F.)
B_SPLINE_CURVE_WITH_KNOTS((3,3),(0.218746031477152,0.271795897845337),
 .UNSPECIFIED.)
CURVE()
GEOMETRIC_REPRESENTATION_ITEM()
RATIONAL_B_SPLINE_CURVE((1.02147610369994,1.02311336089462,1.02428162962101))
REPRESENTATION_ITEM('')
);
#775=(
BOUNDED_CURVE()
B_SPLINE_CURVE(2,(#37685,#37686,#37687),.UNSPECIFIED.,.F.,.F.)
B_SPLINE_CURVE_WITH_KNOTS((3,3),(0.536094506482403,0.58914437285059),
 .UNSPECIFIED.)
CURVE()
GEOMETRIC_REPRESENTATION_ITEM()
RATIONAL_B_SPLINE_CURVE((1.024281629621,1.02311336089461,1.02147610369994))
REPRESENTATION_ITEM('')
);
#776=(
BOUNDED_CURVE()
B_SPLINE_CURVE(2,(#37691,#37692,#37693),.UNSPECIFIED.,.F.,.F.)
B_SPLINE_CURVE_WITH_KNOTS((3,3),(0.218746031477151,0.271795897845343),
 .UNSPECIFIED.)
CURVE()
GEOMETRIC_REPRESENTATION_ITEM()
RATIONAL_B_SPLINE_CURVE((1.02147610370007,1.02311336089475,1.02428162962115))
REPRESENTATION_ITEM('')
);
#777=(
BOUNDED_CURVE()
B_SPLINE_CURVE(2,(#37695,#37696,#37697),.UNSPECIFIED.,.F.,.F.)
B_SPLINE_CURVE_WITH_KNOTS((3,3),(0.536094506482409,0.589144372850593),
 .UNSPECIFIED.)
CURVE()
GEOMETRIC_REPRESENTATION_ITEM()
RATIONAL_B_SPLINE_CURVE((1.02428162962094,1.02311336089455,1.02147610369988))
REPRESENTATION_ITEM('')
);
#778=(
BOUNDED_CURVE()
B_SPLINE_CURVE(2,(#37701,#37702,#37703),.UNSPECIFIED.,.F.,.F.)
B_SPLINE_CURVE_WITH_KNOTS((3,3),(0.218746031477156,0.271795897845345),
 .UNSPECIFIED.)
CURVE()
GEOMETRIC_REPRESENTATION_ITEM()
RATIONAL_B_SPLINE_CURVE((1.02147610370001,1.02311336089469,1.02428162962108))
REPRESENTATION_ITEM('')
);
#779=(
BOUNDED_CURVE()
B_SPLINE_CURVE(2,(#37705,#37706,#37707),.UNSPECIFIED.,.F.,.F.)
B_SPLINE_CURVE_WITH_KNOTS((3,3),(0.536094506482414,0.589144372850603),
 .UNSPECIFIED.)
CURVE()
GEOMETRIC_REPRESENTATION_ITEM()
RATIONAL_B_SPLINE_CURVE((1.02428162962107,1.02311336089467,1.02147610369999))
REPRESENTATION_ITEM('')
);
#780=(
BOUNDED_CURVE()
B_SPLINE_CURVE(2,(#37711,#37712,#37713),.UNSPECIFIED.,.F.,.F.)
B_SPLINE_CURVE_WITH_KNOTS((3,3),(0.218746031477163,0.271795897845352),
 .UNSPECIFIED.)
CURVE()
GEOMETRIC_REPRESENTATION_ITEM()
RATIONAL_B_SPLINE_CURVE((1.02147610369999,1.02311336089467,1.02428162962106))
REPRESENTATION_ITEM('')
);
#781=(
BOUNDED_CURVE()
B_SPLINE_CURVE(2,(#37715,#37716,#37717),.UNSPECIFIED.,.F.,.F.)
B_SPLINE_CURVE_WITH_KNOTS((3,3),(0.536094506482405,0.58914437285059),
 .UNSPECIFIED.)
CURVE()
GEOMETRIC_REPRESENTATION_ITEM()
RATIONAL_B_SPLINE_CURVE((1.02428162962097,1.02311336089458,1.02147610369991))
REPRESENTATION_ITEM('')
);
#782=(
BOUNDED_CURVE()
B_SPLINE_CURVE(2,(#37721,#37722,#37723),.UNSPECIFIED.,.F.,.F.)
B_SPLINE_CURVE_WITH_KNOTS((3,3),(0.218746031477157,0.27179589784534),
 .UNSPECIFIED.)
CURVE()
GEOMETRIC_REPRESENTATION_ITEM()
RATIONAL_B_SPLINE_CURVE((1.02147610369987,1.02311336089454,1.02428162962093))
REPRESENTATION_ITEM('')
);
#783=(
BOUNDED_CURVE()
B_SPLINE_CURVE(2,(#37725,#37726,#37727),.UNSPECIFIED.,.F.,.F.)
B_SPLINE_CURVE_WITH_KNOTS((3,3),(0.536094506482407,0.589144372850599),
 .UNSPECIFIED.)
CURVE()
GEOMETRIC_REPRESENTATION_ITEM()
RATIONAL_B_SPLINE_CURVE((1.02428162962112,1.02311336089472,1.02147610370004))
REPRESENTATION_ITEM('')
);
#784=(
BOUNDED_CURVE()
B_SPLINE_CURVE(2,(#37731,#37732,#37733),.UNSPECIFIED.,.F.,.F.)
B_SPLINE_CURVE_WITH_KNOTS((3,3),(-0.271795897845351,-0.270098893534586),
 .UNSPECIFIED.)
CURVE()
GEOMETRIC_REPRESENTATION_ITEM()
RATIONAL_B_SPLINE_CURVE((1.02428162962102,1.02424425804592,1.02420640656119))
REPRESENTATION_ITEM('')
);
#785=(
BOUNDED_CURVE()
B_SPLINE_CURVE(2,(#37738,#37739,#37740),.UNSPECIFIED.,.F.,.F.)
B_SPLINE_CURVE_WITH_KNOTS((3,3),(-0.270098893534586,-0.218746031477164),
 .UNSPECIFIED.)
CURVE()
GEOMETRIC_REPRESENTATION_ITEM()
RATIONAL_B_SPLINE_CURVE((1.02420640656119,1.02306098691695,1.02147610369995))
REPRESENTATION_ITEM('')
);
#786=(
BOUNDED_CURVE()
B_SPLINE_CURVE(2,(#37742,#37743,#37744),.UNSPECIFIED.,.F.,.F.)
B_SPLINE_CURVE_WITH_KNOTS((3,3),(0.536094506482404,0.589144372850591),
 .UNSPECIFIED.)
CURVE()
GEOMETRIC_REPRESENTATION_ITEM()
RATIONAL_B_SPLINE_CURVE((1.02428162962101,1.02311336089462,1.02147610369994))
REPRESENTATION_ITEM('')
);
#787=(
BOUNDED_CURVE()
B_SPLINE_CURVE(2,(#37748,#37749,#37750),.UNSPECIFIED.,.F.,.F.)
B_SPLINE_CURVE_WITH_KNOTS((3,3),(0.218746031477165,0.271795897845351),
 .UNSPECIFIED.)
CURVE()
GEOMETRIC_REPRESENTATION_ITEM()
RATIONAL_B_SPLINE_CURVE((1.02147610369995,1.02311336089462,1.02428162962101))
REPRESENTATION_ITEM('')
);
#788=(
BOUNDED_CURVE()
B_SPLINE_CURVE(2,(#37752,#37753,#37754),.UNSPECIFIED.,.F.,.F.)
B_SPLINE_CURVE_WITH_KNOTS((3,3),(0.536094506482406,0.589144372850597),
 .UNSPECIFIED.)
CURVE()
GEOMETRIC_REPRESENTATION_ITEM()
RATIONAL_B_SPLINE_CURVE((1.02428162962109,1.02311336089469,1.02147610370001))
REPRESENTATION_ITEM('')
);
#789=(
BOUNDED_CURVE()
B_SPLINE_CURVE(2,(#37758,#37759,#37760),.UNSPECIFIED.,.F.,.F.)
B_SPLINE_CURVE_WITH_KNOTS((3,3),(0.218746031477132,0.271795897845324),
 .UNSPECIFIED.)
CURVE()
GEOMETRIC_REPRESENTATION_ITEM()
RATIONAL_B_SPLINE_CURVE((1.02147610370008,1.02311336089477,1.02428162962117))
REPRESENTATION_ITEM('')
);
#790=(
BOUNDED_CURVE()
B_SPLINE_CURVE(2,(#37762,#37763,#37764),.UNSPECIFIED.,.F.,.F.)
B_SPLINE_CURVE_WITH_KNOTS((3,3),(0.536094506482402,0.589144372850584),
 .UNSPECIFIED.)
CURVE()
GEOMETRIC_REPRESENTATION_ITEM()
RATIONAL_B_SPLINE_CURVE((1.02428162962088,1.0231133608945,1.02147610369983))
REPRESENTATION_ITEM('')
);
#791=(
BOUNDED_CURVE()
B_SPLINE_CURVE(2,(#37768,#37769,#37770),.UNSPECIFIED.,.F.,.F.)
B_SPLINE_CURVE_WITH_KNOTS((3,3),(0.218746031477161,0.271795897845343),
 .UNSPECIFIED.)
CURVE()
GEOMETRIC_REPRESENTATION_ITEM()
RATIONAL_B_SPLINE_CURVE((1.02147610369988,1.02311336089455,1.02428162962093))
REPRESENTATION_ITEM('')
);
#792=(
BOUNDED_CURVE()
B_SPLINE_CURVE(2,(#37772,#37773,#37774),.UNSPECIFIED.,.F.,.F.)
B_SPLINE_CURVE_WITH_KNOTS((3,3),(0.536094506482405,0.589144372850588),
 .UNSPECIFIED.)
CURVE()
GEOMETRIC_REPRESENTATION_ITEM()
RATIONAL_B_SPLINE_CURVE((1.02428162962095,1.02311336089456,1.02147610369989))
REPRESENTATION_ITEM('')
);
#793=(
BOUNDED_CURVE()
B_SPLINE_CURVE(2,(#37778,#37779,#37780),.UNSPECIFIED.,.F.,.F.)
B_SPLINE_CURVE_WITH_KNOTS((3,3),(0.218746031477168,0.271795897845349),
 .UNSPECIFIED.)
CURVE()
GEOMETRIC_REPRESENTATION_ITEM()
RATIONAL_B_SPLINE_CURVE((1.02147610369985,1.02311336089452,1.0242816296209))
REPRESENTATION_ITEM('')
);
#794=(
BOUNDED_CURVE()
B_SPLINE_CURVE(2,(#37782,#37783,#37784),.UNSPECIFIED.,.F.,.F.)
B_SPLINE_CURVE_WITH_KNOTS((3,3),(0.536094506482408,0.589144372850595),
 .UNSPECIFIED.)
CURVE()
GEOMETRIC_REPRESENTATION_ITEM()
RATIONAL_B_SPLINE_CURVE((1.024281629621,1.02311336089461,1.02147610369993))
REPRESENTATION_ITEM('')
);
#795=(
BOUNDED_CURVE()
B_SPLINE_CURVE(2,(#37788,#37789,#37790),.UNSPECIFIED.,.F.,.F.)
B_SPLINE_CURVE_WITH_KNOTS((3,3),(0.218746031477171,0.271795897845352),
 .UNSPECIFIED.)
CURVE()
GEOMETRIC_REPRESENTATION_ITEM()
RATIONAL_B_SPLINE_CURVE((1.02147610369985,1.02311336089452,1.0242816296209))
REPRESENTATION_ITEM('')
);
#796=(
BOUNDED_CURVE()
B_SPLINE_CURVE(2,(#37792,#37793,#37794),.UNSPECIFIED.,.F.,.F.)
B_SPLINE_CURVE_WITH_KNOTS((3,3),(0.536094506482397,0.589144372850578),
 .UNSPECIFIED.)
CURVE()
GEOMETRIC_REPRESENTATION_ITEM()
RATIONAL_B_SPLINE_CURVE((1.02428162962088,1.02311336089449,1.02147610369983))
REPRESENTATION_ITEM('')
);
#797=(
BOUNDED_CURVE()
B_SPLINE_CURVE(2,(#37798,#37799,#37800),.UNSPECIFIED.,.F.,.F.)
B_SPLINE_CURVE_WITH_KNOTS((3,3),(0.218746031477161,0.271795897845346),
 .UNSPECIFIED.)
CURVE()
GEOMETRIC_REPRESENTATION_ITEM()
RATIONAL_B_SPLINE_CURVE((1.02147610369991,1.02311336089458,1.02428162962097))
REPRESENTATION_ITEM('')
);
#798=(
BOUNDED_CURVE()
B_SPLINE_CURVE(2,(#37802,#37803,#37804),.UNSPECIFIED.,.F.,.F.)
B_SPLINE_CURVE_WITH_KNOTS((3,3),(0.536094506482397,0.589144372850583),
 .UNSPECIFIED.)
CURVE()
GEOMETRIC_REPRESENTATION_ITEM()
RATIONAL_B_SPLINE_CURVE((1.02428162962098,1.02311336089459,1.02147610369992))
REPRESENTATION_ITEM('')
);
#799=(
BOUNDED_CURVE()
B_SPLINE_CURVE(2,(#37808,#37809,#37810),.UNSPECIFIED.,.F.,.F.)
B_SPLINE_CURVE_WITH_KNOTS((3,3),(0.218746031477178,0.271795897845362),
 .UNSPECIFIED.)
CURVE()
GEOMETRIC_REPRESENTATION_ITEM()
RATIONAL_B_SPLINE_CURVE((1.02147610369987,1.02311336089454,1.02428162962093))
REPRESENTATION_ITEM('')
);
#800=(
BOUNDED_CURVE()
B_SPLINE_CURVE(2,(#37812,#37813,#37814),.UNSPECIFIED.,.F.,.F.)
B_SPLINE_CURVE_WITH_KNOTS((3,3),(0.536094506482401,0.589144372850588),
 .UNSPECIFIED.)
CURVE()
GEOMETRIC_REPRESENTATION_ITEM()
RATIONAL_B_SPLINE_CURVE((1.02428162962099,1.0231133608946,1.02147610369993))
REPRESENTATION_ITEM('')
);
#801=(
BOUNDED_CURVE()
B_SPLINE_CURVE(2,(#37818,#37819,#37820),.UNSPECIFIED.,.F.,.F.)
B_SPLINE_CURVE_WITH_KNOTS((3,3),(0.218746031477169,0.271795897845355),
 .UNSPECIFIED.)
CURVE()
GEOMETRIC_REPRESENTATION_ITEM()
RATIONAL_B_SPLINE_CURVE((1.02147610369993,1.02311336089461,1.024281629621))
REPRESENTATION_ITEM('')
);
#802=(
BOUNDED_CURVE()
B_SPLINE_CURVE(2,(#37822,#37823,#37824),.UNSPECIFIED.,.F.,.F.)
B_SPLINE_CURVE_WITH_KNOTS((3,3),(0.536094506482416,0.589144372850602),
 .UNSPECIFIED.)
CURVE()
GEOMETRIC_REPRESENTATION_ITEM()
RATIONAL_B_SPLINE_CURVE((1.02428162962103,1.02311336089464,1.02147610369996))
REPRESENTATION_ITEM('')
);
#803=(
BOUNDED_CURVE()
B_SPLINE_CURVE(2,(#37828,#37829,#37830),.UNSPECIFIED.,.F.,.F.)
B_SPLINE_CURVE_WITH_KNOTS((3,3),(0.218746031477151,0.271795897845338),
 .UNSPECIFIED.)
CURVE()
GEOMETRIC_REPRESENTATION_ITEM()
RATIONAL_B_SPLINE_CURVE((1.02147610369997,1.02311336089465,1.02428162962104))
REPRESENTATION_ITEM('')
);
#804=(
BOUNDED_CURVE()
B_SPLINE_CURVE(2,(#37832,#37833,#37834),.UNSPECIFIED.,.F.,.F.)
B_SPLINE_CURVE_WITH_KNOTS((3,3),(0.536094506482404,0.589144372850587),
 .UNSPECIFIED.)
CURVE()
GEOMETRIC_REPRESENTATION_ITEM()
RATIONAL_B_SPLINE_CURVE((1.02428162962093,1.02311336089454,1.02147610369987))
REPRESENTATION_ITEM('')
);
#805=(
BOUNDED_CURVE()
B_SPLINE_CURVE(2,(#37838,#37839,#37840),.UNSPECIFIED.,.F.,.F.)
B_SPLINE_CURVE_WITH_KNOTS((3,3),(0.21874603147716,0.271795897845347),
 .UNSPECIFIED.)
CURVE()
GEOMETRIC_REPRESENTATION_ITEM()
RATIONAL_B_SPLINE_CURVE((1.02147610369994,1.02311336089462,1.02428162962101))
REPRESENTATION_ITEM('')
);
#806=(
BOUNDED_CURVE()
B_SPLINE_CURVE(2,(#37842,#37843,#37844),.UNSPECIFIED.,.F.,.F.)
B_SPLINE_CURVE_WITH_KNOTS((3,3),(0.536094506482402,0.589144372850585),
 .UNSPECIFIED.)
CURVE()
GEOMETRIC_REPRESENTATION_ITEM()
RATIONAL_B_SPLINE_CURVE((1.02428162962091,1.02311336089452,1.02147610369985))
REPRESENTATION_ITEM('')
);
#807=(
BOUNDED_CURVE()
B_SPLINE_CURVE(2,(#37848,#37849,#37850),.UNSPECIFIED.,.F.,.F.)
B_SPLINE_CURVE_WITH_KNOTS((3,3),(0.218746031477168,0.271795897845356),
 .UNSPECIFIED.)
CURVE()
GEOMETRIC_REPRESENTATION_ITEM()
RATIONAL_B_SPLINE_CURVE((1.02147610369995,1.02311336089462,1.02428162962101))
REPRESENTATION_ITEM('')
);
#808=(
BOUNDED_CURVE()
B_SPLINE_CURVE(2,(#37852,#37853,#37854),.UNSPECIFIED.,.F.,.F.)
B_SPLINE_CURVE_WITH_KNOTS((3,3),(0.536094506482419,0.589144372850602),
 .UNSPECIFIED.)
CURVE()
GEOMETRIC_REPRESENTATION_ITEM()
RATIONAL_B_SPLINE_CURVE((1.02428162962094,1.02311336089456,1.02147610369988))
REPRESENTATION_ITEM('')
);
#809=(
BOUNDED_CURVE()
B_SPLINE_CURVE(2,(#37858,#37859,#37860),.UNSPECIFIED.,.F.,.F.)
B_SPLINE_CURVE_WITH_KNOTS((3,3),(0.218746031477172,0.271795897845351),
 .UNSPECIFIED.)
CURVE()
GEOMETRIC_REPRESENTATION_ITEM()
RATIONAL_B_SPLINE_CURVE((1.02147610369981,1.02311336089447,1.02428162962086))
REPRESENTATION_ITEM('')
);
#810=(
BOUNDED_CURVE()
B_SPLINE_CURVE(2,(#37862,#37863,#37864),.UNSPECIFIED.,.F.,.F.)
B_SPLINE_CURVE_WITH_KNOTS((3,3),(0.536094506482413,0.589144372850597),
 .UNSPECIFIED.)
CURVE()
GEOMETRIC_REPRESENTATION_ITEM()
RATIONAL_B_SPLINE_CURVE((1.02428162962095,1.02311336089456,1.02147610369989))
REPRESENTATION_ITEM('')
);
#811=(
BOUNDED_CURVE()
B_SPLINE_CURVE(2,(#37868,#37869,#37870),.UNSPECIFIED.,.F.,.F.)
B_SPLINE_CURVE_WITH_KNOTS((3,3),(0.218746031477175,0.271795897845363),
 .UNSPECIFIED.)
CURVE()
GEOMETRIC_REPRESENTATION_ITEM()
RATIONAL_B_SPLINE_CURVE((1.02147610369996,1.02311336089463,1.02428162962103))
REPRESENTATION_ITEM('')
);
#812=(
BOUNDED_CURVE()
B_SPLINE_CURVE(2,(#37872,#37873,#37874),.UNSPECIFIED.,.F.,.F.)
B_SPLINE_CURVE_WITH_KNOTS((3,3),(0.536094506482418,0.589144372850602),
 .UNSPECIFIED.)
CURVE()
GEOMETRIC_REPRESENTATION_ITEM()
RATIONAL_B_SPLINE_CURVE((1.02428162962098,1.02311336089459,1.02147610369991))
REPRESENTATION_ITEM('')
);
#813=(
BOUNDED_CURVE()
B_SPLINE_CURVE(2,(#37878,#37879,#37880),.UNSPECIFIED.,.F.,.F.)
B_SPLINE_CURVE_WITH_KNOTS((3,3),(0.21874603147716,0.271795897845347),
 .UNSPECIFIED.)
CURVE()
GEOMETRIC_REPRESENTATION_ITEM()
RATIONAL_B_SPLINE_CURVE((1.02147610369995,1.02311336089463,1.02428162962102))
REPRESENTATION_ITEM('')
);
#814=(
BOUNDED_CURVE()
B_SPLINE_CURVE(2,(#37882,#37883,#37884),.UNSPECIFIED.,.F.,.F.)
B_SPLINE_CURVE_WITH_KNOTS((3,3),(0.536094506482396,0.589144372850583),
 .UNSPECIFIED.)
CURVE()
GEOMETRIC_REPRESENTATION_ITEM()
RATIONAL_B_SPLINE_CURVE((1.02428162962099,1.0231133608946,1.02147610369992))
REPRESENTATION_ITEM('')
);
#815=(
BOUNDED_CURVE()
B_SPLINE_CURVE(2,(#37888,#37889,#37890),.UNSPECIFIED.,.F.,.F.)
B_SPLINE_CURVE_WITH_KNOTS((3,3),(0.218746031477158,0.271795897845343),
 .UNSPECIFIED.)
CURVE()
GEOMETRIC_REPRESENTATION_ITEM()
RATIONAL_B_SPLINE_CURVE((1.02147610369992,1.02311336089459,1.02428162962098))
REPRESENTATION_ITEM('')
);
#816=(
BOUNDED_CURVE()
B_SPLINE_CURVE(2,(#37892,#37893,#37894),.UNSPECIFIED.,.F.,.F.)
B_SPLINE_CURVE_WITH_KNOTS((3,3),(0.536094506482406,0.589144372850593),
 .UNSPECIFIED.)
CURVE()
GEOMETRIC_REPRESENTATION_ITEM()
RATIONAL_B_SPLINE_CURVE((1.02428162962099,1.0231133608946,1.02147610369993))
REPRESENTATION_ITEM('')
);
#817=(
BOUNDED_CURVE()
B_SPLINE_CURVE(2,(#37898,#37899,#37900),.UNSPECIFIED.,.F.,.F.)
B_SPLINE_CURVE_WITH_KNOTS((3,3),(0.218746031477158,0.271795897845344),
 .UNSPECIFIED.)
CURVE()
GEOMETRIC_REPRESENTATION_ITEM()
RATIONAL_B_SPLINE_CURVE((1.02147610369995,1.02311336089462,1.02428162962101))
REPRESENTATION_ITEM('')
);
#818=(
BOUNDED_CURVE()
B_SPLINE_CURVE(2,(#37902,#37903,#37904),.UNSPECIFIED.,.F.,.F.)
B_SPLINE_CURVE_WITH_KNOTS((3,3),(0.536094506482404,0.589144372850588),
 .UNSPECIFIED.)
CURVE()
GEOMETRIC_REPRESENTATION_ITEM()
RATIONAL_B_SPLINE_CURVE((1.02428162962094,1.02311336089456,1.02147610369989))
REPRESENTATION_ITEM('')
);
#819=(
BOUNDED_CURVE()
B_SPLINE_CURVE(2,(#37908,#37909,#37910),.UNSPECIFIED.,.F.,.F.)
B_SPLINE_CURVE_WITH_KNOTS((3,3),(0.218746031477163,0.271795897845347),
 .UNSPECIFIED.)
CURVE()
GEOMETRIC_REPRESENTATION_ITEM()
RATIONAL_B_SPLINE_CURVE((1.0214761036999,1.02311336089458,1.02428162962097))
REPRESENTATION_ITEM('')
);
#820=(
BOUNDED_CURVE()
B_SPLINE_CURVE(2,(#37912,#37913,#37914),.UNSPECIFIED.,.F.,.F.)
B_SPLINE_CURVE_WITH_KNOTS((3,3),(0.536094506482397,0.589144372850583),
 .UNSPECIFIED.)
CURVE()
GEOMETRIC_REPRESENTATION_ITEM()
RATIONAL_B_SPLINE_CURVE((1.02428162962099,1.0231133608946,1.02147610369992))
REPRESENTATION_ITEM('')
);
#821=(
BOUNDED_CURVE()
B_SPLINE_CURVE(2,(#37918,#37919,#37920),.UNSPECIFIED.,.F.,.F.)
B_SPLINE_CURVE_WITH_KNOTS((3,3),(0.218746031477164,0.271795897845345),
 .UNSPECIFIED.)
CURVE()
GEOMETRIC_REPRESENTATION_ITEM()
RATIONAL_B_SPLINE_CURVE((1.02147610369985,1.02311336089451,1.0242816296209))
REPRESENTATION_ITEM('')
);
#822=(
BOUNDED_CURVE()
B_SPLINE_CURVE(2,(#37922,#37923,#37924),.UNSPECIFIED.,.F.,.F.)
B_SPLINE_CURVE_WITH_KNOTS((3,3),(0.536094506482409,0.589144372850595),
 .UNSPECIFIED.)
CURVE()
GEOMETRIC_REPRESENTATION_ITEM()
RATIONAL_B_SPLINE_CURVE((1.02428162962099,1.0231133608946,1.02147610369992))
REPRESENTATION_ITEM('')
);
#823=(
BOUNDED_CURVE()
B_SPLINE_CURVE(2,(#37928,#37929,#37930),.UNSPECIFIED.,.F.,.F.)
B_SPLINE_CURVE_WITH_KNOTS((3,3),(0.218746031477171,0.271795897845354),
 .UNSPECIFIED.)
CURVE()
GEOMETRIC_REPRESENTATION_ITEM()
RATIONAL_B_SPLINE_CURVE((1.02147610369987,1.02311336089454,1.02428162962093))
REPRESENTATION_ITEM('')
);
#824=(
BOUNDED_CURVE()
B_SPLINE_CURVE(2,(#37932,#37933,#37934),.UNSPECIFIED.,.F.,.F.)
B_SPLINE_CURVE_WITH_KNOTS((3,3),(0.536094506482407,0.589144372850591),
 .UNSPECIFIED.)
CURVE()
GEOMETRIC_REPRESENTATION_ITEM()
RATIONAL_B_SPLINE_CURVE((1.02428162962096,1.02311336089457,1.0214761036999))
REPRESENTATION_ITEM('')
);
#825=(
BOUNDED_CURVE()
B_SPLINE_CURVE(2,(#37938,#37939,#37940),.UNSPECIFIED.,.F.,.F.)
B_SPLINE_CURVE_WITH_KNOTS((3,3),(0.218746031477165,0.271795897845349),
 .UNSPECIFIED.)
CURVE()
GEOMETRIC_REPRESENTATION_ITEM()
RATIONAL_B_SPLINE_CURVE((1.0214761036999,1.02311336089457,1.02428162962096))
REPRESENTATION_ITEM('')
);
#826=(
BOUNDED_CURVE()
B_SPLINE_CURVE(2,(#37942,#37943,#37944),.UNSPECIFIED.,.F.,.F.)
B_SPLINE_CURVE_WITH_KNOTS((3,3),(0.53609450648241,0.589144372850595),
 .UNSPECIFIED.)
CURVE()
GEOMETRIC_REPRESENTATION_ITEM()
RATIONAL_B_SPLINE_CURVE((1.02428162962096,1.02311336089458,1.0214761036999))
REPRESENTATION_ITEM('')
);
#827=(
BOUNDED_CURVE()
B_SPLINE_CURVE(2,(#37948,#37949,#37950),.UNSPECIFIED.,.F.,.F.)
B_SPLINE_CURVE_WITH_KNOTS((3,3),(0.218746031477166,0.271795897845348),
 .UNSPECIFIED.)
CURVE()
GEOMETRIC_REPRESENTATION_ITEM()
RATIONAL_B_SPLINE_CURVE((1.02147610369988,1.02311336089455,1.02428162962094))
REPRESENTATION_ITEM('')
);
#828=(
BOUNDED_CURVE()
B_SPLINE_CURVE(2,(#37952,#37953,#37954),.UNSPECIFIED.,.F.,.F.)
B_SPLINE_CURVE_WITH_KNOTS((3,3),(0.53609450648241,0.589144372850593),
 .UNSPECIFIED.)
CURVE()
GEOMETRIC_REPRESENTATION_ITEM()
RATIONAL_B_SPLINE_CURVE((1.02428162962095,1.02311336089456,1.02147610369989))
REPRESENTATION_ITEM('')
);
#829=(
BOUNDED_CURVE()
B_SPLINE_CURVE(2,(#37958,#37959,#37960),.UNSPECIFIED.,.F.,.F.)
B_SPLINE_CURVE_WITH_KNOTS((3,3),(0.21874603147716,0.271795897845347),
 .UNSPECIFIED.)
CURVE()
GEOMETRIC_REPRESENTATION_ITEM()
RATIONAL_B_SPLINE_CURVE((1.02147610369996,1.02311336089463,1.02428162962102))
REPRESENTATION_ITEM('')
);
#830=(
BOUNDED_CURVE()
B_SPLINE_CURVE(2,(#37962,#37963,#37964),.UNSPECIFIED.,.F.,.F.)
B_SPLINE_CURVE_WITH_KNOTS((3,3),(0.53609450648241,0.589144372850594),
 .UNSPECIFIED.)
CURVE()
GEOMETRIC_REPRESENTATION_ITEM()
RATIONAL_B_SPLINE_CURVE((1.02428162962095,1.02311336089456,1.02147610369989))
REPRESENTATION_ITEM('')
);
#831=(
BOUNDED_CURVE()
B_SPLINE_CURVE(2,(#37968,#37969,#37970),.UNSPECIFIED.,.F.,.F.)
B_SPLINE_CURVE_WITH_KNOTS((3,3),(0.218746031477162,0.271795897845348),
 .UNSPECIFIED.)
CURVE()
GEOMETRIC_REPRESENTATION_ITEM()
RATIONAL_B_SPLINE_CURVE((1.02147610369995,1.02311336089463,1.02428162962102))
REPRESENTATION_ITEM('')
);
#832=(
BOUNDED_CURVE()
B_SPLINE_CURVE(2,(#37972,#37973,#37974),.UNSPECIFIED.,.F.,.F.)
B_SPLINE_CURVE_WITH_KNOTS((3,3),(0.536094506482406,0.589144372850593),
 .UNSPECIFIED.)
CURVE()
GEOMETRIC_REPRESENTATION_ITEM()
RATIONAL_B_SPLINE_CURVE((1.024281629621,1.02311336089461,1.02147610369993))
REPRESENTATION_ITEM('')
);
#833=(
BOUNDED_CURVE()
B_SPLINE_CURVE(2,(#37978,#37979,#37980),.UNSPECIFIED.,.F.,.F.)
B_SPLINE_CURVE_WITH_KNOTS((3,3),(0.218746031477166,0.271795897845352),
 .UNSPECIFIED.)
CURVE()
GEOMETRIC_REPRESENTATION_ITEM()
RATIONAL_B_SPLINE_CURVE((1.02147610369994,1.02311336089462,1.02428162962101))
REPRESENTATION_ITEM('')
);
#834=(
BOUNDED_CURVE()
B_SPLINE_CURVE(2,(#37982,#37983,#37984),.UNSPECIFIED.,.F.,.F.)
B_SPLINE_CURVE_WITH_KNOTS((3,3),(0.536094506482414,0.589144372850599),
 .UNSPECIFIED.)
CURVE()
GEOMETRIC_REPRESENTATION_ITEM()
RATIONAL_B_SPLINE_CURVE((1.02428162962095,1.02311336089456,1.02147610369989))
REPRESENTATION_ITEM('')
);
#835=(
BOUNDED_CURVE()
B_SPLINE_CURVE(2,(#37988,#37989,#37990),.UNSPECIFIED.,.F.,.F.)
B_SPLINE_CURVE_WITH_KNOTS((3,3),(0.218746031477169,0.271795897845355),
 .UNSPECIFIED.)
CURVE()
GEOMETRIC_REPRESENTATION_ITEM()
RATIONAL_B_SPLINE_CURVE((1.02147610369993,1.0231133608946,1.02428162962099))
REPRESENTATION_ITEM('')
);
#836=(
BOUNDED_CURVE()
B_SPLINE_CURVE(2,(#37992,#37993,#37994),.UNSPECIFIED.,.F.,.F.)
B_SPLINE_CURVE_WITH_KNOTS((3,3),(0.536094506482414,0.589144372850597),
 .UNSPECIFIED.)
CURVE()
GEOMETRIC_REPRESENTATION_ITEM()
RATIONAL_B_SPLINE_CURVE((1.02428162962095,1.02311336089457,1.02147610369989))
REPRESENTATION_ITEM('')
);
#837=(
BOUNDED_CURVE()
B_SPLINE_CURVE(2,(#37998,#37999,#38000),.UNSPECIFIED.,.F.,.F.)
B_SPLINE_CURVE_WITH_KNOTS((3,3),(0.218746031477173,0.271795897845359),
 .UNSPECIFIED.)
CURVE()
GEOMETRIC_REPRESENTATION_ITEM()
RATIONAL_B_SPLINE_CURVE((1.02147610369992,1.02311336089459,1.02428162962098))
REPRESENTATION_ITEM('')
);
#838=(
BOUNDED_CURVE()
B_SPLINE_CURVE(2,(#38002,#38003,#38004),.UNSPECIFIED.,.F.,.F.)
B_SPLINE_CURVE_WITH_KNOTS((3,3),(0.536094506482406,0.589144372850592),
 .UNSPECIFIED.)
CURVE()
GEOMETRIC_REPRESENTATION_ITEM()
RATIONAL_B_SPLINE_CURVE((1.02428162962098,1.02311336089459,1.02147610369992))
REPRESENTATION_ITEM('')
);
#839=(
BOUNDED_CURVE()
B_SPLINE_CURVE(2,(#38008,#38009,#38010),.UNSPECIFIED.,.F.,.F.)
B_SPLINE_CURVE_WITH_KNOTS((3,3),(0.218746031477167,0.271795897845351),
 .UNSPECIFIED.)
CURVE()
GEOMETRIC_REPRESENTATION_ITEM()
RATIONAL_B_SPLINE_CURVE((1.02147610369989,1.02311336089456,1.02428162962095))
REPRESENTATION_ITEM('')
);
#840=(
BOUNDED_CURVE()
B_SPLINE_CURVE(2,(#38012,#38013,#38014),.UNSPECIFIED.,.F.,.F.)
B_SPLINE_CURVE_WITH_KNOTS((3,3),(0.536094506482407,0.589144372850592),
 .UNSPECIFIED.)
CURVE()
GEOMETRIC_REPRESENTATION_ITEM()
RATIONAL_B_SPLINE_CURVE((1.02428162962097,1.02311336089458,1.02147610369991))
REPRESENTATION_ITEM('')
);
#841=(
BOUNDED_CURVE()
B_SPLINE_CURVE(2,(#38018,#38019,#38020),.UNSPECIFIED.,.F.,.F.)
B_SPLINE_CURVE_WITH_KNOTS((3,3),(0.218746031477175,0.271795897845359),
 .UNSPECIFIED.)
CURVE()
GEOMETRIC_REPRESENTATION_ITEM()
RATIONAL_B_SPLINE_CURVE((1.02147610369989,1.02311336089456,1.02428162962095))
REPRESENTATION_ITEM('')
);
#842=(
BOUNDED_CURVE()
B_SPLINE_CURVE(2,(#38022,#38023,#38024),.UNSPECIFIED.,.F.,.F.)
B_SPLINE_CURVE_WITH_KNOTS((3,3),(0.536094506482402,0.589144372850588),
 .UNSPECIFIED.)
CURVE()
GEOMETRIC_REPRESENTATION_ITEM()
RATIONAL_B_SPLINE_CURVE((1.02428162962098,1.02311336089459,1.02147610369991))
REPRESENTATION_ITEM('')
);
#843=(
BOUNDED_CURVE()
B_SPLINE_CURVE(2,(#38028,#38029,#38030),.UNSPECIFIED.,.F.,.F.)
B_SPLINE_CURVE_WITH_KNOTS((3,3),(0.218746031477175,0.271795897845355),
 .UNSPECIFIED.)
CURVE()
GEOMETRIC_REPRESENTATION_ITEM()
RATIONAL_B_SPLINE_CURVE((1.02147610369982,1.02311336089449,1.02428162962087))
REPRESENTATION_ITEM('')
);
#844=(
BOUNDED_CURVE()
B_SPLINE_CURVE(2,(#38032,#38033,#38034),.UNSPECIFIED.,.F.,.F.)
B_SPLINE_CURVE_WITH_KNOTS((3,3),(0.536094506482407,0.589144372850592),
 .UNSPECIFIED.)
CURVE()
GEOMETRIC_REPRESENTATION_ITEM()
RATIONAL_B_SPLINE_CURVE((1.02428162962096,1.02311336089457,1.0214761036999))
REPRESENTATION_ITEM('')
);
#845=(
BOUNDED_CURVE()
B_SPLINE_CURVE(2,(#38038,#38039,#38040),.UNSPECIFIED.,.F.,.F.)
B_SPLINE_CURVE_WITH_KNOTS((3,3),(0.21874603147717,0.271795897845352),
 .UNSPECIFIED.)
CURVE()
GEOMETRIC_REPRESENTATION_ITEM()
RATIONAL_B_SPLINE_CURVE((1.02147610369985,1.02311336089452,1.02428162962091))
REPRESENTATION_ITEM('')
);
#846=(
BOUNDED_CURVE()
B_SPLINE_CURVE(2,(#38042,#38043,#38044),.UNSPECIFIED.,.F.,.F.)
B_SPLINE_CURVE_WITH_KNOTS((3,3),(0.536094506482403,0.589144372850591),
 .UNSPECIFIED.)
CURVE()
GEOMETRIC_REPRESENTATION_ITEM()
RATIONAL_B_SPLINE_CURVE((1.02428162962102,1.02311336089463,1.02147610369996))
REPRESENTATION_ITEM('')
);
#847=(
BOUNDED_CURVE()
B_SPLINE_CURVE(2,(#38048,#38049,#38050),.UNSPECIFIED.,.F.,.F.)
B_SPLINE_CURVE_WITH_KNOTS((3,3),(0.218746031477164,0.271795897845349),
 .UNSPECIFIED.)
CURVE()
GEOMETRIC_REPRESENTATION_ITEM()
RATIONAL_B_SPLINE_CURVE((1.02147610369991,1.02311336089459,1.02428162962097))
REPRESENTATION_ITEM('')
);
#848=(
BOUNDED_CURVE()
B_SPLINE_CURVE(2,(#38052,#38053,#38054),.UNSPECIFIED.,.F.,.F.)
B_SPLINE_CURVE_WITH_KNOTS((3,3),(0.536094506482412,0.589144372850596),
 .UNSPECIFIED.)
CURVE()
GEOMETRIC_REPRESENTATION_ITEM()
RATIONAL_B_SPLINE_CURVE((1.02428162962096,1.02311336089457,1.0214761036999))
REPRESENTATION_ITEM('')
);
#849=(
BOUNDED_CURVE()
B_SPLINE_CURVE(2,(#38058,#38059,#38060),.UNSPECIFIED.,.F.,.F.)
B_SPLINE_CURVE_WITH_KNOTS((3,3),(0.218746031477168,0.27179589784535),
 .UNSPECIFIED.)
CURVE()
GEOMETRIC_REPRESENTATION_ITEM()
RATIONAL_B_SPLINE_CURVE((1.02147610369985,1.02311336089452,1.0242816296209))
REPRESENTATION_ITEM('')
);
#850=(
BOUNDED_CURVE()
B_SPLINE_CURVE(2,(#38062,#38063,#38064),.UNSPECIFIED.,.F.,.F.)
B_SPLINE_CURVE_WITH_KNOTS((3,3),(0.536094506482416,0.589144372850602),
 .UNSPECIFIED.)
CURVE()
GEOMETRIC_REPRESENTATION_ITEM()
RATIONAL_B_SPLINE_CURVE((1.02428162962097,1.02311336089458,1.02147610369991))
REPRESENTATION_ITEM('')
);
#851=(
BOUNDED_CURVE()
B_SPLINE_CURVE(2,(#38068,#38069,#38070),.UNSPECIFIED.,.F.,.F.)
B_SPLINE_CURVE_WITH_KNOTS((3,3),(0.218746031477172,0.271795897845358),
 .UNSPECIFIED.)
CURVE()
GEOMETRIC_REPRESENTATION_ITEM()
RATIONAL_B_SPLINE_CURVE((1.02147610369993,1.02311336089461,1.024281629621))
REPRESENTATION_ITEM('')
);
#852=(
BOUNDED_CURVE()
B_SPLINE_CURVE(2,(#38072,#38073,#38074),.UNSPECIFIED.,.F.,.F.)
B_SPLINE_CURVE_WITH_KNOTS((3,3),(0.536094506482398,0.589144372850586),
 .UNSPECIFIED.)
CURVE()
GEOMETRIC_REPRESENTATION_ITEM()
RATIONAL_B_SPLINE_CURVE((1.02428162962101,1.02311336089462,1.02147610369994))
REPRESENTATION_ITEM('')
);
#853=(
BOUNDED_CURVE()
B_SPLINE_CURVE(2,(#38078,#38079,#38080),.UNSPECIFIED.,.F.,.F.)
B_SPLINE_CURVE_WITH_KNOTS((3,3),(0.218746031477161,0.271795897845345),
 .UNSPECIFIED.)
CURVE()
GEOMETRIC_REPRESENTATION_ITEM()
RATIONAL_B_SPLINE_CURVE((1.02147610369992,1.02311336089459,1.02428162962098))
REPRESENTATION_ITEM('')
);
#854=(
BOUNDED_CURVE()
B_SPLINE_CURVE(2,(#38082,#38083,#38084),.UNSPECIFIED.,.F.,.F.)
B_SPLINE_CURVE_WITH_KNOTS((3,3),(0.536094506482393,0.58914437285058),
 .UNSPECIFIED.)
CURVE()
GEOMETRIC_REPRESENTATION_ITEM()
RATIONAL_B_SPLINE_CURVE((1.02428162962098,1.02311336089459,1.02147610369992))
REPRESENTATION_ITEM('')
);
#855=(
BOUNDED_CURVE()
B_SPLINE_CURVE(2,(#38088,#38089,#38090),.UNSPECIFIED.,.F.,.F.)
B_SPLINE_CURVE_WITH_KNOTS((3,3),(0.21874603147716,0.271795897845346),
 .UNSPECIFIED.)
CURVE()
GEOMETRIC_REPRESENTATION_ITEM()
RATIONAL_B_SPLINE_CURVE((1.02147610369996,1.02311336089463,1.02428162962102))
REPRESENTATION_ITEM('')
);
#856=(
BOUNDED_CURVE()
B_SPLINE_CURVE(2,(#38092,#38093,#38094),.UNSPECIFIED.,.F.,.F.)
B_SPLINE_CURVE_WITH_KNOTS((3,3),(0.536094506482404,0.589144372850591),
 .UNSPECIFIED.)
CURVE()
GEOMETRIC_REPRESENTATION_ITEM()
RATIONAL_B_SPLINE_CURVE((1.02428162962101,1.02311336089461,1.02147610369994))
REPRESENTATION_ITEM('')
);
#857=(
BOUNDED_CURVE()
B_SPLINE_CURVE(2,(#38098,#38099,#38100),.UNSPECIFIED.,.F.,.F.)
B_SPLINE_CURVE_WITH_KNOTS((3,3),(0.218746031477173,0.271795897845354),
 .UNSPECIFIED.)
CURVE()
GEOMETRIC_REPRESENTATION_ITEM()
RATIONAL_B_SPLINE_CURVE((1.02147610369983,1.0231133608945,1.02428162962088))
REPRESENTATION_ITEM('')
);
#858=(
BOUNDED_CURVE()
B_SPLINE_CURVE(2,(#38102,#38103,#38104),.UNSPECIFIED.,.F.,.F.)
B_SPLINE_CURVE_WITH_KNOTS((3,3),(0.536094506482412,0.589144372850603),
 .UNSPECIFIED.)
CURVE()
GEOMETRIC_REPRESENTATION_ITEM()
RATIONAL_B_SPLINE_CURVE((1.02428162962111,1.02311336089471,1.02147610370003))
REPRESENTATION_ITEM('')
);
#859=(
BOUNDED_CURVE()
B_SPLINE_CURVE(2,(#38108,#38109,#38110),.UNSPECIFIED.,.F.,.F.)
B_SPLINE_CURVE_WITH_KNOTS((3,3),(0.218746031477171,0.271795897845355),
 .UNSPECIFIED.)
CURVE()
GEOMETRIC_REPRESENTATION_ITEM()
RATIONAL_B_SPLINE_CURVE((1.02147610369989,1.02311336089456,1.02428162962095))
REPRESENTATION_ITEM('')
);
#860=(
BOUNDED_CURVE()
B_SPLINE_CURVE(2,(#38112,#38113,#38114),.UNSPECIFIED.,.F.,.F.)
B_SPLINE_CURVE_WITH_KNOTS((3,3),(0.536094506482401,0.589144372850588),
 .UNSPECIFIED.)
CURVE()
GEOMETRIC_REPRESENTATION_ITEM()
RATIONAL_B_SPLINE_CURVE((1.02428162962099,1.0231133608946,1.02147610369993))
REPRESENTATION_ITEM('')
);
#861=(
BOUNDED_CURVE()
B_SPLINE_CURVE(2,(#38117,#38118,#38119),.UNSPECIFIED.,.F.,.F.)
B_SPLINE_CURVE_WITH_KNOTS((3,3),(0.218746031477171,0.271795897845354),
 .UNSPECIFIED.)
CURVE()
GEOMETRIC_REPRESENTATION_ITEM()
RATIONAL_B_SPLINE_CURVE((1.02147610369987,1.02311336089454,1.02428162962093))
REPRESENTATION_ITEM('')
);
#885=FACE_BOUND('',#3017,.T.);
#886=FACE_BOUND('',#3018,.T.);
#887=FACE_BOUND('',#3023,.T.);
#888=FACE_BOUND('',#3024,.T.);
#889=FACE_BOUND('',#3026,.T.);
#890=FACE_BOUND('',#3028,.T.);
#891=FACE_BOUND('',#3032,.T.);
#892=FACE_BOUND('',#3041,.T.);
#893=FACE_BOUND('',#3047,.T.);
#894=FACE_BOUND('',#3098,.T.);
#895=FACE_BOUND('',#3100,.T.);
#896=FACE_BOUND('',#3103,.T.);
#897=FACE_BOUND('',#3107,.T.);
#898=FACE_BOUND('',#3109,.T.);
#899=FACE_BOUND('',#3111,.T.);
#900=FACE_BOUND('',#3114,.T.);
#901=FACE_BOUND('',#3116,.T.);
#902=FACE_BOUND('',#3120,.T.);
#903=FACE_BOUND('',#3248,.T.);
#904=FACE_BOUND('',#3413,.T.);
#905=FACE_BOUND('',#3540,.T.);
#906=FACE_BOUND('',#3542,.T.);
#1005=B_SPLINE_CURVE_WITH_KNOTS('',3,(#33448,#33449,#33450,#33451,#33452,
#33453,#33454,#33455,#33456,#33457,#33458,#33459,#33460,#33461,#33462,#33463,
#33464,#33465,#33466,#33467,#33468,#33469,#33470,#33471,#33472,#33473,#33474),
 .UNSPECIFIED.,.F.,.F.,(4,2,2,2,2,2,3,2,2,2,2,2,4),(-0.332209547359341,
-0.298546270509129,-0.214461346284245,-0.130376422059361,-0.0858276476044183,
-0.0429138238022092,0.,0.0429138238022091,0.0858276476044183,0.130376422059361,
0.214461346284245,0.298546270509129,0.332209547359342),.UNSPECIFIED.);
#1006=B_SPLINE_CURVE_WITH_KNOTS('',3,(#33640,#33641,#33642,#33643),
 .UNSPECIFIED.,.F.,.F.,(4,4),(0.,0.000427835206687807),.UNSPECIFIED.);
#1007=B_SPLINE_CURVE_WITH_KNOTS('',3,(#33644,#33645,#33646,#33647),
 .UNSPECIFIED.,.F.,.F.,(4,4),(0.,0.000427835206687776),.UNSPECIFIED.);
#1008=B_SPLINE_CURVE_WITH_KNOTS('',3,(#33652,#33653,#33654,#33655),
 .UNSPECIFIED.,.F.,.F.,(4,4),(0.,0.000427835206687808),.UNSPECIFIED.);
#1009=B_SPLINE_CURVE_WITH_KNOTS('',3,(#33656,#33657,#33658,#33659),
 .UNSPECIFIED.,.F.,.F.,(4,4),(3.46944695195361E-18,0.000427835206687798),
 .UNSPECIFIED.);
#1010=B_SPLINE_CURVE_WITH_KNOTS('',3,(#33667,#33668,#33669,#33670),
 .UNSPECIFIED.,.F.,.F.,(4,4),(0.,0.000427835206687807),.UNSPECIFIED.);
#1011=B_SPLINE_CURVE_WITH_KNOTS('',3,(#33671,#33672,#33673,#33674),
 .UNSPECIFIED.,.F.,.F.,(4,4),(0.,0.000427835206687801),.UNSPECIFIED.);
#1012=B_SPLINE_CURVE_WITH_KNOTS('',3,(#33684,#33685,#33686,#33687),
 .UNSPECIFIED.,.F.,.F.,(4,4),(0.,0.000427835206687808),.UNSPECIFIED.);
#1013=B_SPLINE_CURVE_WITH_KNOTS('',3,(#33688,#33689,#33690,#33691),
 .UNSPECIFIED.,.F.,.F.,(4,4),(3.46944695195361E-18,0.000427835206687774),
 .UNSPECIFIED.);
#1014=B_SPLINE_CURVE_WITH_KNOTS('',3,(#36242,#36243,#36244,#36245,#36246,
#36247,#36248,#36249,#36250,#36251),.UNSPECIFIED.,.F.,.F.,(4,2,2,2,4),(0.407230824200947,
0.441482308570059,0.475169509556855,0.508523321203204,0.522738749128563),
 .UNSPECIFIED.);
#1015=B_SPLINE_CURVE_WITH_KNOTS('',3,(#36255,#36256,#36257,#36258,#36259,
#36260,#36261,#36262,#36263,#36264),.UNSPECIFIED.,.F.,.F.,(4,2,2,2,4),(0.0189522566102193,
0.0331676845355794,0.0665214961819283,0.100208697168724,0.134460181537836),
 .UNSPECIFIED.);
#1016=B_SPLINE_CURVE_WITH_KNOTS('',3,(#36275,#36276,#36277,#36278,#36279,
#36280,#36281,#36282,#36283,#36284),.UNSPECIFIED.,.F.,.F.,(4,2,2,2,4),(0.407230824200947,
0.441482308570059,0.475169509556855,0.508523321203204,0.522738749128564),
 .UNSPECIFIED.);
#1017=B_SPLINE_CURVE_WITH_KNOTS('',3,(#36287,#36288,#36289,#36290,#36291,
#36292,#36293,#36294,#36295,#36296),.UNSPECIFIED.,.F.,.F.,(4,2,2,2,4),(0.0189522566102211,
0.0331676845355794,0.0665214961819283,0.100208697168724,0.134460181537836),
 .UNSPECIFIED.);
#1035=CONICAL_SURFACE('',#18448,2.,0.785398163397458);
#1036=CONICAL_SURFACE('',#18451,1.80000000000002,0.785398163397445);
#1037=CONICAL_SURFACE('',#18455,2.3,0.785398163397448);
#1038=CONICAL_SURFACE('',#18459,1.2,0.785398163397454);
#1039=CONICAL_SURFACE('',#18462,3.49999999999998,0.78539816339745);
#1040=CONICAL_SURFACE('',#18465,1.50000000000001,0.785398163397452);
#1041=CONICAL_SURFACE('',#18469,2.3,0.785398163397444);
#1042=CONICAL_SURFACE('',#18473,2.,0.78539816339744);
#1043=CONICAL_SURFACE('',#18476,1.5,0.785398163397444);
#1044=CONICAL_SURFACE('',#18479,3.2,0.785398163397442);
#1045=CONICAL_SURFACE('',#18593,4.,0.785398163397445);
#1046=CONICAL_SURFACE('',#18594,4.,0.785398163397445);
#1047=CONICAL_SURFACE('',#18595,4.29999999999999,0.785398163397445);
#1048=CONICAL_SURFACE('',#18596,4.29999999999998,0.785398163397451);
#1049=CONICAL_SURFACE('',#18660,2.,0.785398163397446);
#1050=CONICAL_SURFACE('',#18664,1.61,0.959931088596875);
#1051=CONICAL_SURFACE('',#18669,2.,0.959931088596884);
#1052=CONICAL_SURFACE('',#18673,1.61,0.959931088596875);
#1053=CONICAL_SURFACE('',#18678,2.,0.959931088596884);
#1054=CONICAL_SURFACE('',#18682,1.61,0.959931088596875);
#1055=CONICAL_SURFACE('',#18687,2.,0.959931088596884);
#1056=CONICAL_SURFACE('',#18691,1.61,0.959931088596875);
#1057=CONICAL_SURFACE('',#18696,2.,0.959931088596884);
#1058=CONICAL_SURFACE('',#18700,1.61,0.959931088596875);
#1059=CONICAL_SURFACE('',#18705,2.,0.959931088596884);
#1060=CONICAL_SURFACE('',#18709,1.61,0.959931088596875);
#1061=CONICAL_SURFACE('',#18714,2.,0.959931088596884);
#1062=CONICAL_SURFACE('',#18718,1.61,0.959931088596875);
#1063=CONICAL_SURFACE('',#18723,2.,0.959931088596884);
#1064=CONICAL_SURFACE('',#18727,1.61,0.959931088596875);
#1065=CONICAL_SURFACE('',#18732,2.,0.959931088596884);
#1066=CONICAL_SURFACE('',#18736,1.61,0.959931088596875);
#1067=CONICAL_SURFACE('',#18741,2.,0.959931088596884);
#1068=CONICAL_SURFACE('',#18745,1.61,0.959931088596875);
#1069=CONICAL_SURFACE('',#18750,2.,0.959931088596884);
#1070=CONICAL_SURFACE('',#18754,1.61,0.959931088596875);
#1071=CONICAL_SURFACE('',#18759,2.,0.959931088596884);
#1072=CONICAL_SURFACE('',#18763,1.61,0.959931088596875);
#1073=CONICAL_SURFACE('',#18768,2.,0.959931088596884);
#1074=CONICAL_SURFACE('',#18772,1.61,0.959931088596875);
#1075=CONICAL_SURFACE('',#18777,2.,0.959931088596884);
#1076=CONICAL_SURFACE('',#18781,1.61,0.959931088596875);
#1077=CONICAL_SURFACE('',#18786,2.,0.959931088596884);
#1078=CONICAL_SURFACE('',#18790,1.61,0.959931088596875);
#1079=CONICAL_SURFACE('',#18795,2.,0.959931088596884);
#1080=CONICAL_SURFACE('',#18796,8.175,0.785398163397451);
#1081=CONICAL_SURFACE('',#18875,8.175,0.785398163397451);
#1082=CONICAL_SURFACE('',#19198,2.64252040565333,0.0872664625997168);
#1083=CONICAL_SURFACE('',#19214,2.,0.785398163397446);
#1084=CONICAL_SURFACE('',#19218,1.61,0.959931088596878);
#1085=CONICAL_SURFACE('',#19223,2.,0.959931088596884);
#1086=CONICAL_SURFACE('',#19227,1.61,0.959931088596878);
#1087=CONICAL_SURFACE('',#19232,2.,0.959931088596884);
#1088=CONICAL_SURFACE('',#19236,1.61,0.959931088596878);
#1089=CONICAL_SURFACE('',#19241,2.,0.959931088596884);
#1090=CONICAL_SURFACE('',#19245,1.61,0.959931088596878);
#1091=CONICAL_SURFACE('',#19250,2.,0.959931088596884);
#1092=CONICAL_SURFACE('',#19254,1.61,0.959931088596878);
#1093=CONICAL_SURFACE('',#19259,2.,0.959931088596884);
#1094=CONICAL_SURFACE('',#19263,1.61,0.959931088596878);
#1095=CONICAL_SURFACE('',#19268,2.,0.959931088596884);
#1096=CONICAL_SURFACE('',#19272,1.61,0.959931088596878);
#1097=CONICAL_SURFACE('',#19277,2.,0.959931088596884);
#1098=CONICAL_SURFACE('',#19281,1.61,0.959931088596878);
#1099=CONICAL_SURFACE('',#19286,2.,0.959931088596884);
#1100=CONICAL_SURFACE('',#19290,1.61,0.959931088596878);
#1101=CONICAL_SURFACE('',#19295,2.,0.959931088596884);
#1102=CONICAL_SURFACE('',#19299,1.61,0.959931088596878);
#1103=CONICAL_SURFACE('',#19304,2.,0.959931088596884);
#1104=CONICAL_SURFACE('',#19308,1.61,0.959931088596878);
#1105=CONICAL_SURFACE('',#19313,2.,0.959931088596884);
#1106=CONICAL_SURFACE('',#19317,1.61,0.959931088596878);
#1107=CONICAL_SURFACE('',#19322,2.,0.959931088596884);
#1108=CONICAL_SURFACE('',#19326,1.61,0.959931088596878);
#1109=CONICAL_SURFACE('',#19331,2.,0.959931088596884);
#1110=CONICAL_SURFACE('',#19334,8.175,0.785398163397449);
#1111=CONICAL_SURFACE('',#19413,8.175,0.785398163397449);
#1125=SHAPE_REPRESENTATION_RELATIONSHIP('SRR','None',#38698,#1139);
#1139=ADVANCED_BREP_SHAPE_REPRESENTATION('',(#1185,#1186,#1187,#1188,#1189,
#1190,#1191),#38634);
#1159=STYLED_ITEM('',(#38765),#1185);
#1160=STYLED_ITEM('',(#38765),#1186);
#1161=STYLED_ITEM('',(#38765),#1187);
#1162=STYLED_ITEM('',(#38765),#1188);
#1163=STYLED_ITEM('',(#38765),#1189);
#1164=STYLED_ITEM('',(#38765),#1190);
#1165=STYLED_ITEM('',(#38765),#1191);
#1185=MANIFOLD_SOLID_BREP('Body1',#17625);
#1186=MANIFOLD_SOLID_BREP('Body2',#17626);
#1187=MANIFOLD_SOLID_BREP('Body3',#17627);
#1188=MANIFOLD_SOLID_BREP('Body4',#17628);
#1189=MANIFOLD_SOLID_BREP('Body5',#17629);
#1190=MANIFOLD_SOLID_BREP('Body6',#17630);
#1191=MANIFOLD_SOLID_BREP('Body7',#17631);
#1279=PLANE('',#18491);
#1280=PLANE('',#18492);
#1281=PLANE('',#18493);
#1282=PLANE('',#18496);
#1283=PLANE('',#18497);
#1284=PLANE('',#18500);
#1285=PLANE('',#18501);
#1286=PLANE('',#18502);
#1287=PLANE('',#18504);
#1288=PLANE('',#18509);
#1289=PLANE('',#18510);
#1290=PLANE('',#18514);
#1291=PLANE('',#18515);
#1292=PLANE('',#18516);
#1293=PLANE('',#18517);
#1294=PLANE('',#18518);
#1295=PLANE('',#18519);
#1296=PLANE('',#18520);
#1297=PLANE('',#18522);
#1298=PLANE('',#18523);
#1299=PLANE('',#18524);
#1300=PLANE('',#18527);
#1301=PLANE('',#18529);
#1302=PLANE('',#18608);
#1303=PLANE('',#18609);
#1304=PLANE('',#18630);
#1305=PLANE('',#18634);
#1306=PLANE('',#18635);
#1307=PLANE('',#18636);
#1308=PLANE('',#18638);
#1309=PLANE('',#18639);
#1310=PLANE('',#18642);
#1311=PLANE('',#18643);
#1312=PLANE('',#18644);
#1313=PLANE('',#18645);
#1314=PLANE('',#18646);
#1315=PLANE('',#18647);
#1316=PLANE('',#18648);
#1317=PLANE('',#18649);
#1318=PLANE('',#18655);
#1319=PLANE('',#19031);
#1320=PLANE('',#19033);
#1321=PLANE('',#19034);
#1322=PLANE('',#19035);
#1323=PLANE('',#19036);
#1324=PLANE('',#19037);
#1325=PLANE('',#19038);
#1326=PLANE('',#19039);
#1327=PLANE('',#19040);
#1328=PLANE('',#19041);
#1329=PLANE('',#19042);
#1330=PLANE('',#19043);
#1331=PLANE('',#19044);
#1332=PLANE('',#19045);
#1333=PLANE('',#19046);
#1334=PLANE('',#19047);
#1335=PLANE('',#19048);
#1336=PLANE('',#19049);
#1337=PLANE('',#19050);
#1338=PLANE('',#19051);
#1339=PLANE('',#19052);
#1340=PLANE('',#19053);
#1341=PLANE('',#19054);
#1342=PLANE('',#19055);
#1343=PLANE('',#19056);
#1344=PLANE('',#19057);
#1345=PLANE('',#19058);
#1346=PLANE('',#19059);
#1347=PLANE('',#19060);
#1348=PLANE('',#19061);
#1349=PLANE('',#19062);
#1350=PLANE('',#19063);
#1351=PLANE('',#19064);
#1352=PLANE('',#19065);
#1353=PLANE('',#19066);
#1354=PLANE('',#19067);
#1355=PLANE('',#19068);
#1356=PLANE('',#19069);
#1357=PLANE('',#19070);
#1358=PLANE('',#19071);
#1359=PLANE('',#19072);
#1360=PLANE('',#19073);
#1361=PLANE('',#19074);
#1362=PLANE('',#19075);
#1363=PLANE('',#19076);
#1364=PLANE('',#19077);
#1365=PLANE('',#19078);
#1366=PLANE('',#19079);
#1367=PLANE('',#19080);
#1368=PLANE('',#19081);
#1369=PLANE('',#19082);
#1370=PLANE('',#19083);
#1371=PLANE('',#19084);
#1372=PLANE('',#19085);
#1373=PLANE('',#19086);
#1374=PLANE('',#19087);
#1375=PLANE('',#19088);
#1376=PLANE('',#19089);
#1377=PLANE('',#19090);
#1378=PLANE('',#19091);
#1379=PLANE('',#19092);
#1380=PLANE('',#19093);
#1381=PLANE('',#19094);
#1382=PLANE('',#19095);
#1383=PLANE('',#19096);
#1384=PLANE('',#19097);
#1385=PLANE('',#19098);
#1386=PLANE('',#19099);
#1387=PLANE('',#19100);
#1388=PLANE('',#19101);
#1389=PLANE('',#19102);
#1390=PLANE('',#19103);
#1391=PLANE('',#19104);
#1392=PLANE('',#19105);
#1393=PLANE('',#19106);
#1394=PLANE('',#19107);
#1395=PLANE('',#19108);
#1396=PLANE('',#19109);
#1397=PLANE('',#19110);
#1398=PLANE('',#19111);
#1399=PLANE('',#19112);
#1400=PLANE('',#19113);
#1401=PLANE('',#19114);
#1402=PLANE('',#19115);
#1403=PLANE('',#19116);
#1404=PLANE('',#19117);
#1405=PLANE('',#19118);
#1406=PLANE('',#19119);
#1407=PLANE('',#19120);
#1408=PLANE('',#19121);
#1409=PLANE('',#19122);
#1410=PLANE('',#19123);
#1411=PLANE('',#19124);
#1412=PLANE('',#19125);
#1413=PLANE('',#19126);
#1414=PLANE('',#19127);
#1415=PLANE('',#19128);
#1416=PLANE('',#19129);
#1417=PLANE('',#19130);
#1418=PLANE('',#19131);
#1419=PLANE('',#19132);
#1420=PLANE('',#19133);
#1421=PLANE('',#19134);
#1422=PLANE('',#19135);
#1423=PLANE('',#19136);
#1424=PLANE('',#19137);
#1425=PLANE('',#19138);
#1426=PLANE('',#19139);
#1427=PLANE('',#19140);
#1428=PLANE('',#19141);
#1429=PLANE('',#19142);
#1430=PLANE('',#19143);
#1431=PLANE('',#19144);
#1432=PLANE('',#19145);
#1433=PLANE('',#19146);
#1434=PLANE('',#19147);
#1435=PLANE('',#19148);
#1436=PLANE('',#19149);
#1437=PLANE('',#19150);
#1438=PLANE('',#19151);
#1439=PLANE('',#19152);
#1440=PLANE('',#19153);
#1441=PLANE('',#19154);
#1442=PLANE('',#19155);
#1443=PLANE('',#19156);
#1444=PLANE('',#19157);
#1445=PLANE('',#19158);
#1446=PLANE('',#19159);
#1447=PLANE('',#19160);
#1448=PLANE('',#19161);
#1449=PLANE('',#19162);
#1450=PLANE('',#19163);
#1451=PLANE('',#19164);
#1452=PLANE('',#19165);
#1453=PLANE('',#19166);
#1454=PLANE('',#19167);
#1455=PLANE('',#19168);
#1456=PLANE('',#19169);
#1457=PLANE('',#19170);
#1458=PLANE('',#19171);
#1459=PLANE('',#19172);
#1460=PLANE('',#19173);
#1461=PLANE('',#19174);
#1462=PLANE('',#19175);
#1463=PLANE('',#19176);
#1464=PLANE('',#19177);
#1465=PLANE('',#19178);
#1466=PLANE('',#19179);
#1467=PLANE('',#19180);
#1468=PLANE('',#19181);
#1469=PLANE('',#19182);
#1470=PLANE('',#19183);
#1471=PLANE('',#19184);
#1472=PLANE('',#19185);
#1473=PLANE('',#19186);
#1474=PLANE('',#19187);
#1475=PLANE('',#19188);
#1476=PLANE('',#19203);
#1477=PLANE('',#19204);
#1478=PLANE('',#19205);
#1479=PLANE('',#19206);
#1480=PLANE('',#19207);
#1481=PLANE('',#19208);
#1482=PLANE('',#19209);
#1483=PLANE('',#19570);
#1484=PLANE('',#19572);
#1485=PLANE('',#19573);
#1486=PLANE('',#19574);
#1487=PLANE('',#19575);
#1488=PLANE('',#19576);
#1489=PLANE('',#19577);
#1490=PLANE('',#19578);
#1491=PLANE('',#19579);
#1492=PLANE('',#19580);
#1493=PLANE('',#19581);
#1494=PLANE('',#19582);
#1495=PLANE('',#19583);
#1496=PLANE('',#19584);
#1497=PLANE('',#19585);
#1498=PLANE('',#19586);
#1499=PLANE('',#19587);
#1500=PLANE('',#19588);
#1501=PLANE('',#19589);
#1502=PLANE('',#19590);
#1503=PLANE('',#19591);
#1504=PLANE('',#19592);
#1505=PLANE('',#19593);
#1506=PLANE('',#19594);
#1507=PLANE('',#19595);
#1508=PLANE('',#19596);
#1509=PLANE('',#19597);
#1510=PLANE('',#19598);
#1511=PLANE('',#19599);
#1512=PLANE('',#19600);
#1513=PLANE('',#19601);
#1514=PLANE('',#19602);
#1515=PLANE('',#19603);
#1516=PLANE('',#19604);
#1517=PLANE('',#19605);
#1518=PLANE('',#19606);
#1519=PLANE('',#19607);
#1520=PLANE('',#19608);
#1521=PLANE('',#19609);
#1522=PLANE('',#19610);
#1523=PLANE('',#19611);
#1524=PLANE('',#19612);
#1525=PLANE('',#19613);
#1526=PLANE('',#19614);
#1527=PLANE('',#19615);
#1528=PLANE('',#19616);
#1529=PLANE('',#19617);
#1530=PLANE('',#19618);
#1531=PLANE('',#19619);
#1532=PLANE('',#19620);
#1533=PLANE('',#19621);
#1534=PLANE('',#19622);
#1535=PLANE('',#19623);
#1536=PLANE('',#19624);
#1537=PLANE('',#19625);
#1538=PLANE('',#19626);
#1539=PLANE('',#19627);
#1540=PLANE('',#19628);
#1541=PLANE('',#19629);
#1542=PLANE('',#19630);
#1543=PLANE('',#19631);
#1544=PLANE('',#19632);
#1545=PLANE('',#19633);
#1546=PLANE('',#19634);
#1547=PLANE('',#19635);
#1548=PLANE('',#19636);
#1549=PLANE('',#19637);
#1550=PLANE('',#19638);
#1551=PLANE('',#19639);
#1552=PLANE('',#19640);
#1553=PLANE('',#19641);
#1554=PLANE('',#19642);
#1555=PLANE('',#19643);
#1556=PLANE('',#19644);
#1557=PLANE('',#19645);
#1558=PLANE('',#19646);
#1559=PLANE('',#19647);
#1560=PLANE('',#19648);
#1561=PLANE('',#19649);
#1562=PLANE('',#19650);
#1563=PLANE('',#19651);
#1564=PLANE('',#19652);
#1565=PLANE('',#19653);
#1566=PLANE('',#19654);
#1567=PLANE('',#19655);
#1568=PLANE('',#19656);
#1569=PLANE('',#19657);
#1570=PLANE('',#19658);
#1571=PLANE('',#19659);
#1572=PLANE('',#19660);
#1573=PLANE('',#19661);
#1574=PLANE('',#19662);
#1575=PLANE('',#19663);
#1576=PLANE('',#19664);
#1577=PLANE('',#19665);
#1578=PLANE('',#19666);
#1579=PLANE('',#19667);
#1580=PLANE('',#19668);
#1581=PLANE('',#19669);
#1582=PLANE('',#19670);
#1583=PLANE('',#19671);
#1584=PLANE('',#19672);
#1585=PLANE('',#19673);
#1586=PLANE('',#19674);
#1587=PLANE('',#19675);
#1588=PLANE('',#19676);
#1589=PLANE('',#19677);
#1590=PLANE('',#19678);
#1591=PLANE('',#19679);
#1592=PLANE('',#19680);
#1593=PLANE('',#19681);
#1594=PLANE('',#19682);
#1595=PLANE('',#19683);
#1596=PLANE('',#19684);
#1597=PLANE('',#19685);
#1598=PLANE('',#19686);
#1599=PLANE('',#19687);
#1600=PLANE('',#19688);
#1601=PLANE('',#19689);
#1602=PLANE('',#19690);
#1603=PLANE('',#19691);
#1604=PLANE('',#19692);
#1605=PLANE('',#19693);
#1606=PLANE('',#19694);
#1607=PLANE('',#19695);
#1608=PLANE('',#19696);
#1609=PLANE('',#19697);
#1610=PLANE('',#19698);
#1611=PLANE('',#19699);
#1612=PLANE('',#19700);
#1613=PLANE('',#19701);
#1614=PLANE('',#19702);
#1615=PLANE('',#19703);
#1616=PLANE('',#19704);
#1617=PLANE('',#19705);
#1618=PLANE('',#19706);
#1619=PLANE('',#19707);
#1620=PLANE('',#19708);
#1621=PLANE('',#19709);
#1622=PLANE('',#19710);
#1623=PLANE('',#19711);
#1624=PLANE('',#19712);
#1625=PLANE('',#19713);
#1626=PLANE('',#19714);
#1627=PLANE('',#19715);
#1628=PLANE('',#19716);
#1629=PLANE('',#19717);
#1630=PLANE('',#19718);
#1631=PLANE('',#19719);
#1632=PLANE('',#19720);
#1633=PLANE('',#19721);
#1634=PLANE('',#19722);
#1635=PLANE('',#19723);
#1636=PLANE('',#19724);
#1637=PLANE('',#19725);
#1638=PLANE('',#19726);
#1639=PLANE('',#19727);
#1640=PLANE('',#19728);
#1969=FACE_OUTER_BOUND('',#2998,.T.);
#1970=FACE_OUTER_BOUND('',#2999,.T.);
#1971=FACE_OUTER_BOUND('',#3000,.T.);
#1972=FACE_OUTER_BOUND('',#3001,.T.);
#1973=FACE_OUTER_BOUND('',#3002,.T.);
#1974=FACE_OUTER_BOUND('',#3003,.T.);
#1975=FACE_OUTER_BOUND('',#3004,.T.);
#1976=FACE_OUTER_BOUND('',#3005,.T.);
#1977=FACE_OUTER_BOUND('',#3006,.T.);
#1978=FACE_OUTER_BOUND('',#3007,.T.);
#1979=FACE_OUTER_BOUND('',#3008,.T.);
#1980=FACE_OUTER_BOUND('',#3009,.T.);
#1981=FACE_OUTER_BOUND('',#3010,.T.);
#1982=FACE_OUTER_BOUND('',#3011,.T.);
#1983=FACE_OUTER_BOUND('',#3012,.T.);
#1984=FACE_OUTER_BOUND('',#3013,.T.);
#1985=FACE_OUTER_BOUND('',#3014,.T.);
#1986=FACE_OUTER_BOUND('',#3015,.T.);
#1987=FACE_OUTER_BOUND('',#3016,.T.);
#1988=FACE_OUTER_BOUND('',#3019,.T.);
#1989=FACE_OUTER_BOUND('',#3020,.T.);
#1990=FACE_OUTER_BOUND('',#3021,.T.);
#1991=FACE_OUTER_BOUND('',#3022,.T.);
#1992=FACE_OUTER_BOUND('',#3025,.T.);
#1993=FACE_OUTER_BOUND('',#3027,.T.);
#1994=FACE_OUTER_BOUND('',#3029,.T.);
#1995=FACE_OUTER_BOUND('',#3030,.T.);
#1996=FACE_OUTER_BOUND('',#3031,.T.);
#1997=FACE_OUTER_BOUND('',#3033,.T.);
#1998=FACE_OUTER_BOUND('',#3034,.T.);
#1999=FACE_OUTER_BOUND('',#3035,.T.);
#2000=FACE_OUTER_BOUND('',#3036,.T.);
#2001=FACE_OUTER_BOUND('',#3037,.T.);
#2002=FACE_OUTER_BOUND('',#3038,.T.);
#2003=FACE_OUTER_BOUND('',#3039,.T.);
#2004=FACE_OUTER_BOUND('',#3040,.T.);
#2005=FACE_OUTER_BOUND('',#3042,.T.);
#2006=FACE_OUTER_BOUND('',#3043,.T.);
#2007=FACE_OUTER_BOUND('',#3044,.T.);
#2008=FACE_OUTER_BOUND('',#3045,.T.);
#2009=FACE_OUTER_BOUND('',#3046,.T.);
#2010=FACE_OUTER_BOUND('',#3048,.T.);
#2011=FACE_OUTER_BOUND('',#3049,.T.);
#2012=FACE_OUTER_BOUND('',#3050,.T.);
#2013=FACE_OUTER_BOUND('',#3051,.T.);
#2014=FACE_OUTER_BOUND('',#3052,.T.);
#2015=FACE_OUTER_BOUND('',#3053,.T.);
#2016=FACE_OUTER_BOUND('',#3054,.T.);
#2017=FACE_OUTER_BOUND('',#3055,.T.);
#2018=FACE_OUTER_BOUND('',#3056,.T.);
#2019=FACE_OUTER_BOUND('',#3057,.T.);
#2020=FACE_OUTER_BOUND('',#3058,.T.);
#2021=FACE_OUTER_BOUND('',#3059,.T.);
#2022=FACE_OUTER_BOUND('',#3060,.T.);
#2023=FACE_OUTER_BOUND('',#3061,.T.);
#2024=FACE_OUTER_BOUND('',#3062,.T.);
#2025=FACE_OUTER_BOUND('',#3063,.T.);
#2026=FACE_OUTER_BOUND('',#3064,.T.);
#2027=FACE_OUTER_BOUND('',#3065,.T.);
#2028=FACE_OUTER_BOUND('',#3066,.T.);
#2029=FACE_OUTER_BOUND('',#3067,.T.);
#2030=FACE_OUTER_BOUND('',#3068,.T.);
#2031=FACE_OUTER_BOUND('',#3069,.T.);
#2032=FACE_OUTER_BOUND('',#3070,.T.);
#2033=FACE_OUTER_BOUND('',#3071,.T.);
#2034=FACE_OUTER_BOUND('',#3072,.T.);
#2035=FACE_OUTER_BOUND('',#3073,.T.);
#2036=FACE_OUTER_BOUND('',#3074,.T.);
#2037=FACE_OUTER_BOUND('',#3075,.T.);
#2038=FACE_OUTER_BOUND('',#3076,.T.);
#2039=FACE_OUTER_BOUND('',#3077,.T.);
#2040=FACE_OUTER_BOUND('',#3078,.T.);
#2041=FACE_OUTER_BOUND('',#3079,.T.);
#2042=FACE_OUTER_BOUND('',#3080,.T.);
#2043=FACE_OUTER_BOUND('',#3081,.T.);
#2044=FACE_OUTER_BOUND('',#3082,.T.);
#2045=FACE_OUTER_BOUND('',#3083,.T.);
#2046=FACE_OUTER_BOUND('',#3084,.T.);
#2047=FACE_OUTER_BOUND('',#3085,.T.);
#2048=FACE_OUTER_BOUND('',#3086,.T.);
#2049=FACE_OUTER_BOUND('',#3087,.T.);
#2050=FACE_OUTER_BOUND('',#3088,.T.);
#2051=FACE_OUTER_BOUND('',#3089,.T.);
#2052=FACE_OUTER_BOUND('',#3090,.T.);
#2053=FACE_OUTER_BOUND('',#3091,.T.);
#2054=FACE_OUTER_BOUND('',#3092,.T.);
#2055=FACE_OUTER_BOUND('',#3093,.T.);
#2056=FACE_OUTER_BOUND('',#3094,.T.);
#2057=FACE_OUTER_BOUND('',#3095,.T.);
#2058=FACE_OUTER_BOUND('',#3096,.T.);
#2059=FACE_OUTER_BOUND('',#3097,.T.);
#2060=FACE_OUTER_BOUND('',#3099,.T.);
#2061=FACE_OUTER_BOUND('',#3101,.T.);
#2062=FACE_OUTER_BOUND('',#3102,.T.);
#2063=FACE_OUTER_BOUND('',#3104,.T.);
#2064=FACE_OUTER_BOUND('',#3105,.T.);
#2065=FACE_OUTER_BOUND('',#3106,.T.);
#2066=FACE_OUTER_BOUND('',#3108,.T.);
#2067=FACE_OUTER_BOUND('',#3110,.T.);
#2068=FACE_OUTER_BOUND('',#3112,.T.);
#2069=FACE_OUTER_BOUND('',#3113,.T.);
#2070=FACE_OUTER_BOUND('',#3115,.T.);
#2071=FACE_OUTER_BOUND('',#3117,.T.);
#2072=FACE_OUTER_BOUND('',#3118,.T.);
#2073=FACE_OUTER_BOUND('',#3119,.T.);
#2074=FACE_OUTER_BOUND('',#3121,.T.);
#2075=FACE_OUTER_BOUND('',#3122,.T.);
#2076=FACE_OUTER_BOUND('',#3123,.T.);
#2077=FACE_OUTER_BOUND('',#3124,.T.);
#2078=FACE_OUTER_BOUND('',#3125,.T.);
#2079=FACE_OUTER_BOUND('',#3126,.T.);
#2080=FACE_OUTER_BOUND('',#3127,.T.);
#2081=FACE_OUTER_BOUND('',#3128,.T.);
#2082=FACE_OUTER_BOUND('',#3129,.T.);
#2083=FACE_OUTER_BOUND('',#3130,.T.);
#2084=FACE_OUTER_BOUND('',#3131,.T.);
#2085=FACE_OUTER_BOUND('',#3132,.T.);
#2086=FACE_OUTER_BOUND('',#3133,.T.);
#2087=FACE_OUTER_BOUND('',#3134,.T.);
#2088=FACE_OUTER_BOUND('',#3135,.T.);
#2089=FACE_OUTER_BOUND('',#3136,.T.);
#2090=FACE_OUTER_BOUND('',#3137,.T.);
#2091=FACE_OUTER_BOUND('',#3138,.T.);
#2092=FACE_OUTER_BOUND('',#3139,.T.);
#2093=FACE_OUTER_BOUND('',#3140,.T.);
#2094=FACE_OUTER_BOUND('',#3141,.T.);
#2095=FACE_OUTER_BOUND('',#3142,.T.);
#2096=FACE_OUTER_BOUND('',#3143,.T.);
#2097=FACE_OUTER_BOUND('',#3144,.T.);
#2098=FACE_OUTER_BOUND('',#3145,.T.);
#2099=FACE_OUTER_BOUND('',#3146,.T.);
#2100=FACE_OUTER_BOUND('',#3147,.T.);
#2101=FACE_OUTER_BOUND('',#3148,.T.);
#2102=FACE_OUTER_BOUND('',#3149,.T.);
#2103=FACE_OUTER_BOUND('',#3150,.T.);
#2104=FACE_OUTER_BOUND('',#3151,.T.);
#2105=FACE_OUTER_BOUND('',#3152,.T.);
#2106=FACE_OUTER_BOUND('',#3153,.T.);
#2107=FACE_OUTER_BOUND('',#3154,.T.);
#2108=FACE_OUTER_BOUND('',#3155,.T.);
#2109=FACE_OUTER_BOUND('',#3156,.T.);
#2110=FACE_OUTER_BOUND('',#3157,.T.);
#2111=FACE_OUTER_BOUND('',#3158,.T.);
#2112=FACE_OUTER_BOUND('',#3159,.T.);
#2113=FACE_OUTER_BOUND('',#3160,.T.);
#2114=FACE_OUTER_BOUND('',#3161,.T.);
#2115=FACE_OUTER_BOUND('',#3162,.T.);
#2116=FACE_OUTER_BOUND('',#3163,.T.);
#2117=FACE_OUTER_BOUND('',#3164,.T.);
#2118=FACE_OUTER_BOUND('',#3165,.T.);
#2119=FACE_OUTER_BOUND('',#3166,.T.);
#2120=FACE_OUTER_BOUND('',#3167,.T.);
#2121=FACE_OUTER_BOUND('',#3168,.T.);
#2122=FACE_OUTER_BOUND('',#3169,.T.);
#2123=FACE_OUTER_BOUND('',#3170,.T.);
#2124=FACE_OUTER_BOUND('',#3171,.T.);
#2125=FACE_OUTER_BOUND('',#3172,.T.);
#2126=FACE_OUTER_BOUND('',#3173,.T.);
#2127=FACE_OUTER_BOUND('',#3174,.T.);
#2128=FACE_OUTER_BOUND('',#3175,.T.);
#2129=FACE_OUTER_BOUND('',#3176,.T.);
#2130=FACE_OUTER_BOUND('',#3177,.T.);
#2131=FACE_OUTER_BOUND('',#3178,.T.);
#2132=FACE_OUTER_BOUND('',#3179,.T.);
#2133=FACE_OUTER_BOUND('',#3180,.T.);
#2134=FACE_OUTER_BOUND('',#3181,.T.);
#2135=FACE_OUTER_BOUND('',#3182,.T.);
#2136=FACE_OUTER_BOUND('',#3183,.T.);
#2137=FACE_OUTER_BOUND('',#3184,.T.);
#2138=FACE_OUTER_BOUND('',#3185,.T.);
#2139=FACE_OUTER_BOUND('',#3186,.T.);
#2140=FACE_OUTER_BOUND('',#3187,.T.);
#2141=FACE_OUTER_BOUND('',#3188,.T.);
#2142=FACE_OUTER_BOUND('',#3189,.T.);
#2143=FACE_OUTER_BOUND('',#3190,.T.);
#2144=FACE_OUTER_BOUND('',#3191,.T.);
#2145=FACE_OUTER_BOUND('',#3192,.T.);
#2146=FACE_OUTER_BOUND('',#3193,.T.);
#2147=FACE_OUTER_BOUND('',#3194,.T.);
#2148=FACE_OUTER_BOUND('',#3195,.T.);
#2149=FACE_OUTER_BOUND('',#3196,.T.);
#2150=FACE_OUTER_BOUND('',#3197,.T.);
#2151=FACE_OUTER_BOUND('',#3198,.T.);
#2152=FACE_OUTER_BOUND('',#3199,.T.);
#2153=FACE_OUTER_BOUND('',#3200,.T.);
#2154=FACE_OUTER_BOUND('',#3201,.T.);
#2155=FACE_OUTER_BOUND('',#3202,.T.);
#2156=FACE_OUTER_BOUND('',#3203,.T.);
#2157=FACE_OUTER_BOUND('',#3204,.T.);
#2158=FACE_OUTER_BOUND('',#3205,.T.);
#2159=FACE_OUTER_BOUND('',#3206,.T.);
#2160=FACE_OUTER_BOUND('',#3207,.T.);
#2161=FACE_OUTER_BOUND('',#3208,.T.);
#2162=FACE_OUTER_BOUND('',#3209,.T.);
#2163=FACE_OUTER_BOUND('',#3210,.T.);
#2164=FACE_OUTER_BOUND('',#3211,.T.);
#2165=FACE_OUTER_BOUND('',#3212,.T.);
#2166=FACE_OUTER_BOUND('',#3213,.T.);
#2167=FACE_OUTER_BOUND('',#3214,.T.);
#2168=FACE_OUTER_BOUND('',#3215,.T.);
#2169=FACE_OUTER_BOUND('',#3216,.T.);
#2170=FACE_OUTER_BOUND('',#3217,.T.);
#2171=FACE_OUTER_BOUND('',#3218,.T.);
#2172=FACE_OUTER_BOUND('',#3219,.T.);
#2173=FACE_OUTER_BOUND('',#3220,.T.);
#2174=FACE_OUTER_BOUND('',#3221,.T.);
#2175=FACE_OUTER_BOUND('',#3222,.T.);
#2176=FACE_OUTER_BOUND('',#3223,.T.);
#2177=FACE_OUTER_BOUND('',#3224,.T.);
#2178=FACE_OUTER_BOUND('',#3225,.T.);
#2179=FACE_OUTER_BOUND('',#3226,.T.);
#2180=FACE_OUTER_BOUND('',#3227,.T.);
#2181=FACE_OUTER_BOUND('',#3228,.T.);
#2182=FACE_OUTER_BOUND('',#3229,.T.);
#2183=FACE_OUTER_BOUND('',#3230,.T.);
#2184=FACE_OUTER_BOUND('',#3231,.T.);
#2185=FACE_OUTER_BOUND('',#3232,.T.);
#2186=FACE_OUTER_BOUND('',#3233,.T.);
#2187=FACE_OUTER_BOUND('',#3234,.T.);
#2188=FACE_OUTER_BOUND('',#3235,.T.);
#2189=FACE_OUTER_BOUND('',#3236,.T.);
#2190=FACE_OUTER_BOUND('',#3237,.T.);
#2191=FACE_OUTER_BOUND('',#3238,.T.);
#2192=FACE_OUTER_BOUND('',#3239,.T.);
#2193=FACE_OUTER_BOUND('',#3240,.T.);
#2194=FACE_OUTER_BOUND('',#3241,.T.);
#2195=FACE_OUTER_BOUND('',#3242,.T.);
#2196=FACE_OUTER_BOUND('',#3243,.T.);
#2197=FACE_OUTER_BOUND('',#3244,.T.);
#2198=FACE_OUTER_BOUND('',#3245,.T.);
#2199=FACE_OUTER_BOUND('',#3246,.T.);
#2200=FACE_OUTER_BOUND('',#3247,.T.);
#2201=FACE_OUTER_BOUND('',#3249,.T.);
#2202=FACE_OUTER_BOUND('',#3250,.T.);
#2203=FACE_OUTER_BOUND('',#3251,.T.);
#2204=FACE_OUTER_BOUND('',#3252,.T.);
#2205=FACE_OUTER_BOUND('',#3253,.T.);
#2206=FACE_OUTER_BOUND('',#3254,.T.);
#2207=FACE_OUTER_BOUND('',#3255,.T.);
#2208=FACE_OUTER_BOUND('',#3256,.T.);
#2209=FACE_OUTER_BOUND('',#3257,.T.);
#2210=FACE_OUTER_BOUND('',#3258,.T.);
#2211=FACE_OUTER_BOUND('',#3259,.T.);
#2212=FACE_OUTER_BOUND('',#3260,.T.);
#2213=FACE_OUTER_BOUND('',#3261,.T.);
#2214=FACE_OUTER_BOUND('',#3262,.T.);
#2215=FACE_OUTER_BOUND('',#3263,.T.);
#2216=FACE_OUTER_BOUND('',#3264,.T.);
#2217=FACE_OUTER_BOUND('',#3265,.T.);
#2218=FACE_OUTER_BOUND('',#3266,.T.);
#2219=FACE_OUTER_BOUND('',#3267,.T.);
#2220=FACE_OUTER_BOUND('',#3268,.T.);
#2221=FACE_OUTER_BOUND('',#3269,.T.);
#2222=FACE_OUTER_BOUND('',#3270,.T.);
#2223=FACE_OUTER_BOUND('',#3271,.T.);
#2224=FACE_OUTER_BOUND('',#3272,.T.);
#2225=FACE_OUTER_BOUND('',#3273,.T.);
#2226=FACE_OUTER_BOUND('',#3274,.T.);
#2227=FACE_OUTER_BOUND('',#3275,.T.);
#2228=FACE_OUTER_BOUND('',#3276,.T.);
#2229=FACE_OUTER_BOUND('',#3277,.T.);
#2230=FACE_OUTER_BOUND('',#3278,.T.);
#2231=FACE_OUTER_BOUND('',#3279,.T.);
#2232=FACE_OUTER_BOUND('',#3280,.T.);
#2233=FACE_OUTER_BOUND('',#3281,.T.);
#2234=FACE_OUTER_BOUND('',#3282,.T.);
#2235=FACE_OUTER_BOUND('',#3283,.T.);
#2236=FACE_OUTER_BOUND('',#3284,.T.);
#2237=FACE_OUTER_BOUND('',#3285,.T.);
#2238=FACE_OUTER_BOUND('',#3286,.T.);
#2239=FACE_OUTER_BOUND('',#3287,.T.);
#2240=FACE_OUTER_BOUND('',#3288,.T.);
#2241=FACE_OUTER_BOUND('',#3289,.T.);
#2242=FACE_OUTER_BOUND('',#3290,.T.);
#2243=FACE_OUTER_BOUND('',#3291,.T.);
#2244=FACE_OUTER_BOUND('',#3292,.T.);
#2245=FACE_OUTER_BOUND('',#3293,.T.);
#2246=FACE_OUTER_BOUND('',#3294,.T.);
#2247=FACE_OUTER_BOUND('',#3295,.T.);
#2248=FACE_OUTER_BOUND('',#3296,.T.);
#2249=FACE_OUTER_BOUND('',#3297,.T.);
#2250=FACE_OUTER_BOUND('',#3298,.T.);
#2251=FACE_OUTER_BOUND('',#3299,.T.);
#2252=FACE_OUTER_BOUND('',#3300,.T.);
#2253=FACE_OUTER_BOUND('',#3301,.T.);
#2254=FACE_OUTER_BOUND('',#3302,.T.);
#2255=FACE_OUTER_BOUND('',#3303,.T.);
#2256=FACE_OUTER_BOUND('',#3304,.T.);
#2257=FACE_OUTER_BOUND('',#3305,.T.);
#2258=FACE_OUTER_BOUND('',#3306,.T.);
#2259=FACE_OUTER_BOUND('',#3307,.T.);
#2260=FACE_OUTER_BOUND('',#3308,.T.);
#2261=FACE_OUTER_BOUND('',#3309,.T.);
#2262=FACE_OUTER_BOUND('',#3310,.T.);
#2263=FACE_OUTER_BOUND('',#3311,.T.);
#2264=FACE_OUTER_BOUND('',#3312,.T.);
#2265=FACE_OUTER_BOUND('',#3313,.T.);
#2266=FACE_OUTER_BOUND('',#3314,.T.);
#2267=FACE_OUTER_BOUND('',#3315,.T.);
#2268=FACE_OUTER_BOUND('',#3316,.T.);
#2269=FACE_OUTER_BOUND('',#3317,.T.);
#2270=FACE_OUTER_BOUND('',#3318,.T.);
#2271=FACE_OUTER_BOUND('',#3319,.T.);
#2272=FACE_OUTER_BOUND('',#3320,.T.);
#2273=FACE_OUTER_BOUND('',#3321,.T.);
#2274=FACE_OUTER_BOUND('',#3322,.T.);
#2275=FACE_OUTER_BOUND('',#3323,.T.);
#2276=FACE_OUTER_BOUND('',#3324,.T.);
#2277=FACE_OUTER_BOUND('',#3325,.T.);
#2278=FACE_OUTER_BOUND('',#3326,.T.);
#2279=FACE_OUTER_BOUND('',#3327,.T.);
#2280=FACE_OUTER_BOUND('',#3328,.T.);
#2281=FACE_OUTER_BOUND('',#3329,.T.);
#2282=FACE_OUTER_BOUND('',#3330,.T.);
#2283=FACE_OUTER_BOUND('',#3331,.T.);
#2284=FACE_OUTER_BOUND('',#3332,.T.);
#2285=FACE_OUTER_BOUND('',#3333,.T.);
#2286=FACE_OUTER_BOUND('',#3334,.T.);
#2287=FACE_OUTER_BOUND('',#3335,.T.);
#2288=FACE_OUTER_BOUND('',#3336,.T.);
#2289=FACE_OUTER_BOUND('',#3337,.T.);
#2290=FACE_OUTER_BOUND('',#3338,.T.);
#2291=FACE_OUTER_BOUND('',#3339,.T.);
#2292=FACE_OUTER_BOUND('',#3340,.T.);
#2293=FACE_OUTER_BOUND('',#3341,.T.);
#2294=FACE_OUTER_BOUND('',#3342,.T.);
#2295=FACE_OUTER_BOUND('',#3343,.T.);
#2296=FACE_OUTER_BOUND('',#3344,.T.);
#2297=FACE_OUTER_BOUND('',#3345,.T.);
#2298=FACE_OUTER_BOUND('',#3346,.T.);
#2299=FACE_OUTER_BOUND('',#3347,.T.);
#2300=FACE_OUTER_BOUND('',#3348,.T.);
#2301=FACE_OUTER_BOUND('',#3349,.T.);
#2302=FACE_OUTER_BOUND('',#3350,.T.);
#2303=FACE_OUTER_BOUND('',#3351,.T.);
#2304=FACE_OUTER_BOUND('',#3352,.T.);
#2305=FACE_OUTER_BOUND('',#3353,.T.);
#2306=FACE_OUTER_BOUND('',#3354,.T.);
#2307=FACE_OUTER_BOUND('',#3355,.T.);
#2308=FACE_OUTER_BOUND('',#3356,.T.);
#2309=FACE_OUTER_BOUND('',#3357,.T.);
#2310=FACE_OUTER_BOUND('',#3358,.T.);
#2311=FACE_OUTER_BOUND('',#3359,.T.);
#2312=FACE_OUTER_BOUND('',#3360,.T.);
#2313=FACE_OUTER_BOUND('',#3361,.T.);
#2314=FACE_OUTER_BOUND('',#3362,.T.);
#2315=FACE_OUTER_BOUND('',#3363,.T.);
#2316=FACE_OUTER_BOUND('',#3364,.T.);
#2317=FACE_OUTER_BOUND('',#3365,.T.);
#2318=FACE_OUTER_BOUND('',#3366,.T.);
#2319=FACE_OUTER_BOUND('',#3367,.T.);
#2320=FACE_OUTER_BOUND('',#3368,.T.);
#2321=FACE_OUTER_BOUND('',#3369,.T.);
#2322=FACE_OUTER_BOUND('',#3370,.T.);
#2323=FACE_OUTER_BOUND('',#3371,.T.);
#2324=FACE_OUTER_BOUND('',#3372,.T.);
#2325=FACE_OUTER_BOUND('',#3373,.T.);
#2326=FACE_OUTER_BOUND('',#3374,.T.);
#2327=FACE_OUTER_BOUND('',#3375,.T.);
#2328=FACE_OUTER_BOUND('',#3376,.T.);
#2329=FACE_OUTER_BOUND('',#3377,.T.);
#2330=FACE_OUTER_BOUND('',#3378,.T.);
#2331=FACE_OUTER_BOUND('',#3379,.T.);
#2332=FACE_OUTER_BOUND('',#3380,.T.);
#2333=FACE_OUTER_BOUND('',#3381,.T.);
#2334=FACE_OUTER_BOUND('',#3382,.T.);
#2335=FACE_OUTER_BOUND('',#3383,.T.);
#2336=FACE_OUTER_BOUND('',#3384,.T.);
#2337=FACE_OUTER_BOUND('',#3385,.T.);
#2338=FACE_OUTER_BOUND('',#3386,.T.);
#2339=FACE_OUTER_BOUND('',#3387,.T.);
#2340=FACE_OUTER_BOUND('',#3388,.T.);
#2341=FACE_OUTER_BOUND('',#3389,.T.);
#2342=FACE_OUTER_BOUND('',#3390,.T.);
#2343=FACE_OUTER_BOUND('',#3391,.T.);
#2344=FACE_OUTER_BOUND('',#3392,.T.);
#2345=FACE_OUTER_BOUND('',#3393,.T.);
#2346=FACE_OUTER_BOUND('',#3394,.T.);
#2347=FACE_OUTER_BOUND('',#3395,.T.);
#2348=FACE_OUTER_BOUND('',#3396,.T.);
#2349=FACE_OUTER_BOUND('',#3397,.T.);
#2350=FACE_OUTER_BOUND('',#3398,.T.);
#2351=FACE_OUTER_BOUND('',#3399,.T.);
#2352=FACE_OUTER_BOUND('',#3400,.T.);
#2353=FACE_OUTER_BOUND('',#3401,.T.);
#2354=FACE_OUTER_BOUND('',#3402,.T.);
#2355=FACE_OUTER_BOUND('',#3403,.T.);
#2356=FACE_OUTER_BOUND('',#3404,.T.);
#2357=FACE_OUTER_BOUND('',#3405,.T.);
#2358=FACE_OUTER_BOUND('',#3406,.T.);
#2359=FACE_OUTER_BOUND('',#3407,.T.);
#2360=FACE_OUTER_BOUND('',#3408,.T.);
#2361=FACE_OUTER_BOUND('',#3409,.T.);
#2362=FACE_OUTER_BOUND('',#3410,.T.);
#2363=FACE_OUTER_BOUND('',#3411,.T.);
#2364=FACE_OUTER_BOUND('',#3412,.T.);
#2365=FACE_OUTER_BOUND('',#3414,.T.);
#2366=FACE_OUTER_BOUND('',#3415,.T.);
#2367=FACE_OUTER_BOUND('',#3416,.T.);
#2368=FACE_OUTER_BOUND('',#3417,.T.);
#2369=FACE_OUTER_BOUND('',#3418,.T.);
#2370=FACE_OUTER_BOUND('',#3419,.T.);
#2371=FACE_OUTER_BOUND('',#3420,.T.);
#2372=FACE_OUTER_BOUND('',#3421,.T.);
#2373=FACE_OUTER_BOUND('',#3422,.T.);
#2374=FACE_OUTER_BOUND('',#3423,.T.);
#2375=FACE_OUTER_BOUND('',#3424,.T.);
#2376=FACE_OUTER_BOUND('',#3425,.T.);
#2377=FACE_OUTER_BOUND('',#3426,.T.);
#2378=FACE_OUTER_BOUND('',#3427,.T.);
#2379=FACE_OUTER_BOUND('',#3428,.T.);
#2380=FACE_OUTER_BOUND('',#3429,.T.);
#2381=FACE_OUTER_BOUND('',#3430,.T.);
#2382=FACE_OUTER_BOUND('',#3431,.T.);
#2383=FACE_OUTER_BOUND('',#3432,.T.);
#2384=FACE_OUTER_BOUND('',#3433,.T.);
#2385=FACE_OUTER_BOUND('',#3434,.T.);
#2386=FACE_OUTER_BOUND('',#3435,.T.);
#2387=FACE_OUTER_BOUND('',#3436,.T.);
#2388=FACE_OUTER_BOUND('',#3437,.T.);
#2389=FACE_OUTER_BOUND('',#3438,.T.);
#2390=FACE_OUTER_BOUND('',#3439,.T.);
#2391=FACE_OUTER_BOUND('',#3440,.T.);
#2392=FACE_OUTER_BOUND('',#3441,.T.);
#2393=FACE_OUTER_BOUND('',#3442,.T.);
#2394=FACE_OUTER_BOUND('',#3443,.T.);
#2395=FACE_OUTER_BOUND('',#3444,.T.);
#2396=FACE_OUTER_BOUND('',#3445,.T.);
#2397=FACE_OUTER_BOUND('',#3446,.T.);
#2398=FACE_OUTER_BOUND('',#3447,.T.);
#2399=FACE_OUTER_BOUND('',#3448,.T.);
#2400=FACE_OUTER_BOUND('',#3449,.T.);
#2401=FACE_OUTER_BOUND('',#3450,.T.);
#2402=FACE_OUTER_BOUND('',#3451,.T.);
#2403=FACE_OUTER_BOUND('',#3452,.T.);
#2404=FACE_OUTER_BOUND('',#3453,.T.);
#2405=FACE_OUTER_BOUND('',#3454,.T.);
#2406=FACE_OUTER_BOUND('',#3455,.T.);
#2407=FACE_OUTER_BOUND('',#3456,.T.);
#2408=FACE_OUTER_BOUND('',#3457,.T.);
#2409=FACE_OUTER_BOUND('',#3458,.T.);
#2410=FACE_OUTER_BOUND('',#3459,.T.);
#2411=FACE_OUTER_BOUND('',#3460,.T.);
#2412=FACE_OUTER_BOUND('',#3461,.T.);
#2413=FACE_OUTER_BOUND('',#3462,.T.);
#2414=FACE_OUTER_BOUND('',#3463,.T.);
#2415=FACE_OUTER_BOUND('',#3464,.T.);
#2416=FACE_OUTER_BOUND('',#3465,.T.);
#2417=FACE_OUTER_BOUND('',#3466,.T.);
#2418=FACE_OUTER_BOUND('',#3467,.T.);
#2419=FACE_OUTER_BOUND('',#3468,.T.);
#2420=FACE_OUTER_BOUND('',#3469,.T.);
#2421=FACE_OUTER_BOUND('',#3470,.T.);
#2422=FACE_OUTER_BOUND('',#3471,.T.);
#2423=FACE_OUTER_BOUND('',#3472,.T.);
#2424=FACE_OUTER_BOUND('',#3473,.T.);
#2425=FACE_OUTER_BOUND('',#3474,.T.);
#2426=FACE_OUTER_BOUND('',#3475,.T.);
#2427=FACE_OUTER_BOUND('',#3476,.T.);
#2428=FACE_OUTER_BOUND('',#3477,.T.);
#2429=FACE_OUTER_BOUND('',#3478,.T.);
#2430=FACE_OUTER_BOUND('',#3479,.T.);
#2431=FACE_OUTER_BOUND('',#3480,.T.);
#2432=FACE_OUTER_BOUND('',#3481,.T.);
#2433=FACE_OUTER_BOUND('',#3482,.T.);
#2434=FACE_OUTER_BOUND('',#3483,.T.);
#2435=FACE_OUTER_BOUND('',#3484,.T.);
#2436=FACE_OUTER_BOUND('',#3485,.T.);
#2437=FACE_OUTER_BOUND('',#3486,.T.);
#2438=FACE_OUTER_BOUND('',#3487,.T.);
#2439=FACE_OUTER_BOUND('',#3488,.T.);
#2440=FACE_OUTER_BOUND('',#3489,.T.);
#2441=FACE_OUTER_BOUND('',#3490,.T.);
#2442=FACE_OUTER_BOUND('',#3491,.T.);
#2443=FACE_OUTER_BOUND('',#3492,.T.);
#2444=FACE_OUTER_BOUND('',#3493,.T.);
#2445=FACE_OUTER_BOUND('',#3494,.T.);
#2446=FACE_OUTER_BOUND('',#3495,.T.);
#2447=FACE_OUTER_BOUND('',#3496,.T.);
#2448=FACE_OUTER_BOUND('',#3497,.T.);
#2449=FACE_OUTER_BOUND('',#3498,.T.);
#2450=FACE_OUTER_BOUND('',#3499,.T.);
#2451=FACE_OUTER_BOUND('',#3500,.T.);
#2452=FACE_OUTER_BOUND('',#3501,.T.);
#2453=FACE_OUTER_BOUND('',#3502,.T.);
#2454=FACE_OUTER_BOUND('',#3503,.T.);
#2455=FACE_OUTER_BOUND('',#3504,.T.);
#2456=FACE_OUTER_BOUND('',#3505,.T.);
#2457=FACE_OUTER_BOUND('',#3506,.T.);
#2458=FACE_OUTER_BOUND('',#3507,.T.);
#2459=FACE_OUTER_BOUND('',#3508,.T.);
#2460=FACE_OUTER_BOUND('',#3509,.T.);
#2461=FACE_OUTER_BOUND('',#3510,.T.);
#2462=FACE_OUTER_BOUND('',#3511,.T.);
#2463=FACE_OUTER_BOUND('',#3512,.T.);
#2464=FACE_OUTER_BOUND('',#3513,.T.);
#2465=FACE_OUTER_BOUND('',#3514,.T.);
#2466=FACE_OUTER_BOUND('',#3515,.T.);
#2467=FACE_OUTER_BOUND('',#3516,.T.);
#2468=FACE_OUTER_BOUND('',#3517,.T.);
#2469=FACE_OUTER_BOUND('',#3518,.T.);
#2470=FACE_OUTER_BOUND('',#3519,.T.);
#2471=FACE_OUTER_BOUND('',#3520,.T.);
#2472=FACE_OUTER_BOUND('',#3521,.T.);
#2473=FACE_OUTER_BOUND('',#3522,.T.);
#2474=FACE_OUTER_BOUND('',#3523,.T.);
#2475=FACE_OUTER_BOUND('',#3524,.T.);
#2476=FACE_OUTER_BOUND('',#3525,.T.);
#2477=FACE_OUTER_BOUND('',#3526,.T.);
#2478=FACE_OUTER_BOUND('',#3527,.T.);
#2479=FACE_OUTER_BOUND('',#3528,.T.);
#2480=FACE_OUTER_BOUND('',#3529,.T.);
#2481=FACE_OUTER_BOUND('',#3530,.T.);
#2482=FACE_OUTER_BOUND('',#3531,.T.);
#2483=FACE_OUTER_BOUND('',#3532,.T.);
#2484=FACE_OUTER_BOUND('',#3533,.T.);
#2485=FACE_OUTER_BOUND('',#3534,.T.);
#2486=FACE_OUTER_BOUND('',#3535,.T.);
#2487=FACE_OUTER_BOUND('',#3536,.T.);
#2488=FACE_OUTER_BOUND('',#3537,.T.);
#2489=FACE_OUTER_BOUND('',#3538,.T.);
#2490=FACE_OUTER_BOUND('',#3539,.T.);
#2491=FACE_OUTER_BOUND('',#3541,.T.);
#2492=FACE_OUTER_BOUND('',#3543,.T.);
#2493=FACE_OUTER_BOUND('',#3544,.T.);
#2494=FACE_OUTER_BOUND('',#3545,.T.);
#2495=FACE_OUTER_BOUND('',#3546,.T.);
#2496=FACE_OUTER_BOUND('',#3547,.T.);
#2497=FACE_OUTER_BOUND('',#3548,.T.);
#2498=FACE_OUTER_BOUND('',#3549,.T.);
#2499=FACE_OUTER_BOUND('',#3550,.T.);
#2500=FACE_OUTER_BOUND('',#3551,.T.);
#2501=FACE_OUTER_BOUND('',#3552,.T.);
#2502=FACE_OUTER_BOUND('',#3553,.T.);
#2503=FACE_OUTER_BOUND('',#3554,.T.);
#2504=FACE_OUTER_BOUND('',#3555,.T.);
#2505=FACE_OUTER_BOUND('',#3556,.T.);
#2506=FACE_OUTER_BOUND('',#3557,.T.);
#2507=FACE_OUTER_BOUND('',#3558,.T.);
#2508=FACE_OUTER_BOUND('',#3559,.T.);
#2509=FACE_OUTER_BOUND('',#3560,.T.);
#2510=FACE_OUTER_BOUND('',#3561,.T.);
#2511=FACE_OUTER_BOUND('',#3562,.T.);
#2512=FACE_OUTER_BOUND('',#3563,.T.);
#2513=FACE_OUTER_BOUND('',#3564,.T.);
#2514=FACE_OUTER_BOUND('',#3565,.T.);
#2515=FACE_OUTER_BOUND('',#3566,.T.);
#2516=FACE_OUTER_BOUND('',#3567,.T.);
#2517=FACE_OUTER_BOUND('',#3568,.T.);
#2518=FACE_OUTER_BOUND('',#3569,.T.);
#2519=FACE_OUTER_BOUND('',#3570,.T.);
#2520=FACE_OUTER_BOUND('',#3571,.T.);
#2521=FACE_OUTER_BOUND('',#3572,.T.);
#2522=FACE_OUTER_BOUND('',#3573,.T.);
#2523=FACE_OUTER_BOUND('',#3574,.T.);
#2524=FACE_OUTER_BOUND('',#3575,.T.);
#2525=FACE_OUTER_BOUND('',#3576,.T.);
#2526=FACE_OUTER_BOUND('',#3577,.T.);
#2527=FACE_OUTER_BOUND('',#3578,.T.);
#2528=FACE_OUTER_BOUND('',#3579,.T.);
#2529=FACE_OUTER_BOUND('',#3580,.T.);
#2530=FACE_OUTER_BOUND('',#3581,.T.);
#2531=FACE_OUTER_BOUND('',#3582,.T.);
#2532=FACE_OUTER_BOUND('',#3583,.T.);
#2533=FACE_OUTER_BOUND('',#3584,.T.);
#2534=FACE_OUTER_BOUND('',#3585,.T.);
#2535=FACE_OUTER_BOUND('',#3586,.T.);
#2536=FACE_OUTER_BOUND('',#3587,.T.);
#2537=FACE_OUTER_BOUND('',#3588,.T.);
#2538=FACE_OUTER_BOUND('',#3589,.T.);
#2539=FACE_OUTER_BOUND('',#3590,.T.);
#2540=FACE_OUTER_BOUND('',#3591,.T.);
#2541=FACE_OUTER_BOUND('',#3592,.T.);
#2542=FACE_OUTER_BOUND('',#3593,.T.);
#2543=FACE_OUTER_BOUND('',#3594,.T.);
#2544=FACE_OUTER_BOUND('',#3595,.T.);
#2545=FACE_OUTER_BOUND('',#3596,.T.);
#2546=FACE_OUTER_BOUND('',#3597,.T.);
#2547=FACE_OUTER_BOUND('',#3598,.T.);
#2548=FACE_OUTER_BOUND('',#3599,.T.);
#2549=FACE_OUTER_BOUND('',#3600,.T.);
#2550=FACE_OUTER_BOUND('',#3601,.T.);
#2551=FACE_OUTER_BOUND('',#3602,.T.);
#2552=FACE_OUTER_BOUND('',#3603,.T.);
#2553=FACE_OUTER_BOUND('',#3604,.T.);
#2554=FACE_OUTER_BOUND('',#3605,.T.);
#2555=FACE_OUTER_BOUND('',#3606,.T.);
#2556=FACE_OUTER_BOUND('',#3607,.T.);
#2557=FACE_OUTER_BOUND('',#3608,.T.);
#2558=FACE_OUTER_BOUND('',#3609,.T.);
#2559=FACE_OUTER_BOUND('',#3610,.T.);
#2560=FACE_OUTER_BOUND('',#3611,.T.);
#2561=FACE_OUTER_BOUND('',#3612,.T.);
#2562=FACE_OUTER_BOUND('',#3613,.T.);
#2563=FACE_OUTER_BOUND('',#3614,.T.);
#2564=FACE_OUTER_BOUND('',#3615,.T.);
#2565=FACE_OUTER_BOUND('',#3616,.T.);
#2566=FACE_OUTER_BOUND('',#3617,.T.);
#2567=FACE_OUTER_BOUND('',#3618,.T.);
#2568=FACE_OUTER_BOUND('',#3619,.T.);
#2569=FACE_OUTER_BOUND('',#3620,.T.);
#2570=FACE_OUTER_BOUND('',#3621,.T.);
#2571=FACE_OUTER_BOUND('',#3622,.T.);
#2572=FACE_OUTER_BOUND('',#3623,.T.);
#2573=FACE_OUTER_BOUND('',#3624,.T.);
#2574=FACE_OUTER_BOUND('',#3625,.T.);
#2575=FACE_OUTER_BOUND('',#3626,.T.);
#2576=FACE_OUTER_BOUND('',#3627,.T.);
#2577=FACE_OUTER_BOUND('',#3628,.T.);
#2578=FACE_OUTER_BOUND('',#3629,.T.);
#2579=FACE_OUTER_BOUND('',#3630,.T.);
#2580=FACE_OUTER_BOUND('',#3631,.T.);
#2581=FACE_OUTER_BOUND('',#3632,.T.);
#2582=FACE_OUTER_BOUND('',#3633,.T.);
#2583=FACE_OUTER_BOUND('',#3634,.T.);
#2584=FACE_OUTER_BOUND('',#3635,.T.);
#2585=FACE_OUTER_BOUND('',#3636,.T.);
#2586=FACE_OUTER_BOUND('',#3637,.T.);
#2587=FACE_OUTER_BOUND('',#3638,.T.);
#2588=FACE_OUTER_BOUND('',#3639,.T.);
#2589=FACE_OUTER_BOUND('',#3640,.T.);
#2590=FACE_OUTER_BOUND('',#3641,.T.);
#2591=FACE_OUTER_BOUND('',#3642,.T.);
#2592=FACE_OUTER_BOUND('',#3643,.T.);
#2593=FACE_OUTER_BOUND('',#3644,.T.);
#2594=FACE_OUTER_BOUND('',#3645,.T.);
#2595=FACE_OUTER_BOUND('',#3646,.T.);
#2596=FACE_OUTER_BOUND('',#3647,.T.);
#2597=FACE_OUTER_BOUND('',#3648,.T.);
#2598=FACE_OUTER_BOUND('',#3649,.T.);
#2599=FACE_OUTER_BOUND('',#3650,.T.);
#2600=FACE_OUTER_BOUND('',#3651,.T.);
#2601=FACE_OUTER_BOUND('',#3652,.T.);
#2602=FACE_OUTER_BOUND('',#3653,.T.);
#2603=FACE_OUTER_BOUND('',#3654,.T.);
#2604=FACE_OUTER_BOUND('',#3655,.T.);
#2605=FACE_OUTER_BOUND('',#3656,.T.);
#2606=FACE_OUTER_BOUND('',#3657,.T.);
#2607=FACE_OUTER_BOUND('',#3658,.T.);
#2608=FACE_OUTER_BOUND('',#3659,.T.);
#2609=FACE_OUTER_BOUND('',#3660,.T.);
#2610=FACE_OUTER_BOUND('',#3661,.T.);
#2611=FACE_OUTER_BOUND('',#3662,.T.);
#2612=FACE_OUTER_BOUND('',#3663,.T.);
#2613=FACE_OUTER_BOUND('',#3664,.T.);
#2614=FACE_OUTER_BOUND('',#3665,.T.);
#2615=FACE_OUTER_BOUND('',#3666,.T.);
#2616=FACE_OUTER_BOUND('',#3667,.T.);
#2617=FACE_OUTER_BOUND('',#3668,.T.);
#2618=FACE_OUTER_BOUND('',#3669,.T.);
#2619=FACE_OUTER_BOUND('',#3670,.T.);
#2620=FACE_OUTER_BOUND('',#3671,.T.);
#2621=FACE_OUTER_BOUND('',#3672,.T.);
#2622=FACE_OUTER_BOUND('',#3673,.T.);
#2623=FACE_OUTER_BOUND('',#3674,.T.);
#2624=FACE_OUTER_BOUND('',#3675,.T.);
#2625=FACE_OUTER_BOUND('',#3676,.T.);
#2626=FACE_OUTER_BOUND('',#3677,.T.);
#2627=FACE_OUTER_BOUND('',#3678,.T.);
#2628=FACE_OUTER_BOUND('',#3679,.T.);
#2629=FACE_OUTER_BOUND('',#3680,.T.);
#2630=FACE_OUTER_BOUND('',#3681,.T.);
#2631=FACE_OUTER_BOUND('',#3682,.T.);
#2632=FACE_OUTER_BOUND('',#3683,.T.);
#2633=FACE_OUTER_BOUND('',#3684,.T.);
#2634=FACE_OUTER_BOUND('',#3685,.T.);
#2635=FACE_OUTER_BOUND('',#3686,.T.);
#2636=FACE_OUTER_BOUND('',#3687,.T.);
#2637=FACE_OUTER_BOUND('',#3688,.T.);
#2638=FACE_OUTER_BOUND('',#3689,.T.);
#2639=FACE_OUTER_BOUND('',#3690,.T.);
#2640=FACE_OUTER_BOUND('',#3691,.T.);
#2641=FACE_OUTER_BOUND('',#3692,.T.);
#2642=FACE_OUTER_BOUND('',#3693,.T.);
#2643=FACE_OUTER_BOUND('',#3694,.T.);
#2644=FACE_OUTER_BOUND('',#3695,.T.);
#2645=FACE_OUTER_BOUND('',#3696,.T.);
#2646=FACE_OUTER_BOUND('',#3697,.T.);
#2998=EDGE_LOOP('',(#12369,#12370,#12371,#12372));
#2999=EDGE_LOOP('',(#12373,#12374,#12375,#12376,#12377));
#3000=EDGE_LOOP('',(#12378,#12379,#12380,#12381,#12382));
#3001=EDGE_LOOP('',(#12383,#12384,#12385,#12386));
#3002=EDGE_LOOP('',(#12387,#12388,#12389,#12390));
#3003=EDGE_LOOP('',(#12391,#12392,#12393,#12394,#12395));
#3004=EDGE_LOOP('',(#12396,#12397,#12398,#12399,#12400));
#3005=EDGE_LOOP('',(#12401,#12402,#12403,#12404));
#3006=EDGE_LOOP('',(#12405,#12406,#12407,#12408));
#3007=EDGE_LOOP('',(#12409,#12410,#12411,#12412));
#3008=EDGE_LOOP('',(#12413,#12414,#12415,#12416,#12417,#12418,#12419));
#3009=EDGE_LOOP('',(#12420,#12421,#12422,#12423));
#3010=EDGE_LOOP('',(#12424,#12425,#12426,#12427,#12428));
#3011=EDGE_LOOP('',(#12429,#12430,#12431,#12432,#12433,#12434));
#3012=EDGE_LOOP('',(#12435,#12436,#12437,#12438,#12439));
#3013=EDGE_LOOP('',(#12440,#12441,#12442,#12443,#12444));
#3014=EDGE_LOOP('',(#12445,#12446,#12447,#12448));
#3015=EDGE_LOOP('',(#12449,#12450,#12451,#12452));
#3016=EDGE_LOOP('',(#12453,#12454,#12455,#12456,#12457,#12458,#12459,#12460,
#12461,#12462,#12463,#12464,#12465,#12466,#12467,#12468));
#3017=EDGE_LOOP('',(#12469));
#3018=EDGE_LOOP('',(#12470));
#3019=EDGE_LOOP('',(#12471,#12472,#12473,#12474));
#3020=EDGE_LOOP('',(#12475,#12476,#12477,#12478,#12479,#12480,#12481,#12482,
#12483,#12484,#12485,#12486,#12487,#12488,#12489,#12490,#12491,#12492,#12493,
#12494));
#3021=EDGE_LOOP('',(#12495,#12496,#12497,#12498));
#3022=EDGE_LOOP('',(#12499,#12500,#12501,#12502,#12503,#12504,#12505,#12506));
#3023=EDGE_LOOP('',(#12507));
#3024=EDGE_LOOP('',(#12508));
#3025=EDGE_LOOP('',(#12509,#12510,#12511,#12512,#12513,#12514,#12515));
#3026=EDGE_LOOP('',(#12516));
#3027=EDGE_LOOP('',(#12517,#12518,#12519,#12520,#12521,#12522,#12523,#12524,
#12525));
#3028=EDGE_LOOP('',(#12526));
#3029=EDGE_LOOP('',(#12527,#12528,#12529,#12530));
#3030=EDGE_LOOP('',(#12531,#12532,#12533,#12534,#12535,#12536,#12537,#12538,
#12539,#12540,#12541));
#3031=EDGE_LOOP('',(#12542,#12543,#12544,#12545,#12546,#12547,#12548,#12549));
#3032=EDGE_LOOP('',(#12550));
#3033=EDGE_LOOP('',(#12551,#12552,#12553,#12554));
#3034=EDGE_LOOP('',(#12555,#12556,#12557,#12558,#12559,#12560));
#3035=EDGE_LOOP('',(#12561,#12562,#12563,#12564));
#3036=EDGE_LOOP('',(#12565,#12566,#12567,#12568));
#3037=EDGE_LOOP('',(#12569,#12570,#12571,#12572));
#3038=EDGE_LOOP('',(#12573,#12574,#12575,#12576));
#3039=EDGE_LOOP('',(#12577,#12578,#12579,#12580,#12581,#12582));
#3040=EDGE_LOOP('',(#12583,#12584,#12585,#12586,#12587,#12588,#12589));
#3041=EDGE_LOOP('',(#12590));
#3042=EDGE_LOOP('',(#12591,#12592,#12593,#12594));
#3043=EDGE_LOOP('',(#12595,#12596,#12597,#12598));
#3044=EDGE_LOOP('',(#12599,#12600,#12601,#12602));
#3045=EDGE_LOOP('',(#12603,#12604,#12605,#12606));
#3046=EDGE_LOOP('',(#12607,#12608,#12609,#12610,#12611));
#3047=EDGE_LOOP('',(#12612));
#3048=EDGE_LOOP('',(#12613,#12614,#12615,#12616));
#3049=EDGE_LOOP('',(#12617,#12618,#12619,#12620));
#3050=EDGE_LOOP('',(#12621,#12622,#12623,#12624));
#3051=EDGE_LOOP('',(#12625,#12626,#12627,#12628));
#3052=EDGE_LOOP('',(#12629,#12630,#12631,#12632));
#3053=EDGE_LOOP('',(#12633,#12634,#12635,#12636));
#3054=EDGE_LOOP('',(#12637,#12638,#12639,#12640));
#3055=EDGE_LOOP('',(#12641,#12642,#12643,#12644));
#3056=EDGE_LOOP('',(#12645,#12646,#12647));
#3057=EDGE_LOOP('',(#12648,#12649,#12650,#12651));
#3058=EDGE_LOOP('',(#12652,#12653,#12654,#12655));
#3059=EDGE_LOOP('',(#12656,#12657,#12658,#12659));
#3060=EDGE_LOOP('',(#12660,#12661,#12662,#12663));
#3061=EDGE_LOOP('',(#12664,#12665,#12666,#12667));
#3062=EDGE_LOOP('',(#12668,#12669,#12670,#12671));
#3063=EDGE_LOOP('',(#12672,#12673,#12674,#12675));
#3064=EDGE_LOOP('',(#12676,#12677,#12678));
#3065=EDGE_LOOP('',(#12679,#12680,#12681));
#3066=EDGE_LOOP('',(#12682,#12683,#12684,#12685));
#3067=EDGE_LOOP('',(#12686,#12687,#12688,#12689));
#3068=EDGE_LOOP('',(#12690,#12691,#12692,#12693));
#3069=EDGE_LOOP('',(#12694,#12695,#12696,#12697));
#3070=EDGE_LOOP('',(#12698,#12699,#12700));
#3071=EDGE_LOOP('',(#12701,#12702,#12703,#12704));
#3072=EDGE_LOOP('',(#12705,#12706,#12707));
#3073=EDGE_LOOP('',(#12708,#12709,#12710,#12711));
#3074=EDGE_LOOP('',(#12712,#12713,#12714,#12715));
#3075=EDGE_LOOP('',(#12716,#12717,#12718,#12719));
#3076=EDGE_LOOP('',(#12720,#12721,#12722,#12723));
#3077=EDGE_LOOP('',(#12724,#12725,#12726,#12727));
#3078=EDGE_LOOP('',(#12728,#12729,#12730));
#3079=EDGE_LOOP('',(#12731,#12732,#12733,#12734));
#3080=EDGE_LOOP('',(#12735,#12736,#12737,#12738));
#3081=EDGE_LOOP('',(#12739,#12740,#12741,#12742));
#3082=EDGE_LOOP('',(#12743,#12744,#12745,#12746));
#3083=EDGE_LOOP('',(#12747,#12748,#12749,#12750,#12751));
#3084=EDGE_LOOP('',(#12752,#12753,#12754,#12755,#12756));
#3085=EDGE_LOOP('',(#12757,#12758,#12759,#12760,#12761,#12762));
#3086=EDGE_LOOP('',(#12763));
#3087=EDGE_LOOP('',(#12764));
#3088=EDGE_LOOP('',(#12765,#12766,#12767,#12768));
#3089=EDGE_LOOP('',(#12769,#12770,#12771,#12772,#12773,#12774));
#3090=EDGE_LOOP('',(#12775,#12776,#12777,#12778));
#3091=EDGE_LOOP('',(#12779,#12780,#12781,#12782));
#3092=EDGE_LOOP('',(#12783,#12784,#12785,#12786));
#3093=EDGE_LOOP('',(#12787,#12788,#12789,#12790));
#3094=EDGE_LOOP('',(#12791,#12792,#12793,#12794));
#3095=EDGE_LOOP('',(#12795,#12796,#12797,#12798));
#3096=EDGE_LOOP('',(#12799,#12800,#12801,#12802));
#3097=EDGE_LOOP('',(#12803,#12804,#12805,#12806,#12807));
#3098=EDGE_LOOP('',(#12808));
#3099=EDGE_LOOP('',(#12809,#12810,#12811,#12812,#12813));
#3100=EDGE_LOOP('',(#12814));
#3101=EDGE_LOOP('',(#12815,#12816,#12817,#12818,#12819));
#3102=EDGE_LOOP('',(#12820,#12821,#12822,#12823,#12824,#12825,#12826,#12827,
#12828));
#3103=EDGE_LOOP('',(#12829));
#3104=EDGE_LOOP('',(#12830,#12831,#12832,#12833));
#3105=EDGE_LOOP('',(#12834,#12835,#12836,#12837));
#3106=EDGE_LOOP('',(#12838,#12839,#12840,#12841,#12842,#12843,#12844,#12845,
#12846));
#3107=EDGE_LOOP('',(#12847));
#3108=EDGE_LOOP('',(#12848,#12849,#12850,#12851,#12852));
#3109=EDGE_LOOP('',(#12853));
#3110=EDGE_LOOP('',(#12854,#12855,#12856,#12857,#12858));
#3111=EDGE_LOOP('',(#12859));
#3112=EDGE_LOOP('',(#12860,#12861,#12862,#12863));
#3113=EDGE_LOOP('',(#12864));
#3114=EDGE_LOOP('',(#12865));
#3115=EDGE_LOOP('',(#12866));
#3116=EDGE_LOOP('',(#12867));
#3117=EDGE_LOOP('',(#12868));
#3118=EDGE_LOOP('',(#12869,#12870,#12871,#12872));
#3119=EDGE_LOOP('',(#12873,#12874));
#3120=EDGE_LOOP('',(#12875));
#3121=EDGE_LOOP('',(#12876));
#3122=EDGE_LOOP('',(#12877,#12878,#12879,#12880));
#3123=EDGE_LOOP('',(#12881,#12882,#12883,#12884,#12885));
#3124=EDGE_LOOP('',(#12886,#12887,#12888,#12889,#12890,#12891));
#3125=EDGE_LOOP('',(#12892,#12893,#12894,#12895,#12896,#12897));
#3126=EDGE_LOOP('',(#12898,#12899,#12900,#12901,#12902,#12903));
#3127=EDGE_LOOP('',(#12904,#12905,#12906,#12907,#12908,#12909));
#3128=EDGE_LOOP('',(#12910,#12911,#12912,#12913,#12914,#12915));
#3129=EDGE_LOOP('',(#12916,#12917,#12918,#12919,#12920,#12921));
#3130=EDGE_LOOP('',(#12922,#12923,#12924,#12925,#12926,#12927));
#3131=EDGE_LOOP('',(#12928,#12929,#12930,#12931,#12932,#12933));
#3132=EDGE_LOOP('',(#12934,#12935,#12936,#12937,#12938,#12939));
#3133=EDGE_LOOP('',(#12940,#12941,#12942,#12943,#12944,#12945));
#3134=EDGE_LOOP('',(#12946,#12947,#12948,#12949,#12950,#12951));
#3135=EDGE_LOOP('',(#12952,#12953,#12954,#12955,#12956,#12957));
#3136=EDGE_LOOP('',(#12958,#12959,#12960,#12961,#12962,#12963));
#3137=EDGE_LOOP('',(#12964,#12965,#12966,#12967,#12968,#12969));
#3138=EDGE_LOOP('',(#12970,#12971,#12972,#12973,#12974,#12975));
#3139=EDGE_LOOP('',(#12976,#12977,#12978,#12979,#12980,#12981));
#3140=EDGE_LOOP('',(#12982,#12983,#12984,#12985,#12986,#12987));
#3141=EDGE_LOOP('',(#12988,#12989,#12990,#12991,#12992,#12993));
#3142=EDGE_LOOP('',(#12994,#12995,#12996,#12997,#12998,#12999));
#3143=EDGE_LOOP('',(#13000,#13001,#13002,#13003,#13004,#13005));
#3144=EDGE_LOOP('',(#13006,#13007,#13008,#13009,#13010,#13011));
#3145=EDGE_LOOP('',(#13012,#13013,#13014,#13015,#13016,#13017));
#3146=EDGE_LOOP('',(#13018,#13019,#13020,#13021,#13022,#13023));
#3147=EDGE_LOOP('',(#13024,#13025,#13026,#13027,#13028,#13029));
#3148=EDGE_LOOP('',(#13030,#13031,#13032,#13033,#13034,#13035));
#3149=EDGE_LOOP('',(#13036,#13037,#13038,#13039,#13040,#13041));
#3150=EDGE_LOOP('',(#13042,#13043,#13044,#13045,#13046,#13047));
#3151=EDGE_LOOP('',(#13048,#13049,#13050,#13051,#13052,#13053));
#3152=EDGE_LOOP('',(#13054,#13055,#13056,#13057,#13058,#13059));
#3153=EDGE_LOOP('',(#13060,#13061,#13062,#13063,#13064,#13065));
#3154=EDGE_LOOP('',(#13066,#13067,#13068,#13069,#13070,#13071));
#3155=EDGE_LOOP('',(#13072,#13073,#13074,#13075,#13076,#13077));
#3156=EDGE_LOOP('',(#13078,#13079,#13080,#13081,#13082,#13083));
#3157=EDGE_LOOP('',(#13084,#13085,#13086,#13087,#13088,#13089));
#3158=EDGE_LOOP('',(#13090,#13091,#13092,#13093,#13094,#13095));
#3159=EDGE_LOOP('',(#13096,#13097,#13098,#13099,#13100,#13101));
#3160=EDGE_LOOP('',(#13102,#13103,#13104,#13105,#13106,#13107));
#3161=EDGE_LOOP('',(#13108,#13109,#13110,#13111,#13112,#13113));
#3162=EDGE_LOOP('',(#13114,#13115,#13116,#13117,#13118,#13119));
#3163=EDGE_LOOP('',(#13120,#13121,#13122,#13123,#13124,#13125));
#3164=EDGE_LOOP('',(#13126,#13127,#13128,#13129,#13130,#13131));
#3165=EDGE_LOOP('',(#13132,#13133,#13134,#13135,#13136,#13137));
#3166=EDGE_LOOP('',(#13138,#13139,#13140,#13141,#13142,#13143));
#3167=EDGE_LOOP('',(#13144,#13145,#13146,#13147,#13148,#13149));
#3168=EDGE_LOOP('',(#13150,#13151,#13152,#13153,#13154,#13155,#13156,#13157,
#13158,#13159,#13160,#13161,#13162,#13163,#13164,#13165,#13166,#13167,#13168,
#13169,#13170,#13171,#13172,#13173,#13174,#13175,#13176,#13177,#13178,#13179,
#13180,#13181,#13182,#13183,#13184,#13185,#13186,#13187,#13188,#13189,#13190,
#13191,#13192,#13193,#13194,#13195,#13196,#13197,#13198,#13199,#13200,#13201,
#13202,#13203,#13204,#13205,#13206,#13207,#13208,#13209,#13210,#13211,#13212,
#13213,#13214,#13215,#13216,#13217,#13218,#13219,#13220,#13221,#13222,#13223,
#13224,#13225,#13226,#13227,#13228,#13229,#13230,#13231,#13232,#13233,#13234,
#13235,#13236,#13237,#13238,#13239,#13240,#13241,#13242,#13243,#13244,#13245,
#13246,#13247,#13248,#13249,#13250,#13251,#13252,#13253,#13254,#13255,#13256,
#13257,#13258,#13259,#13260,#13261,#13262,#13263,#13264,#13265,#13266,#13267,
#13268,#13269,#13270,#13271,#13272,#13273,#13274,#13275,#13276,#13277,#13278,
#13279,#13280,#13281,#13282,#13283,#13284,#13285,#13286,#13287,#13288,#13289,
#13290,#13291,#13292,#13293,#13294,#13295,#13296,#13297,#13298,#13299,#13300,
#13301,#13302,#13303,#13304,#13305,#13306,#13307,#13308,#13309,#13310,#13311,
#13312,#13313,#13314,#13315,#13316,#13317,#13318,#13319,#13320,#13321,#13322,
#13323,#13324,#13325,#13326,#13327,#13328,#13329,#13330,#13331,#13332,#13333,
#13334,#13335,#13336,#13337,#13338,#13339,#13340,#13341,#13342,#13343,#13344,
#13345,#13346,#13347,#13348,#13349,#13350,#13351,#13352,#13353,#13354,#13355,
#13356,#13357,#13358,#13359,#13360,#13361,#13362,#13363,#13364,#13365,#13366,
#13367,#13368,#13369,#13370,#13371,#13372,#13373,#13374,#13375,#13376,#13377,
#13378,#13379,#13380,#13381,#13382,#13383,#13384));
#3169=EDGE_LOOP('',(#13385,#13386,#13387,#13388,#13389,#13390,#13391,#13392,
#13393,#13394,#13395,#13396,#13397,#13398,#13399,#13400,#13401,#13402,#13403,
#13404,#13405,#13406,#13407,#13408,#13409,#13410,#13411,#13412,#13413,#13414,
#13415,#13416,#13417,#13418,#13419,#13420,#13421,#13422,#13423,#13424,#13425,
#13426,#13427,#13428,#13429,#13430,#13431,#13432,#13433,#13434,#13435,#13436,
#13437,#13438,#13439,#13440,#13441,#13442,#13443,#13444,#13445,#13446,#13447,
#13448,#13449,#13450,#13451,#13452,#13453,#13454,#13455,#13456,#13457,#13458,
#13459,#13460,#13461,#13462,#13463,#13464,#13465,#13466,#13467,#13468,#13469,
#13470,#13471,#13472,#13473,#13474,#13475,#13476,#13477,#13478,#13479,#13480,
#13481,#13482,#13483,#13484,#13485,#13486,#13487,#13488,#13489,#13490,#13491,
#13492,#13493,#13494,#13495,#13496,#13497,#13498,#13499,#13500,#13501,#13502,
#13503,#13504,#13505,#13506,#13507,#13508,#13509,#13510,#13511,#13512,#13513,
#13514,#13515,#13516,#13517,#13518,#13519,#13520,#13521,#13522,#13523,#13524,
#13525,#13526,#13527,#13528,#13529,#13530,#13531,#13532,#13533,#13534,#13535,
#13536,#13537,#13538,#13539,#13540,#13541,#13542,#13543,#13544,#13545,#13546,
#13547,#13548,#13549,#13550,#13551,#13552,#13553,#13554,#13555,#13556,#13557,
#13558,#13559,#13560,#13561,#13562,#13563,#13564,#13565,#13566,#13567,#13568,
#13569,#13570,#13571,#13572,#13573,#13574,#13575,#13576,#13577,#13578,#13579,
#13580,#13581,#13582,#13583,#13584,#13585,#13586,#13587,#13588,#13589,#13590,
#13591,#13592,#13593,#13594,#13595,#13596,#13597,#13598,#13599,#13600,#13601,
#13602,#13603,#13604,#13605,#13606,#13607,#13608,#13609,#13610,#13611,#13612,
#13613,#13614,#13615,#13616,#13617,#13618,#13619));
#3170=EDGE_LOOP('',(#13620,#13621,#13622,#13623,#13624));
#3171=EDGE_LOOP('',(#13625,#13626,#13627,#13628));
#3172=EDGE_LOOP('',(#13629,#13630,#13631,#13632));
#3173=EDGE_LOOP('',(#13633,#13634,#13635,#13636));
#3174=EDGE_LOOP('',(#13637,#13638,#13639,#13640));
#3175=EDGE_LOOP('',(#13641,#13642,#13643,#13644));
#3176=EDGE_LOOP('',(#13645,#13646,#13647,#13648));
#3177=EDGE_LOOP('',(#13649,#13650,#13651,#13652));
#3178=EDGE_LOOP('',(#13653,#13654,#13655,#13656));
#3179=EDGE_LOOP('',(#13657,#13658,#13659,#13660));
#3180=EDGE_LOOP('',(#13661,#13662,#13663,#13664));
#3181=EDGE_LOOP('',(#13665,#13666,#13667,#13668));
#3182=EDGE_LOOP('',(#13669,#13670,#13671,#13672));
#3183=EDGE_LOOP('',(#13673,#13674,#13675,#13676));
#3184=EDGE_LOOP('',(#13677,#13678,#13679,#13680));
#3185=EDGE_LOOP('',(#13681,#13682,#13683,#13684));
#3186=EDGE_LOOP('',(#13685,#13686,#13687,#13688));
#3187=EDGE_LOOP('',(#13689,#13690,#13691,#13692));
#3188=EDGE_LOOP('',(#13693,#13694,#13695,#13696));
#3189=EDGE_LOOP('',(#13697,#13698,#13699,#13700));
#3190=EDGE_LOOP('',(#13701,#13702,#13703,#13704));
#3191=EDGE_LOOP('',(#13705,#13706,#13707,#13708));
#3192=EDGE_LOOP('',(#13709,#13710,#13711,#13712));
#3193=EDGE_LOOP('',(#13713,#13714,#13715,#13716));
#3194=EDGE_LOOP('',(#13717,#13718,#13719,#13720));
#3195=EDGE_LOOP('',(#13721,#13722,#13723,#13724));
#3196=EDGE_LOOP('',(#13725,#13726,#13727,#13728));
#3197=EDGE_LOOP('',(#13729,#13730,#13731,#13732));
#3198=EDGE_LOOP('',(#13733,#13734,#13735,#13736));
#3199=EDGE_LOOP('',(#13737,#13738,#13739,#13740));
#3200=EDGE_LOOP('',(#13741,#13742,#13743,#13744));
#3201=EDGE_LOOP('',(#13745,#13746,#13747,#13748));
#3202=EDGE_LOOP('',(#13749,#13750,#13751,#13752));
#3203=EDGE_LOOP('',(#13753,#13754,#13755,#13756));
#3204=EDGE_LOOP('',(#13757,#13758,#13759,#13760));
#3205=EDGE_LOOP('',(#13761,#13762,#13763,#13764));
#3206=EDGE_LOOP('',(#13765,#13766,#13767,#13768));
#3207=EDGE_LOOP('',(#13769,#13770,#13771,#13772));
#3208=EDGE_LOOP('',(#13773,#13774,#13775,#13776));
#3209=EDGE_LOOP('',(#13777,#13778,#13779,#13780));
#3210=EDGE_LOOP('',(#13781,#13782,#13783,#13784));
#3211=EDGE_LOOP('',(#13785,#13786,#13787,#13788));
#3212=EDGE_LOOP('',(#13789,#13790,#13791,#13792));
#3213=EDGE_LOOP('',(#13793,#13794,#13795,#13796));
#3214=EDGE_LOOP('',(#13797,#13798,#13799,#13800));
#3215=EDGE_LOOP('',(#13801,#13802,#13803,#13804));
#3216=EDGE_LOOP('',(#13805,#13806,#13807,#13808));
#3217=EDGE_LOOP('',(#13809,#13810,#13811,#13812));
#3218=EDGE_LOOP('',(#13813,#13814,#13815,#13816));
#3219=EDGE_LOOP('',(#13817,#13818,#13819,#13820));
#3220=EDGE_LOOP('',(#13821,#13822,#13823,#13824));
#3221=EDGE_LOOP('',(#13825,#13826,#13827,#13828));
#3222=EDGE_LOOP('',(#13829,#13830,#13831,#13832));
#3223=EDGE_LOOP('',(#13833,#13834,#13835,#13836));
#3224=EDGE_LOOP('',(#13837,#13838,#13839,#13840));
#3225=EDGE_LOOP('',(#13841,#13842,#13843,#13844));
#3226=EDGE_LOOP('',(#13845,#13846,#13847,#13848));
#3227=EDGE_LOOP('',(#13849,#13850,#13851,#13852));
#3228=EDGE_LOOP('',(#13853,#13854,#13855,#13856));
#3229=EDGE_LOOP('',(#13857,#13858,#13859,#13860));
#3230=EDGE_LOOP('',(#13861,#13862,#13863,#13864));
#3231=EDGE_LOOP('',(#13865,#13866,#13867,#13868));
#3232=EDGE_LOOP('',(#13869,#13870,#13871,#13872));
#3233=EDGE_LOOP('',(#13873,#13874,#13875,#13876));
#3234=EDGE_LOOP('',(#13877,#13878,#13879,#13880));
#3235=EDGE_LOOP('',(#13881,#13882,#13883,#13884));
#3236=EDGE_LOOP('',(#13885,#13886,#13887,#13888));
#3237=EDGE_LOOP('',(#13889,#13890,#13891,#13892));
#3238=EDGE_LOOP('',(#13893,#13894,#13895,#13896));
#3239=EDGE_LOOP('',(#13897,#13898,#13899,#13900));
#3240=EDGE_LOOP('',(#13901,#13902,#13903,#13904));
#3241=EDGE_LOOP('',(#13905,#13906,#13907,#13908));
#3242=EDGE_LOOP('',(#13909,#13910,#13911,#13912));
#3243=EDGE_LOOP('',(#13913,#13914,#13915,#13916));
#3244=EDGE_LOOP('',(#13917,#13918,#13919,#13920));
#3245=EDGE_LOOP('',(#13921,#13922,#13923,#13924));
#3246=EDGE_LOOP('',(#13925,#13926,#13927,#13928));
#3247=EDGE_LOOP('',(#13929));
#3248=EDGE_LOOP('',(#13930));
#3249=EDGE_LOOP('',(#13931,#13932,#13933,#13934));
#3250=EDGE_LOOP('',(#13935));
#3251=EDGE_LOOP('',(#13936));
#3252=EDGE_LOOP('',(#13937,#13938,#13939,#13940));
#3253=EDGE_LOOP('',(#13941,#13942,#13943,#13944));
#3254=EDGE_LOOP('',(#13945,#13946,#13947,#13948));
#3255=EDGE_LOOP('',(#13949,#13950,#13951,#13952));
#3256=EDGE_LOOP('',(#13953,#13954,#13955,#13956));
#3257=EDGE_LOOP('',(#13957,#13958,#13959,#13960));
#3258=EDGE_LOOP('',(#13961,#13962,#13963,#13964));
#3259=EDGE_LOOP('',(#13965,#13966,#13967,#13968));
#3260=EDGE_LOOP('',(#13969,#13970,#13971,#13972));
#3261=EDGE_LOOP('',(#13973,#13974,#13975,#13976));
#3262=EDGE_LOOP('',(#13977,#13978,#13979,#13980));
#3263=EDGE_LOOP('',(#13981,#13982,#13983,#13984));
#3264=EDGE_LOOP('',(#13985,#13986,#13987,#13988));
#3265=EDGE_LOOP('',(#13989,#13990,#13991,#13992));
#3266=EDGE_LOOP('',(#13993,#13994,#13995,#13996));
#3267=EDGE_LOOP('',(#13997,#13998,#13999,#14000));
#3268=EDGE_LOOP('',(#14001,#14002,#14003,#14004));
#3269=EDGE_LOOP('',(#14005,#14006,#14007,#14008));
#3270=EDGE_LOOP('',(#14009,#14010,#14011,#14012));
#3271=EDGE_LOOP('',(#14013,#14014,#14015,#14016));
#3272=EDGE_LOOP('',(#14017,#14018,#14019,#14020));
#3273=EDGE_LOOP('',(#14021,#14022,#14023,#14024));
#3274=EDGE_LOOP('',(#14025,#14026,#14027,#14028));
#3275=EDGE_LOOP('',(#14029,#14030,#14031,#14032));
#3276=EDGE_LOOP('',(#14033,#14034,#14035,#14036));
#3277=EDGE_LOOP('',(#14037,#14038,#14039,#14040));
#3278=EDGE_LOOP('',(#14041,#14042,#14043,#14044));
#3279=EDGE_LOOP('',(#14045,#14046,#14047,#14048));
#3280=EDGE_LOOP('',(#14049,#14050,#14051,#14052));
#3281=EDGE_LOOP('',(#14053,#14054,#14055,#14056));
#3282=EDGE_LOOP('',(#14057,#14058,#14059,#14060));
#3283=EDGE_LOOP('',(#14061,#14062,#14063,#14064));
#3284=EDGE_LOOP('',(#14065,#14066,#14067,#14068));
#3285=EDGE_LOOP('',(#14069,#14070,#14071,#14072));
#3286=EDGE_LOOP('',(#14073,#14074,#14075,#14076));
#3287=EDGE_LOOP('',(#14077,#14078,#14079,#14080));
#3288=EDGE_LOOP('',(#14081,#14082,#14083,#14084));
#3289=EDGE_LOOP('',(#14085,#14086,#14087,#14088));
#3290=EDGE_LOOP('',(#14089,#14090,#14091,#14092));
#3291=EDGE_LOOP('',(#14093,#14094,#14095,#14096));
#3292=EDGE_LOOP('',(#14097,#14098,#14099,#14100,#14101));
#3293=EDGE_LOOP('',(#14102,#14103,#14104,#14105));
#3294=EDGE_LOOP('',(#14106,#14107,#14108,#14109));
#3295=EDGE_LOOP('',(#14110,#14111,#14112,#14113));
#3296=EDGE_LOOP('',(#14114,#14115,#14116,#14117));
#3297=EDGE_LOOP('',(#14118,#14119,#14120,#14121));
#3298=EDGE_LOOP('',(#14122,#14123,#14124,#14125));
#3299=EDGE_LOOP('',(#14126,#14127,#14128,#14129));
#3300=EDGE_LOOP('',(#14130,#14131,#14132,#14133));
#3301=EDGE_LOOP('',(#14134,#14135,#14136,#14137));
#3302=EDGE_LOOP('',(#14138,#14139,#14140,#14141));
#3303=EDGE_LOOP('',(#14142,#14143,#14144,#14145));
#3304=EDGE_LOOP('',(#14146,#14147,#14148,#14149));
#3305=EDGE_LOOP('',(#14150,#14151,#14152,#14153));
#3306=EDGE_LOOP('',(#14154,#14155,#14156,#14157));
#3307=EDGE_LOOP('',(#14158,#14159,#14160,#14161));
#3308=EDGE_LOOP('',(#14162,#14163,#14164,#14165));
#3309=EDGE_LOOP('',(#14166,#14167,#14168,#14169));
#3310=EDGE_LOOP('',(#14170,#14171,#14172,#14173));
#3311=EDGE_LOOP('',(#14174,#14175,#14176,#14177));
#3312=EDGE_LOOP('',(#14178,#14179,#14180,#14181));
#3313=EDGE_LOOP('',(#14182,#14183,#14184,#14185));
#3314=EDGE_LOOP('',(#14186,#14187,#14188,#14189));
#3315=EDGE_LOOP('',(#14190,#14191,#14192,#14193));
#3316=EDGE_LOOP('',(#14194,#14195,#14196,#14197));
#3317=EDGE_LOOP('',(#14198,#14199,#14200,#14201));
#3318=EDGE_LOOP('',(#14202,#14203,#14204,#14205));
#3319=EDGE_LOOP('',(#14206,#14207,#14208,#14209));
#3320=EDGE_LOOP('',(#14210,#14211,#14212,#14213));
#3321=EDGE_LOOP('',(#14214,#14215,#14216,#14217));
#3322=EDGE_LOOP('',(#14218,#14219,#14220,#14221));
#3323=EDGE_LOOP('',(#14222,#14223,#14224,#14225));
#3324=EDGE_LOOP('',(#14226,#14227,#14228,#14229));
#3325=EDGE_LOOP('',(#14230,#14231,#14232,#14233));
#3326=EDGE_LOOP('',(#14234,#14235,#14236,#14237));
#3327=EDGE_LOOP('',(#14238,#14239,#14240,#14241));
#3328=EDGE_LOOP('',(#14242,#14243,#14244,#14245));
#3329=EDGE_LOOP('',(#14246,#14247,#14248,#14249));
#3330=EDGE_LOOP('',(#14250,#14251,#14252,#14253));
#3331=EDGE_LOOP('',(#14254,#14255,#14256,#14257));
#3332=EDGE_LOOP('',(#14258,#14259,#14260,#14261));
#3333=EDGE_LOOP('',(#14262,#14263,#14264,#14265));
#3334=EDGE_LOOP('',(#14266,#14267,#14268,#14269));
#3335=EDGE_LOOP('',(#14270,#14271,#14272,#14273));
#3336=EDGE_LOOP('',(#14274,#14275,#14276,#14277));
#3337=EDGE_LOOP('',(#14278,#14279,#14280,#14281));
#3338=EDGE_LOOP('',(#14282,#14283,#14284,#14285));
#3339=EDGE_LOOP('',(#14286,#14287,#14288,#14289));
#3340=EDGE_LOOP('',(#14290,#14291,#14292,#14293));
#3341=EDGE_LOOP('',(#14294,#14295,#14296,#14297));
#3342=EDGE_LOOP('',(#14298,#14299,#14300,#14301));
#3343=EDGE_LOOP('',(#14302,#14303,#14304,#14305));
#3344=EDGE_LOOP('',(#14306,#14307,#14308,#14309));
#3345=EDGE_LOOP('',(#14310,#14311,#14312,#14313));
#3346=EDGE_LOOP('',(#14314,#14315,#14316,#14317));
#3347=EDGE_LOOP('',(#14318,#14319,#14320,#14321));
#3348=EDGE_LOOP('',(#14322,#14323,#14324,#14325));
#3349=EDGE_LOOP('',(#14326,#14327,#14328,#14329));
#3350=EDGE_LOOP('',(#14330,#14331,#14332,#14333));
#3351=EDGE_LOOP('',(#14334,#14335,#14336,#14337));
#3352=EDGE_LOOP('',(#14338,#14339,#14340,#14341));
#3353=EDGE_LOOP('',(#14342,#14343,#14344,#14345));
#3354=EDGE_LOOP('',(#14346,#14347,#14348,#14349));
#3355=EDGE_LOOP('',(#14350,#14351,#14352,#14353));
#3356=EDGE_LOOP('',(#14354,#14355,#14356,#14357));
#3357=EDGE_LOOP('',(#14358,#14359,#14360,#14361));
#3358=EDGE_LOOP('',(#14362,#14363,#14364,#14365));
#3359=EDGE_LOOP('',(#14366,#14367,#14368,#14369));
#3360=EDGE_LOOP('',(#14370,#14371,#14372,#14373));
#3361=EDGE_LOOP('',(#14374,#14375,#14376,#14377));
#3362=EDGE_LOOP('',(#14378,#14379,#14380,#14381));
#3363=EDGE_LOOP('',(#14382,#14383,#14384,#14385));
#3364=EDGE_LOOP('',(#14386,#14387,#14388,#14389));
#3365=EDGE_LOOP('',(#14390,#14391,#14392,#14393));
#3366=EDGE_LOOP('',(#14394,#14395,#14396,#14397));
#3367=EDGE_LOOP('',(#14398,#14399,#14400,#14401));
#3368=EDGE_LOOP('',(#14402,#14403,#14404,#14405));
#3369=EDGE_LOOP('',(#14406,#14407,#14408,#14409));
#3370=EDGE_LOOP('',(#14410,#14411,#14412,#14413));
#3371=EDGE_LOOP('',(#14414,#14415,#14416,#14417,#14418));
#3372=EDGE_LOOP('',(#14419,#14420,#14421,#14422));
#3373=EDGE_LOOP('',(#14423,#14424,#14425,#14426));
#3374=EDGE_LOOP('',(#14427,#14428,#14429,#14430));
#3375=EDGE_LOOP('',(#14431,#14432,#14433,#14434));
#3376=EDGE_LOOP('',(#14435,#14436,#14437,#14438));
#3377=EDGE_LOOP('',(#14439,#14440,#14441,#14442));
#3378=EDGE_LOOP('',(#14443,#14444,#14445,#14446));
#3379=EDGE_LOOP('',(#14447,#14448,#14449,#14450));
#3380=EDGE_LOOP('',(#14451,#14452,#14453,#14454));
#3381=EDGE_LOOP('',(#14455,#14456,#14457,#14458));
#3382=EDGE_LOOP('',(#14459,#14460,#14461,#14462));
#3383=EDGE_LOOP('',(#14463,#14464,#14465,#14466));
#3384=EDGE_LOOP('',(#14467,#14468,#14469,#14470));
#3385=EDGE_LOOP('',(#14471,#14472,#14473,#14474));
#3386=EDGE_LOOP('',(#14475,#14476,#14477,#14478));
#3387=EDGE_LOOP('',(#14479,#14480,#14481,#14482));
#3388=EDGE_LOOP('',(#14483,#14484,#14485,#14486));
#3389=EDGE_LOOP('',(#14487,#14488,#14489,#14490));
#3390=EDGE_LOOP('',(#14491,#14492,#14493,#14494));
#3391=EDGE_LOOP('',(#14495,#14496,#14497,#14498));
#3392=EDGE_LOOP('',(#14499,#14500,#14501,#14502));
#3393=EDGE_LOOP('',(#14503,#14504,#14505,#14506));
#3394=EDGE_LOOP('',(#14507,#14508,#14509,#14510));
#3395=EDGE_LOOP('',(#14511,#14512,#14513,#14514));
#3396=EDGE_LOOP('',(#14515,#14516,#14517,#14518));
#3397=EDGE_LOOP('',(#14519,#14520,#14521,#14522));
#3398=EDGE_LOOP('',(#14523,#14524,#14525,#14526));
#3399=EDGE_LOOP('',(#14527,#14528,#14529,#14530));
#3400=EDGE_LOOP('',(#14531,#14532,#14533,#14534));
#3401=EDGE_LOOP('',(#14535,#14536,#14537,#14538));
#3402=EDGE_LOOP('',(#14539,#14540,#14541,#14542));
#3403=EDGE_LOOP('',(#14543,#14544,#14545,#14546));
#3404=EDGE_LOOP('',(#14547,#14548,#14549,#14550));
#3405=EDGE_LOOP('',(#14551,#14552,#14553,#14554));
#3406=EDGE_LOOP('',(#14555,#14556,#14557,#14558,#14559,#14560,#14561,#14562,
#14563,#14564,#14565,#14566,#14567));
#3407=EDGE_LOOP('',(#14568,#14569,#14570,#14571,#14572));
#3408=EDGE_LOOP('',(#14573,#14574,#14575,#14576));
#3409=EDGE_LOOP('',(#14577,#14578));
#3410=EDGE_LOOP('',(#14579));
#3411=EDGE_LOOP('',(#14580,#14581));
#3412=EDGE_LOOP('',(#14582));
#3413=EDGE_LOOP('',(#14583));
#3414=EDGE_LOOP('',(#14584,#14585,#14586,#14587));
#3415=EDGE_LOOP('',(#14588,#14589,#14590,#14591));
#3416=EDGE_LOOP('',(#14592,#14593,#14594,#14595,#14596));
#3417=EDGE_LOOP('',(#14597,#14598,#14599,#14600));
#3418=EDGE_LOOP('',(#14601,#14602,#14603,#14604,#14605));
#3419=EDGE_LOOP('',(#14606,#14607,#14608,#14609,#14610,#14611));
#3420=EDGE_LOOP('',(#14612,#14613,#14614,#14615,#14616,#14617));
#3421=EDGE_LOOP('',(#14618,#14619,#14620,#14621,#14622,#14623));
#3422=EDGE_LOOP('',(#14624,#14625,#14626,#14627,#14628,#14629));
#3423=EDGE_LOOP('',(#14630,#14631,#14632,#14633,#14634,#14635));
#3424=EDGE_LOOP('',(#14636,#14637,#14638,#14639,#14640,#14641));
#3425=EDGE_LOOP('',(#14642,#14643,#14644,#14645,#14646,#14647));
#3426=EDGE_LOOP('',(#14648,#14649,#14650,#14651,#14652,#14653));
#3427=EDGE_LOOP('',(#14654,#14655,#14656,#14657,#14658,#14659));
#3428=EDGE_LOOP('',(#14660,#14661,#14662,#14663,#14664,#14665));
#3429=EDGE_LOOP('',(#14666,#14667,#14668,#14669,#14670,#14671));
#3430=EDGE_LOOP('',(#14672,#14673,#14674,#14675,#14676,#14677));
#3431=EDGE_LOOP('',(#14678,#14679,#14680,#14681,#14682,#14683));
#3432=EDGE_LOOP('',(#14684,#14685,#14686,#14687,#14688,#14689));
#3433=EDGE_LOOP('',(#14690,#14691,#14692,#14693,#14694,#14695));
#3434=EDGE_LOOP('',(#14696,#14697,#14698,#14699,#14700,#14701));
#3435=EDGE_LOOP('',(#14702,#14703,#14704,#14705,#14706,#14707));
#3436=EDGE_LOOP('',(#14708,#14709,#14710,#14711,#14712,#14713));
#3437=EDGE_LOOP('',(#14714,#14715,#14716,#14717,#14718,#14719));
#3438=EDGE_LOOP('',(#14720,#14721,#14722,#14723,#14724,#14725));
#3439=EDGE_LOOP('',(#14726,#14727,#14728,#14729,#14730,#14731));
#3440=EDGE_LOOP('',(#14732,#14733,#14734,#14735,#14736,#14737));
#3441=EDGE_LOOP('',(#14738,#14739,#14740,#14741,#14742,#14743));
#3442=EDGE_LOOP('',(#14744,#14745,#14746,#14747,#14748,#14749));
#3443=EDGE_LOOP('',(#14750,#14751,#14752,#14753,#14754,#14755));
#3444=EDGE_LOOP('',(#14756,#14757,#14758,#14759,#14760,#14761));
#3445=EDGE_LOOP('',(#14762,#14763,#14764,#14765,#14766,#14767));
#3446=EDGE_LOOP('',(#14768,#14769,#14770,#14771,#14772,#14773));
#3447=EDGE_LOOP('',(#14774,#14775,#14776,#14777,#14778,#14779));
#3448=EDGE_LOOP('',(#14780,#14781,#14782,#14783,#14784,#14785));
#3449=EDGE_LOOP('',(#14786,#14787,#14788,#14789,#14790,#14791));
#3450=EDGE_LOOP('',(#14792,#14793,#14794,#14795,#14796,#14797));
#3451=EDGE_LOOP('',(#14798,#14799,#14800,#14801,#14802,#14803));
#3452=EDGE_LOOP('',(#14804,#14805,#14806,#14807,#14808,#14809));
#3453=EDGE_LOOP('',(#14810,#14811,#14812,#14813,#14814,#14815));
#3454=EDGE_LOOP('',(#14816,#14817,#14818,#14819,#14820,#14821));
#3455=EDGE_LOOP('',(#14822,#14823,#14824,#14825,#14826,#14827));
#3456=EDGE_LOOP('',(#14828,#14829,#14830,#14831,#14832,#14833));
#3457=EDGE_LOOP('',(#14834,#14835,#14836,#14837));
#3458=EDGE_LOOP('',(#14838,#14839,#14840,#14841,#14842,#14843,#14844,#14845,
#14846,#14847,#14848,#14849,#14850,#14851,#14852,#14853,#14854,#14855,#14856,
#14857,#14858,#14859,#14860,#14861,#14862,#14863,#14864,#14865,#14866,#14867,
#14868,#14869,#14870,#14871,#14872,#14873,#14874,#14875,#14876,#14877,#14878,
#14879,#14880,#14881,#14882,#14883,#14884,#14885,#14886,#14887,#14888,#14889,
#14890,#14891,#14892,#14893,#14894,#14895,#14896,#14897,#14898,#14899,#14900,
#14901,#14902,#14903,#14904,#14905,#14906,#14907,#14908,#14909,#14910,#14911,
#14912,#14913,#14914,#14915,#14916,#14917,#14918,#14919,#14920,#14921,#14922,
#14923,#14924,#14925,#14926,#14927,#14928,#14929,#14930,#14931,#14932,#14933,
#14934,#14935,#14936,#14937,#14938,#14939,#14940,#14941,#14942,#14943,#14944,
#14945,#14946,#14947,#14948,#14949,#14950,#14951,#14952,#14953,#14954,#14955,
#14956,#14957,#14958,#14959,#14960,#14961,#14962,#14963,#14964,#14965,#14966,
#14967,#14968,#14969,#14970,#14971,#14972,#14973,#14974,#14975,#14976,#14977,
#14978,#14979,#14980,#14981,#14982,#14983,#14984,#14985,#14986,#14987,#14988,
#14989,#14990,#14991,#14992,#14993,#14994,#14995,#14996,#14997,#14998,#14999,
#15000,#15001,#15002,#15003,#15004,#15005,#15006,#15007,#15008,#15009,#15010,
#15011,#15012,#15013,#15014,#15015,#15016,#15017,#15018,#15019,#15020,#15021,
#15022,#15023,#15024,#15025,#15026,#15027,#15028,#15029,#15030,#15031,#15032,
#15033,#15034,#15035,#15036,#15037,#15038,#15039,#15040,#15041,#15042,#15043,
#15044,#15045,#15046,#15047,#15048,#15049,#15050,#15051,#15052,#15053,#15054,
#15055,#15056,#15057,#15058,#15059,#15060,#15061,#15062,#15063,#15064,#15065,
#15066,#15067,#15068,#15069,#15070,#15071,#15072));
#3459=EDGE_LOOP('',(#15073,#15074,#15075,#15076,#15077,#15078,#15079,#15080,
#15081,#15082,#15083,#15084,#15085,#15086,#15087,#15088,#15089,#15090,#15091,
#15092,#15093,#15094,#15095,#15096,#15097,#15098,#15099,#15100,#15101,#15102,
#15103,#15104,#15105,#15106,#15107,#15108,#15109,#15110,#15111,#15112,#15113,
#15114,#15115,#15116,#15117,#15118,#15119,#15120,#15121,#15122,#15123,#15124,
#15125,#15126,#15127,#15128,#15129,#15130,#15131,#15132,#15133,#15134,#15135,
#15136,#15137,#15138,#15139,#15140,#15141,#15142,#15143,#15144,#15145,#15146,
#15147,#15148,#15149,#15150,#15151,#15152,#15153,#15154,#15155,#15156,#15157,
#15158,#15159,#15160,#15161,#15162,#15163,#15164,#15165,#15166,#15167,#15168,
#15169,#15170,#15171,#15172,#15173,#15174,#15175,#15176,#15177,#15178,#15179,
#15180,#15181,#15182,#15183,#15184,#15185,#15186,#15187,#15188,#15189,#15190,
#15191,#15192,#15193,#15194,#15195,#15196,#15197,#15198,#15199,#15200,#15201,
#15202,#15203,#15204,#15205,#15206,#15207,#15208,#15209,#15210,#15211,#15212,
#15213,#15214,#15215,#15216,#15217,#15218,#15219,#15220,#15221,#15222,#15223,
#15224,#15225,#15226,#15227,#15228,#15229,#15230,#15231,#15232,#15233,#15234,
#15235,#15236,#15237,#15238,#15239,#15240,#15241,#15242,#15243,#15244,#15245,
#15246,#15247,#15248,#15249,#15250,#15251,#15252,#15253,#15254,#15255,#15256,
#15257,#15258,#15259,#15260,#15261,#15262,#15263,#15264,#15265,#15266,#15267,
#15268,#15269,#15270,#15271,#15272,#15273,#15274,#15275,#15276,#15277,#15278,
#15279,#15280,#15281,#15282,#15283,#15284,#15285,#15286,#15287,#15288,#15289,
#15290,#15291,#15292,#15293,#15294,#15295,#15296,#15297,#15298,#15299,#15300,
#15301,#15302,#15303,#15304,#15305,#15306,#15307));
#3460=EDGE_LOOP('',(#15308,#15309,#15310,#15311,#15312));
#3461=EDGE_LOOP('',(#15313,#15314,#15315,#15316));
#3462=EDGE_LOOP('',(#15317,#15318,#15319,#15320));
#3463=EDGE_LOOP('',(#15321,#15322,#15323,#15324));
#3464=EDGE_LOOP('',(#15325,#15326,#15327,#15328));
#3465=EDGE_LOOP('',(#15329,#15330,#15331,#15332));
#3466=EDGE_LOOP('',(#15333,#15334,#15335,#15336));
#3467=EDGE_LOOP('',(#15337,#15338,#15339,#15340));
#3468=EDGE_LOOP('',(#15341,#15342,#15343,#15344));
#3469=EDGE_LOOP('',(#15345,#15346,#15347,#15348));
#3470=EDGE_LOOP('',(#15349,#15350,#15351,#15352));
#3471=EDGE_LOOP('',(#15353,#15354,#15355,#15356));
#3472=EDGE_LOOP('',(#15357,#15358,#15359,#15360));
#3473=EDGE_LOOP('',(#15361,#15362,#15363,#15364));
#3474=EDGE_LOOP('',(#15365,#15366,#15367,#15368));
#3475=EDGE_LOOP('',(#15369,#15370,#15371,#15372));
#3476=EDGE_LOOP('',(#15373,#15374,#15375,#15376));
#3477=EDGE_LOOP('',(#15377,#15378,#15379,#15380));
#3478=EDGE_LOOP('',(#15381,#15382,#15383,#15384));
#3479=EDGE_LOOP('',(#15385,#15386,#15387,#15388));
#3480=EDGE_LOOP('',(#15389,#15390,#15391,#15392));
#3481=EDGE_LOOP('',(#15393,#15394,#15395,#15396));
#3482=EDGE_LOOP('',(#15397,#15398,#15399,#15400));
#3483=EDGE_LOOP('',(#15401,#15402,#15403,#15404));
#3484=EDGE_LOOP('',(#15405,#15406,#15407,#15408));
#3485=EDGE_LOOP('',(#15409,#15410,#15411,#15412));
#3486=EDGE_LOOP('',(#15413,#15414,#15415,#15416));
#3487=EDGE_LOOP('',(#15417,#15418,#15419,#15420));
#3488=EDGE_LOOP('',(#15421,#15422,#15423,#15424));
#3489=EDGE_LOOP('',(#15425,#15426,#15427,#15428));
#3490=EDGE_LOOP('',(#15429,#15430,#15431,#15432));
#3491=EDGE_LOOP('',(#15433,#15434,#15435,#15436));
#3492=EDGE_LOOP('',(#15437,#15438,#15439,#15440));
#3493=EDGE_LOOP('',(#15441,#15442,#15443,#15444));
#3494=EDGE_LOOP('',(#15445,#15446,#15447,#15448));
#3495=EDGE_LOOP('',(#15449,#15450,#15451,#15452));
#3496=EDGE_LOOP('',(#15453,#15454,#15455,#15456));
#3497=EDGE_LOOP('',(#15457,#15458,#15459,#15460));
#3498=EDGE_LOOP('',(#15461,#15462,#15463,#15464));
#3499=EDGE_LOOP('',(#15465,#15466,#15467,#15468));
#3500=EDGE_LOOP('',(#15469,#15470,#15471,#15472));
#3501=EDGE_LOOP('',(#15473,#15474,#15475,#15476));
#3502=EDGE_LOOP('',(#15477,#15478,#15479,#15480));
#3503=EDGE_LOOP('',(#15481,#15482,#15483,#15484));
#3504=EDGE_LOOP('',(#15485,#15486,#15487,#15488));
#3505=EDGE_LOOP('',(#15489,#15490,#15491,#15492));
#3506=EDGE_LOOP('',(#15493,#15494,#15495,#15496));
#3507=EDGE_LOOP('',(#15497,#15498,#15499,#15500));
#3508=EDGE_LOOP('',(#15501,#15502,#15503,#15504));
#3509=EDGE_LOOP('',(#15505,#15506,#15507,#15508));
#3510=EDGE_LOOP('',(#15509,#15510,#15511,#15512));
#3511=EDGE_LOOP('',(#15513,#15514,#15515,#15516));
#3512=EDGE_LOOP('',(#15517,#15518,#15519,#15520));
#3513=EDGE_LOOP('',(#15521,#15522,#15523,#15524));
#3514=EDGE_LOOP('',(#15525,#15526,#15527,#15528));
#3515=EDGE_LOOP('',(#15529,#15530,#15531,#15532));
#3516=EDGE_LOOP('',(#15533,#15534,#15535,#15536));
#3517=EDGE_LOOP('',(#15537,#15538,#15539,#15540));
#3518=EDGE_LOOP('',(#15541,#15542,#15543,#15544));
#3519=EDGE_LOOP('',(#15545,#15546,#15547,#15548));
#3520=EDGE_LOOP('',(#15549,#15550,#15551,#15552));
#3521=EDGE_LOOP('',(#15553,#15554,#15555,#15556));
#3522=EDGE_LOOP('',(#15557,#15558,#15559,#15560));
#3523=EDGE_LOOP('',(#15561,#15562,#15563,#15564));
#3524=EDGE_LOOP('',(#15565,#15566,#15567,#15568));
#3525=EDGE_LOOP('',(#15569,#15570,#15571,#15572));
#3526=EDGE_LOOP('',(#15573,#15574,#15575,#15576));
#3527=EDGE_LOOP('',(#15577,#15578,#15579,#15580));
#3528=EDGE_LOOP('',(#15581,#15582,#15583,#15584));
#3529=EDGE_LOOP('',(#15585,#15586,#15587,#15588));
#3530=EDGE_LOOP('',(#15589,#15590,#15591,#15592));
#3531=EDGE_LOOP('',(#15593,#15594,#15595,#15596));
#3532=EDGE_LOOP('',(#15597,#15598,#15599,#15600));
#3533=EDGE_LOOP('',(#15601,#15602,#15603,#15604));
#3534=EDGE_LOOP('',(#15605,#15606,#15607,#15608));
#3535=EDGE_LOOP('',(#15609,#15610,#15611,#15612));
#3536=EDGE_LOOP('',(#15613,#15614,#15615,#15616));
#3537=EDGE_LOOP('',(#15617));
#3538=EDGE_LOOP('',(#15618,#15619,#15620,#15621));
#3539=EDGE_LOOP('',(#15622));
#3540=EDGE_LOOP('',(#15623));
#3541=EDGE_LOOP('',(#15624));
#3542=EDGE_LOOP('',(#15625));
#3543=EDGE_LOOP('',(#15626));
#3544=EDGE_LOOP('',(#15627,#15628,#15629,#15630));
#3545=EDGE_LOOP('',(#15631,#15632,#15633,#15634));
#3546=EDGE_LOOP('',(#15635,#15636,#15637,#15638));
#3547=EDGE_LOOP('',(#15639,#15640,#15641,#15642));
#3548=EDGE_LOOP('',(#15643,#15644,#15645,#15646));
#3549=EDGE_LOOP('',(#15647,#15648,#15649,#15650));
#3550=EDGE_LOOP('',(#15651,#15652,#15653,#15654));
#3551=EDGE_LOOP('',(#15655,#15656,#15657,#15658));
#3552=EDGE_LOOP('',(#15659,#15660,#15661,#15662));
#3553=EDGE_LOOP('',(#15663,#15664,#15665,#15666));
#3554=EDGE_LOOP('',(#15667,#15668,#15669,#15670));
#3555=EDGE_LOOP('',(#15671,#15672,#15673,#15674));
#3556=EDGE_LOOP('',(#15675,#15676,#15677,#15678));
#3557=EDGE_LOOP('',(#15679,#15680,#15681,#15682));
#3558=EDGE_LOOP('',(#15683,#15684,#15685,#15686));
#3559=EDGE_LOOP('',(#15687,#15688,#15689,#15690));
#3560=EDGE_LOOP('',(#15691,#15692,#15693,#15694));
#3561=EDGE_LOOP('',(#15695,#15696,#15697,#15698));
#3562=EDGE_LOOP('',(#15699,#15700,#15701,#15702));
#3563=EDGE_LOOP('',(#15703,#15704,#15705,#15706));
#3564=EDGE_LOOP('',(#15707,#15708,#15709,#15710));
#3565=EDGE_LOOP('',(#15711,#15712,#15713,#15714));
#3566=EDGE_LOOP('',(#15715,#15716,#15717,#15718));
#3567=EDGE_LOOP('',(#15719,#15720,#15721,#15722));
#3568=EDGE_LOOP('',(#15723,#15724,#15725,#15726));
#3569=EDGE_LOOP('',(#15727,#15728,#15729,#15730));
#3570=EDGE_LOOP('',(#15731,#15732,#15733,#15734));
#3571=EDGE_LOOP('',(#15735,#15736,#15737,#15738));
#3572=EDGE_LOOP('',(#15739,#15740,#15741,#15742));
#3573=EDGE_LOOP('',(#15743,#15744,#15745,#15746));
#3574=EDGE_LOOP('',(#15747,#15748,#15749,#15750));
#3575=EDGE_LOOP('',(#15751,#15752,#15753,#15754));
#3576=EDGE_LOOP('',(#15755,#15756,#15757,#15758));
#3577=EDGE_LOOP('',(#15759,#15760,#15761,#15762));
#3578=EDGE_LOOP('',(#15763,#15764,#15765,#15766));
#3579=EDGE_LOOP('',(#15767,#15768,#15769,#15770));
#3580=EDGE_LOOP('',(#15771,#15772,#15773,#15774));
#3581=EDGE_LOOP('',(#15775,#15776,#15777,#15778));
#3582=EDGE_LOOP('',(#15779,#15780,#15781,#15782));
#3583=EDGE_LOOP('',(#15783,#15784,#15785,#15786));
#3584=EDGE_LOOP('',(#15787,#15788,#15789,#15790,#15791));
#3585=EDGE_LOOP('',(#15792,#15793,#15794,#15795));
#3586=EDGE_LOOP('',(#15796,#15797,#15798,#15799));
#3587=EDGE_LOOP('',(#15800,#15801,#15802,#15803));
#3588=EDGE_LOOP('',(#15804,#15805,#15806,#15807));
#3589=EDGE_LOOP('',(#15808,#15809,#15810,#15811));
#3590=EDGE_LOOP('',(#15812,#15813,#15814,#15815));
#3591=EDGE_LOOP('',(#15816,#15817,#15818,#15819));
#3592=EDGE_LOOP('',(#15820,#15821,#15822,#15823));
#3593=EDGE_LOOP('',(#15824,#15825,#15826,#15827));
#3594=EDGE_LOOP('',(#15828,#15829,#15830,#15831));
#3595=EDGE_LOOP('',(#15832,#15833,#15834,#15835));
#3596=EDGE_LOOP('',(#15836,#15837,#15838,#15839));
#3597=EDGE_LOOP('',(#15840,#15841,#15842,#15843));
#3598=EDGE_LOOP('',(#15844,#15845,#15846,#15847));
#3599=EDGE_LOOP('',(#15848,#15849,#15850,#15851));
#3600=EDGE_LOOP('',(#15852,#15853,#15854,#15855));
#3601=EDGE_LOOP('',(#15856,#15857,#15858,#15859));
#3602=EDGE_LOOP('',(#15860,#15861,#15862,#15863));
#3603=EDGE_LOOP('',(#15864,#15865,#15866,#15867));
#3604=EDGE_LOOP('',(#15868,#15869,#15870,#15871));
#3605=EDGE_LOOP('',(#15872,#15873,#15874,#15875));
#3606=EDGE_LOOP('',(#15876,#15877,#15878,#15879));
#3607=EDGE_LOOP('',(#15880,#15881,#15882,#15883));
#3608=EDGE_LOOP('',(#15884,#15885,#15886,#15887));
#3609=EDGE_LOOP('',(#15888,#15889,#15890,#15891));
#3610=EDGE_LOOP('',(#15892,#15893,#15894,#15895));
#3611=EDGE_LOOP('',(#15896,#15897,#15898,#15899));
#3612=EDGE_LOOP('',(#15900,#15901,#15902,#15903));
#3613=EDGE_LOOP('',(#15904,#15905,#15906,#15907));
#3614=EDGE_LOOP('',(#15908,#15909,#15910,#15911));
#3615=EDGE_LOOP('',(#15912,#15913,#15914,#15915));
#3616=EDGE_LOOP('',(#15916,#15917,#15918,#15919));
#3617=EDGE_LOOP('',(#15920,#15921,#15922,#15923));
#3618=EDGE_LOOP('',(#15924,#15925,#15926,#15927));
#3619=EDGE_LOOP('',(#15928,#15929,#15930,#15931));
#3620=EDGE_LOOP('',(#15932,#15933,#15934,#15935));
#3621=EDGE_LOOP('',(#15936,#15937,#15938,#15939));
#3622=EDGE_LOOP('',(#15940,#15941,#15942,#15943));
#3623=EDGE_LOOP('',(#15944,#15945,#15946,#15947));
#3624=EDGE_LOOP('',(#15948,#15949,#15950,#15951));
#3625=EDGE_LOOP('',(#15952,#15953,#15954,#15955));
#3626=EDGE_LOOP('',(#15956,#15957,#15958,#15959));
#3627=EDGE_LOOP('',(#15960,#15961,#15962,#15963));
#3628=EDGE_LOOP('',(#15964,#15965,#15966,#15967));
#3629=EDGE_LOOP('',(#15968,#15969,#15970,#15971));
#3630=EDGE_LOOP('',(#15972,#15973,#15974,#15975));
#3631=EDGE_LOOP('',(#15976,#15977,#15978,#15979));
#3632=EDGE_LOOP('',(#15980,#15981,#15982,#15983));
#3633=EDGE_LOOP('',(#15984,#15985,#15986,#15987));
#3634=EDGE_LOOP('',(#15988,#15989,#15990,#15991));
#3635=EDGE_LOOP('',(#15992,#15993,#15994,#15995));
#3636=EDGE_LOOP('',(#15996,#15997,#15998,#15999));
#3637=EDGE_LOOP('',(#16000,#16001,#16002,#16003));
#3638=EDGE_LOOP('',(#16004,#16005,#16006,#16007));
#3639=EDGE_LOOP('',(#16008,#16009,#16010,#16011));
#3640=EDGE_LOOP('',(#16012,#16013,#16014,#16015));
#3641=EDGE_LOOP('',(#16016,#16017,#16018,#16019));
#3642=EDGE_LOOP('',(#16020,#16021,#16022,#16023));
#3643=EDGE_LOOP('',(#16024,#16025,#16026,#16027));
#3644=EDGE_LOOP('',(#16028,#16029,#16030,#16031));
#3645=EDGE_LOOP('',(#16032,#16033,#16034,#16035));
#3646=EDGE_LOOP('',(#16036,#16037,#16038,#16039));
#3647=EDGE_LOOP('',(#16040,#16041,#16042,#16043));
#3648=EDGE_LOOP('',(#16044,#16045,#16046,#16047));
#3649=EDGE_LOOP('',(#16048,#16049,#16050,#16051));
#3650=EDGE_LOOP('',(#16052,#16053,#16054,#16055));
#3651=EDGE_LOOP('',(#16056,#16057,#16058,#16059));
#3652=EDGE_LOOP('',(#16060,#16061,#16062,#16063));
#3653=EDGE_LOOP('',(#16064,#16065,#16066,#16067));
#3654=EDGE_LOOP('',(#16068,#16069,#16070,#16071));
#3655=EDGE_LOOP('',(#16072,#16073,#16074,#16075));
#3656=EDGE_LOOP('',(#16076,#16077,#16078,#16079));
#3657=EDGE_LOOP('',(#16080,#16081,#16082,#16083));
#3658=EDGE_LOOP('',(#16084,#16085,#16086,#16087));
#3659=EDGE_LOOP('',(#16088,#16089,#16090,#16091));
#3660=EDGE_LOOP('',(#16092,#16093,#16094,#16095));
#3661=EDGE_LOOP('',(#16096,#16097,#16098,#16099));
#3662=EDGE_LOOP('',(#16100,#16101,#16102,#16103));
#3663=EDGE_LOOP('',(#16104,#16105,#16106,#16107,#16108));
#3664=EDGE_LOOP('',(#16109,#16110,#16111,#16112));
#3665=EDGE_LOOP('',(#16113,#16114,#16115,#16116));
#3666=EDGE_LOOP('',(#16117,#16118,#16119,#16120));
#3667=EDGE_LOOP('',(#16121,#16122,#16123,#16124));
#3668=EDGE_LOOP('',(#16125,#16126,#16127,#16128));
#3669=EDGE_LOOP('',(#16129,#16130,#16131,#16132));
#3670=EDGE_LOOP('',(#16133,#16134,#16135,#16136));
#3671=EDGE_LOOP('',(#16137,#16138,#16139,#16140));
#3672=EDGE_LOOP('',(#16141,#16142,#16143,#16144));
#3673=EDGE_LOOP('',(#16145,#16146,#16147,#16148));
#3674=EDGE_LOOP('',(#16149,#16150,#16151,#16152));
#3675=EDGE_LOOP('',(#16153,#16154,#16155,#16156));
#3676=EDGE_LOOP('',(#16157,#16158,#16159,#16160));
#3677=EDGE_LOOP('',(#16161,#16162,#16163,#16164));
#3678=EDGE_LOOP('',(#16165,#16166,#16167,#16168));
#3679=EDGE_LOOP('',(#16169,#16170,#16171,#16172));
#3680=EDGE_LOOP('',(#16173,#16174,#16175,#16176));
#3681=EDGE_LOOP('',(#16177,#16178,#16179,#16180));
#3682=EDGE_LOOP('',(#16181,#16182,#16183,#16184));
#3683=EDGE_LOOP('',(#16185,#16186,#16187,#16188));
#3684=EDGE_LOOP('',(#16189,#16190,#16191,#16192));
#3685=EDGE_LOOP('',(#16193,#16194,#16195,#16196));
#3686=EDGE_LOOP('',(#16197,#16198,#16199,#16200));
#3687=EDGE_LOOP('',(#16201,#16202,#16203,#16204));
#3688=EDGE_LOOP('',(#16205,#16206,#16207,#16208));
#3689=EDGE_LOOP('',(#16209,#16210,#16211,#16212));
#3690=EDGE_LOOP('',(#16213,#16214,#16215,#16216));
#3691=EDGE_LOOP('',(#16217,#16218,#16219,#16220));
#3692=EDGE_LOOP('',(#16221,#16222,#16223,#16224));
#3693=EDGE_LOOP('',(#16225,#16226,#16227,#16228));
#3694=EDGE_LOOP('',(#16229,#16230,#16231,#16232));
#3695=EDGE_LOOP('',(#16233,#16234,#16235,#16236));
#3696=EDGE_LOOP('',(#16237,#16238,#16239,#16240));
#3697=EDGE_LOOP('',(#16241,#16242,#16243,#16244));
#3944=LINE('',#33364,#4888);
#3945=LINE('',#33372,#4889);
#3946=LINE('',#33380,#4890);
#3947=LINE('',#33386,#4891);
#3948=LINE('',#33407,#4892);
#3949=LINE('',#33415,#4893);
#3950=LINE('',#33421,#4894);
#3951=LINE('',#33427,#4895);
#3952=LINE('',#33444,#4896);
#3953=LINE('',#33479,#4897);
#3954=LINE('',#33481,#4898);
#3955=LINE('',#33483,#4899);
#3956=LINE('',#33484,#4900);
#3957=LINE('',#33485,#4901);
#3958=LINE('',#33487,#4902);
#3959=LINE('',#33489,#4903);
#3960=LINE('',#33493,#4904);
#3961=LINE('',#33495,#4905);
#3962=LINE('',#33497,#4906);
#3963=LINE('',#33498,#4907);
#3964=LINE('',#33502,#4908);
#3965=LINE('',#33504,#4909);
#3966=LINE('',#33506,#4910);
#3967=LINE('',#33507,#4911);
#3968=LINE('',#33510,#4912);
#3969=LINE('',#33514,#4913);
#3970=LINE('',#33516,#4914);
#3971=LINE('',#33517,#4915);
#3972=LINE('',#33519,#4916);
#3973=LINE('',#33521,#4917);
#3974=LINE('',#33523,#4918);
#3975=LINE('',#33525,#4919);
#3976=LINE('',#33527,#4920);
#3977=LINE('',#33529,#4921);
#3978=LINE('',#33531,#4922);
#3979=LINE('',#33534,#4923);
#3980=LINE('',#33537,#4924);
#3981=LINE('',#33539,#4925);
#3982=LINE('',#33540,#4926);
#3983=LINE('',#33543,#4927);
#3984=LINE('',#33545,#4928);
#3985=LINE('',#33549,#4929);
#3986=LINE('',#33551,#4930);
#3987=LINE('',#33552,#4931);
#3988=LINE('',#33554,#4932);
#3989=LINE('',#33556,#4933);
#3990=LINE('',#33558,#4934);
#3991=LINE('',#33560,#4935);
#3992=LINE('',#33562,#4936);
#3993=LINE('',#33564,#4937);
#3994=LINE('',#33565,#4938);
#3995=LINE('',#33567,#4939);
#3996=LINE('',#33569,#4940);
#3997=LINE('',#33571,#4941);
#3998=LINE('',#33576,#4942);
#3999=LINE('',#33578,#4943);
#4000=LINE('',#33580,#4944);
#4001=LINE('',#33581,#4945);
#4002=LINE('',#33585,#4946);
#4003=LINE('',#33587,#4947);
#4004=LINE('',#33589,#4948);
#4005=LINE('',#33591,#4949);
#4006=LINE('',#33593,#4950);
#4007=LINE('',#33594,#4951);
#4008=LINE('',#33595,#4952);
#4009=LINE('',#33599,#4953);
#4010=LINE('',#33601,#4954);
#4011=LINE('',#33603,#4955);
#4012=LINE('',#33605,#4956);
#4013=LINE('',#33609,#4957);
#4014=LINE('',#33610,#4958);
#4015=LINE('',#33614,#4959);
#4016=LINE('',#33616,#4960);
#4017=LINE('',#33618,#4961);
#4018=LINE('',#33620,#4962);
#4019=LINE('',#33624,#4963);
#4020=LINE('',#33626,#4964);
#4021=LINE('',#33628,#4965);
#4022=LINE('',#33629,#4966);
#4023=LINE('',#33633,#4967);
#4024=LINE('',#33637,#4968);
#4025=LINE('',#33651,#4969);
#4026=LINE('',#33663,#4970);
#4027=LINE('',#33675,#4971);
#4028=LINE('',#33677,#4972);
#4029=LINE('',#33680,#4973);
#4030=LINE('',#33682,#4974);
#4031=LINE('',#33694,#4975);
#4032=LINE('',#33696,#4976);
#4033=LINE('',#33700,#4977);
#4034=LINE('',#33701,#4978);
#4035=LINE('',#33704,#4979);
#4036=LINE('',#33705,#4980);
#4037=LINE('',#33708,#4981);
#4038=LINE('',#33710,#4982);
#4039=LINE('',#33711,#4983);
#4040=LINE('',#33714,#4984);
#4041=LINE('',#33715,#4985);
#4042=LINE('',#33721,#4986);
#4043=LINE('',#33722,#4987);
#4044=LINE('',#33727,#4988);
#4045=LINE('',#33728,#4989);
#4046=LINE('',#33729,#4990);
#4047=LINE('',#33814,#4991);
#4048=LINE('',#33821,#4992);
#4049=LINE('',#33830,#4993);
#4050=LINE('',#33837,#4994);
#4051=LINE('',#33843,#4995);
#4052=LINE('',#33849,#4996);
#4053=LINE('',#33855,#4997);
#4054=LINE('',#33859,#4998);
#4055=LINE('',#33861,#4999);
#4056=LINE('',#33862,#5000);
#4057=LINE('',#33866,#5001);
#4058=LINE('',#33870,#5002);
#4059=LINE('',#33874,#5003);
#4060=LINE('',#33876,#5004);
#4061=LINE('',#33877,#5005);
#4062=LINE('',#33879,#5006);
#4063=LINE('',#33880,#5007);
#4064=LINE('',#33884,#5008);
#4065=LINE('',#33886,#5009);
#4066=LINE('',#33888,#5010);
#4067=LINE('',#33891,#5011);
#4068=LINE('',#33893,#5012);
#4069=LINE('',#33894,#5013);
#4070=LINE('',#33898,#5014);
#4071=LINE('',#33899,#5015);
#4072=LINE('',#33901,#5016);
#4073=LINE('',#33902,#5017);
#4074=LINE('',#33905,#5018);
#4075=LINE('',#33909,#5019);
#4076=LINE('',#33910,#5020);
#4077=LINE('',#33913,#5021);
#4078=LINE('',#33915,#5022);
#4079=LINE('',#33916,#5023);
#4080=LINE('',#33918,#5024);
#4081=LINE('',#33920,#5025);
#4082=LINE('',#33929,#5026);
#4083=LINE('',#33948,#5027);
#4084=LINE('',#33956,#5028);
#4085=LINE('',#33961,#5029);
#4086=LINE('',#33967,#5030);
#4087=LINE('',#33974,#5031);
#4088=LINE('',#33979,#5032);
#4089=LINE('',#33985,#5033);
#4090=LINE('',#33992,#5034);
#4091=LINE('',#33997,#5035);
#4092=LINE('',#34003,#5036);
#4093=LINE('',#34010,#5037);
#4094=LINE('',#34015,#5038);
#4095=LINE('',#34021,#5039);
#4096=LINE('',#34028,#5040);
#4097=LINE('',#34033,#5041);
#4098=LINE('',#34039,#5042);
#4099=LINE('',#34046,#5043);
#4100=LINE('',#34051,#5044);
#4101=LINE('',#34057,#5045);
#4102=LINE('',#34064,#5046);
#4103=LINE('',#34069,#5047);
#4104=LINE('',#34075,#5048);
#4105=LINE('',#34082,#5049);
#4106=LINE('',#34087,#5050);
#4107=LINE('',#34093,#5051);
#4108=LINE('',#34100,#5052);
#4109=LINE('',#34105,#5053);
#4110=LINE('',#34111,#5054);
#4111=LINE('',#34118,#5055);
#4112=LINE('',#34123,#5056);
#4113=LINE('',#34129,#5057);
#4114=LINE('',#34136,#5058);
#4115=LINE('',#34141,#5059);
#4116=LINE('',#34147,#5060);
#4117=LINE('',#34154,#5061);
#4118=LINE('',#34159,#5062);
#4119=LINE('',#34165,#5063);
#4120=LINE('',#34172,#5064);
#4121=LINE('',#34177,#5065);
#4122=LINE('',#34183,#5066);
#4123=LINE('',#34190,#5067);
#4124=LINE('',#34195,#5068);
#4125=LINE('',#34201,#5069);
#4126=LINE('',#34208,#5070);
#4127=LINE('',#34213,#5071);
#4128=LINE('',#34607,#5072);
#4129=LINE('',#35385,#5073);
#4130=LINE('',#35771,#5074);
#4131=LINE('',#35773,#5075);
#4132=LINE('',#35774,#5076);
#4133=LINE('',#35776,#5077);
#4134=LINE('',#35777,#5078);
#4135=LINE('',#35779,#5079);
#4136=LINE('',#35780,#5080);
#4137=LINE('',#35782,#5081);
#4138=LINE('',#35783,#5082);
#4139=LINE('',#35785,#5083);
#4140=LINE('',#35786,#5084);
#4141=LINE('',#35788,#5085);
#4142=LINE('',#35789,#5086);
#4143=LINE('',#35791,#5087);
#4144=LINE('',#35792,#5088);
#4145=LINE('',#35794,#5089);
#4146=LINE('',#35795,#5090);
#4147=LINE('',#35797,#5091);
#4148=LINE('',#35798,#5092);
#4149=LINE('',#35800,#5093);
#4150=LINE('',#35801,#5094);
#4151=LINE('',#35803,#5095);
#4152=LINE('',#35804,#5096);
#4153=LINE('',#35806,#5097);
#4154=LINE('',#35807,#5098);
#4155=LINE('',#35809,#5099);
#4156=LINE('',#35810,#5100);
#4157=LINE('',#35812,#5101);
#4158=LINE('',#35813,#5102);
#4159=LINE('',#35815,#5103);
#4160=LINE('',#35816,#5104);
#4161=LINE('',#35818,#5105);
#4162=LINE('',#35819,#5106);
#4163=LINE('',#35821,#5107);
#4164=LINE('',#35822,#5108);
#4165=LINE('',#35824,#5109);
#4166=LINE('',#35825,#5110);
#4167=LINE('',#35827,#5111);
#4168=LINE('',#35828,#5112);
#4169=LINE('',#35830,#5113);
#4170=LINE('',#35831,#5114);
#4171=LINE('',#35833,#5115);
#4172=LINE('',#35834,#5116);
#4173=LINE('',#35836,#5117);
#4174=LINE('',#35837,#5118);
#4175=LINE('',#35839,#5119);
#4176=LINE('',#35840,#5120);
#4177=LINE('',#35842,#5121);
#4178=LINE('',#35843,#5122);
#4179=LINE('',#35845,#5123);
#4180=LINE('',#35846,#5124);
#4181=LINE('',#35848,#5125);
#4182=LINE('',#35849,#5126);
#4183=LINE('',#35851,#5127);
#4184=LINE('',#35852,#5128);
#4185=LINE('',#35854,#5129);
#4186=LINE('',#35855,#5130);
#4187=LINE('',#35857,#5131);
#4188=LINE('',#35858,#5132);
#4189=LINE('',#35860,#5133);
#4190=LINE('',#35861,#5134);
#4191=LINE('',#35863,#5135);
#4192=LINE('',#35864,#5136);
#4193=LINE('',#35866,#5137);
#4194=LINE('',#35867,#5138);
#4195=LINE('',#35869,#5139);
#4196=LINE('',#35870,#5140);
#4197=LINE('',#35872,#5141);
#4198=LINE('',#35873,#5142);
#4199=LINE('',#35875,#5143);
#4200=LINE('',#35876,#5144);
#4201=LINE('',#35878,#5145);
#4202=LINE('',#35879,#5146);
#4203=LINE('',#35881,#5147);
#4204=LINE('',#35882,#5148);
#4205=LINE('',#35884,#5149);
#4206=LINE('',#35885,#5150);
#4207=LINE('',#35887,#5151);
#4208=LINE('',#35888,#5152);
#4209=LINE('',#35890,#5153);
#4210=LINE('',#35891,#5154);
#4211=LINE('',#35893,#5155);
#4212=LINE('',#35894,#5156);
#4213=LINE('',#35896,#5157);
#4214=LINE('',#35897,#5158);
#4215=LINE('',#35899,#5159);
#4216=LINE('',#35900,#5160);
#4217=LINE('',#35902,#5161);
#4218=LINE('',#35903,#5162);
#4219=LINE('',#35905,#5163);
#4220=LINE('',#35906,#5164);
#4221=LINE('',#35908,#5165);
#4222=LINE('',#35909,#5166);
#4223=LINE('',#35911,#5167);
#4224=LINE('',#35912,#5168);
#4225=LINE('',#35914,#5169);
#4226=LINE('',#35915,#5170);
#4227=LINE('',#35917,#5171);
#4228=LINE('',#35918,#5172);
#4229=LINE('',#35920,#5173);
#4230=LINE('',#35921,#5174);
#4231=LINE('',#35923,#5175);
#4232=LINE('',#35924,#5176);
#4233=LINE('',#35926,#5177);
#4234=LINE('',#35927,#5178);
#4235=LINE('',#35929,#5179);
#4236=LINE('',#35930,#5180);
#4237=LINE('',#35932,#5181);
#4238=LINE('',#35933,#5182);
#4239=LINE('',#35935,#5183);
#4240=LINE('',#35936,#5184);
#4241=LINE('',#35938,#5185);
#4242=LINE('',#35939,#5186);
#4243=LINE('',#35941,#5187);
#4244=LINE('',#35942,#5188);
#4245=LINE('',#35944,#5189);
#4246=LINE('',#35945,#5190);
#4247=LINE('',#35947,#5191);
#4248=LINE('',#35948,#5192);
#4249=LINE('',#35950,#5193);
#4250=LINE('',#35951,#5194);
#4251=LINE('',#35953,#5195);
#4252=LINE('',#35954,#5196);
#4253=LINE('',#35956,#5197);
#4254=LINE('',#35957,#5198);
#4255=LINE('',#35959,#5199);
#4256=LINE('',#35960,#5200);
#4257=LINE('',#35962,#5201);
#4258=LINE('',#35963,#5202);
#4259=LINE('',#35965,#5203);
#4260=LINE('',#35966,#5204);
#4261=LINE('',#35968,#5205);
#4262=LINE('',#35969,#5206);
#4263=LINE('',#35971,#5207);
#4264=LINE('',#35972,#5208);
#4265=LINE('',#35974,#5209);
#4266=LINE('',#35975,#5210);
#4267=LINE('',#35977,#5211);
#4268=LINE('',#35978,#5212);
#4269=LINE('',#35980,#5213);
#4270=LINE('',#35981,#5214);
#4271=LINE('',#35983,#5215);
#4272=LINE('',#35984,#5216);
#4273=LINE('',#35986,#5217);
#4274=LINE('',#35987,#5218);
#4275=LINE('',#35989,#5219);
#4276=LINE('',#35990,#5220);
#4277=LINE('',#35992,#5221);
#4278=LINE('',#35993,#5222);
#4279=LINE('',#35995,#5223);
#4280=LINE('',#35996,#5224);
#4281=LINE('',#35998,#5225);
#4282=LINE('',#35999,#5226);
#4283=LINE('',#36002,#5227);
#4284=LINE('',#36003,#5228);
#4285=LINE('',#36007,#5229);
#4286=LINE('',#36010,#5230);
#4287=LINE('',#36013,#5231);
#4288=LINE('',#36016,#5232);
#4289=LINE('',#36019,#5233);
#4290=LINE('',#36022,#5234);
#4291=LINE('',#36025,#5235);
#4292=LINE('',#36028,#5236);
#4293=LINE('',#36031,#5237);
#4294=LINE('',#36034,#5238);
#4295=LINE('',#36037,#5239);
#4296=LINE('',#36040,#5240);
#4297=LINE('',#36043,#5241);
#4298=LINE('',#36046,#5242);
#4299=LINE('',#36049,#5243);
#4300=LINE('',#36052,#5244);
#4301=LINE('',#36055,#5245);
#4302=LINE('',#36058,#5246);
#4303=LINE('',#36061,#5247);
#4304=LINE('',#36064,#5248);
#4305=LINE('',#36067,#5249);
#4306=LINE('',#36070,#5250);
#4307=LINE('',#36073,#5251);
#4308=LINE('',#36076,#5252);
#4309=LINE('',#36079,#5253);
#4310=LINE('',#36082,#5254);
#4311=LINE('',#36085,#5255);
#4312=LINE('',#36088,#5256);
#4313=LINE('',#36091,#5257);
#4314=LINE('',#36094,#5258);
#4315=LINE('',#36097,#5259);
#4316=LINE('',#36100,#5260);
#4317=LINE('',#36103,#5261);
#4318=LINE('',#36106,#5262);
#4319=LINE('',#36109,#5263);
#4320=LINE('',#36112,#5264);
#4321=LINE('',#36115,#5265);
#4322=LINE('',#36118,#5266);
#4323=LINE('',#36121,#5267);
#4324=LINE('',#36124,#5268);
#4325=LINE('',#36127,#5269);
#4326=LINE('',#36130,#5270);
#4327=LINE('',#36133,#5271);
#4328=LINE('',#36136,#5272);
#4329=LINE('',#36139,#5273);
#4330=LINE('',#36142,#5274);
#4331=LINE('',#36145,#5275);
#4332=LINE('',#36148,#5276);
#4333=LINE('',#36151,#5277);
#4334=LINE('',#36154,#5278);
#4335=LINE('',#36157,#5279);
#4336=LINE('',#36160,#5280);
#4337=LINE('',#36163,#5281);
#4338=LINE('',#36166,#5282);
#4339=LINE('',#36169,#5283);
#4340=LINE('',#36172,#5284);
#4341=LINE('',#36175,#5285);
#4342=LINE('',#36178,#5286);
#4343=LINE('',#36181,#5287);
#4344=LINE('',#36184,#5288);
#4345=LINE('',#36187,#5289);
#4346=LINE('',#36190,#5290);
#4347=LINE('',#36193,#5291);
#4348=LINE('',#36196,#5292);
#4349=LINE('',#36199,#5293);
#4350=LINE('',#36202,#5294);
#4351=LINE('',#36205,#5295);
#4352=LINE('',#36208,#5296);
#4353=LINE('',#36211,#5297);
#4354=LINE('',#36214,#5298);
#4355=LINE('',#36217,#5299);
#4356=LINE('',#36220,#5300);
#4357=LINE('',#36223,#5301);
#4358=LINE('',#36226,#5302);
#4359=LINE('',#36229,#5303);
#4360=LINE('',#36232,#5304);
#4361=LINE('',#36235,#5305);
#4362=LINE('',#36300,#5306);
#4363=LINE('',#36305,#5307);
#4364=LINE('',#36308,#5308);
#4365=LINE('',#36311,#5309);
#4366=LINE('',#36314,#5310);
#4367=LINE('',#36316,#5311);
#4368=LINE('',#36330,#5312);
#4369=LINE('',#36338,#5313);
#4370=LINE('',#36343,#5314);
#4371=LINE('',#36349,#5315);
#4372=LINE('',#36356,#5316);
#4373=LINE('',#36361,#5317);
#4374=LINE('',#36367,#5318);
#4375=LINE('',#36374,#5319);
#4376=LINE('',#36379,#5320);
#4377=LINE('',#36385,#5321);
#4378=LINE('',#36392,#5322);
#4379=LINE('',#36397,#5323);
#4380=LINE('',#36403,#5324);
#4381=LINE('',#36410,#5325);
#4382=LINE('',#36415,#5326);
#4383=LINE('',#36421,#5327);
#4384=LINE('',#36428,#5328);
#4385=LINE('',#36433,#5329);
#4386=LINE('',#36439,#5330);
#4387=LINE('',#36446,#5331);
#4388=LINE('',#36451,#5332);
#4389=LINE('',#36457,#5333);
#4390=LINE('',#36464,#5334);
#4391=LINE('',#36469,#5335);
#4392=LINE('',#36475,#5336);
#4393=LINE('',#36482,#5337);
#4394=LINE('',#36487,#5338);
#4395=LINE('',#36493,#5339);
#4396=LINE('',#36500,#5340);
#4397=LINE('',#36505,#5341);
#4398=LINE('',#36511,#5342);
#4399=LINE('',#36518,#5343);
#4400=LINE('',#36523,#5344);
#4401=LINE('',#36529,#5345);
#4402=LINE('',#36536,#5346);
#4403=LINE('',#36541,#5347);
#4404=LINE('',#36547,#5348);
#4405=LINE('',#36554,#5349);
#4406=LINE('',#36559,#5350);
#4407=LINE('',#36562,#5351);
#4408=LINE('',#36957,#5352);
#4409=LINE('',#37735,#5353);
#4410=LINE('',#38123,#5354);
#4411=LINE('',#38125,#5355);
#4412=LINE('',#38126,#5356);
#4413=LINE('',#38128,#5357);
#4414=LINE('',#38129,#5358);
#4415=LINE('',#38131,#5359);
#4416=LINE('',#38132,#5360);
#4417=LINE('',#38134,#5361);
#4418=LINE('',#38135,#5362);
#4419=LINE('',#38137,#5363);
#4420=LINE('',#38138,#5364);
#4421=LINE('',#38140,#5365);
#4422=LINE('',#38141,#5366);
#4423=LINE('',#38143,#5367);
#4424=LINE('',#38144,#5368);
#4425=LINE('',#38146,#5369);
#4426=LINE('',#38147,#5370);
#4427=LINE('',#38149,#5371);
#4428=LINE('',#38150,#5372);
#4429=LINE('',#38152,#5373);
#4430=LINE('',#38153,#5374);
#4431=LINE('',#38155,#5375);
#4432=LINE('',#38156,#5376);
#4433=LINE('',#38158,#5377);
#4434=LINE('',#38159,#5378);
#4435=LINE('',#38161,#5379);
#4436=LINE('',#38162,#5380);
#4437=LINE('',#38164,#5381);
#4438=LINE('',#38165,#5382);
#4439=LINE('',#38167,#5383);
#4440=LINE('',#38168,#5384);
#4441=LINE('',#38170,#5385);
#4442=LINE('',#38171,#5386);
#4443=LINE('',#38173,#5387);
#4444=LINE('',#38174,#5388);
#4445=LINE('',#38176,#5389);
#4446=LINE('',#38177,#5390);
#4447=LINE('',#38179,#5391);
#4448=LINE('',#38180,#5392);
#4449=LINE('',#38182,#5393);
#4450=LINE('',#38183,#5394);
#4451=LINE('',#38185,#5395);
#4452=LINE('',#38186,#5396);
#4453=LINE('',#38188,#5397);
#4454=LINE('',#38189,#5398);
#4455=LINE('',#38191,#5399);
#4456=LINE('',#38192,#5400);
#4457=LINE('',#38194,#5401);
#4458=LINE('',#38195,#5402);
#4459=LINE('',#38197,#5403);
#4460=LINE('',#38198,#5404);
#4461=LINE('',#38200,#5405);
#4462=LINE('',#38201,#5406);
#4463=LINE('',#38203,#5407);
#4464=LINE('',#38204,#5408);
#4465=LINE('',#38206,#5409);
#4466=LINE('',#38207,#5410);
#4467=LINE('',#38209,#5411);
#4468=LINE('',#38210,#5412);
#4469=LINE('',#38212,#5413);
#4470=LINE('',#38213,#5414);
#4471=LINE('',#38215,#5415);
#4472=LINE('',#38216,#5416);
#4473=LINE('',#38218,#5417);
#4474=LINE('',#38219,#5418);
#4475=LINE('',#38221,#5419);
#4476=LINE('',#38222,#5420);
#4477=LINE('',#38224,#5421);
#4478=LINE('',#38225,#5422);
#4479=LINE('',#38227,#5423);
#4480=LINE('',#38228,#5424);
#4481=LINE('',#38230,#5425);
#4482=LINE('',#38231,#5426);
#4483=LINE('',#38233,#5427);
#4484=LINE('',#38234,#5428);
#4485=LINE('',#38236,#5429);
#4486=LINE('',#38237,#5430);
#4487=LINE('',#38239,#5431);
#4488=LINE('',#38240,#5432);
#4489=LINE('',#38242,#5433);
#4490=LINE('',#38243,#5434);
#4491=LINE('',#38245,#5435);
#4492=LINE('',#38246,#5436);
#4493=LINE('',#38248,#5437);
#4494=LINE('',#38249,#5438);
#4495=LINE('',#38251,#5439);
#4496=LINE('',#38252,#5440);
#4497=LINE('',#38254,#5441);
#4498=LINE('',#38255,#5442);
#4499=LINE('',#38257,#5443);
#4500=LINE('',#38258,#5444);
#4501=LINE('',#38260,#5445);
#4502=LINE('',#38261,#5446);
#4503=LINE('',#38263,#5447);
#4504=LINE('',#38264,#5448);
#4505=LINE('',#38266,#5449);
#4506=LINE('',#38267,#5450);
#4507=LINE('',#38269,#5451);
#4508=LINE('',#38270,#5452);
#4509=LINE('',#38272,#5453);
#4510=LINE('',#38273,#5454);
#4511=LINE('',#38275,#5455);
#4512=LINE('',#38276,#5456);
#4513=LINE('',#38278,#5457);
#4514=LINE('',#38279,#5458);
#4515=LINE('',#38281,#5459);
#4516=LINE('',#38282,#5460);
#4517=LINE('',#38284,#5461);
#4518=LINE('',#38285,#5462);
#4519=LINE('',#38287,#5463);
#4520=LINE('',#38288,#5464);
#4521=LINE('',#38290,#5465);
#4522=LINE('',#38291,#5466);
#4523=LINE('',#38293,#5467);
#4524=LINE('',#38294,#5468);
#4525=LINE('',#38296,#5469);
#4526=LINE('',#38297,#5470);
#4527=LINE('',#38299,#5471);
#4528=LINE('',#38300,#5472);
#4529=LINE('',#38302,#5473);
#4530=LINE('',#38303,#5474);
#4531=LINE('',#38305,#5475);
#4532=LINE('',#38306,#5476);
#4533=LINE('',#38308,#5477);
#4534=LINE('',#38309,#5478);
#4535=LINE('',#38311,#5479);
#4536=LINE('',#38312,#5480);
#4537=LINE('',#38314,#5481);
#4538=LINE('',#38315,#5482);
#4539=LINE('',#38317,#5483);
#4540=LINE('',#38318,#5484);
#4541=LINE('',#38320,#5485);
#4542=LINE('',#38321,#5486);
#4543=LINE('',#38323,#5487);
#4544=LINE('',#38324,#5488);
#4545=LINE('',#38326,#5489);
#4546=LINE('',#38327,#5490);
#4547=LINE('',#38329,#5491);
#4548=LINE('',#38330,#5492);
#4549=LINE('',#38332,#5493);
#4550=LINE('',#38333,#5494);
#4551=LINE('',#38335,#5495);
#4552=LINE('',#38336,#5496);
#4553=LINE('',#38338,#5497);
#4554=LINE('',#38339,#5498);
#4555=LINE('',#38341,#5499);
#4556=LINE('',#38342,#5500);
#4557=LINE('',#38344,#5501);
#4558=LINE('',#38345,#5502);
#4559=LINE('',#38347,#5503);
#4560=LINE('',#38348,#5504);
#4561=LINE('',#38350,#5505);
#4562=LINE('',#38351,#5506);
#4563=LINE('',#38354,#5507);
#4564=LINE('',#38355,#5508);
#4565=LINE('',#38360,#5509);
#4566=LINE('',#38363,#5510);
#4567=LINE('',#38366,#5511);
#4568=LINE('',#38369,#5512);
#4569=LINE('',#38372,#5513);
#4570=LINE('',#38375,#5514);
#4571=LINE('',#38378,#5515);
#4572=LINE('',#38381,#5516);
#4573=LINE('',#38384,#5517);
#4574=LINE('',#38387,#5518);
#4575=LINE('',#38390,#5519);
#4576=LINE('',#38393,#5520);
#4577=LINE('',#38396,#5521);
#4578=LINE('',#38399,#5522);
#4579=LINE('',#38402,#5523);
#4580=LINE('',#38405,#5524);
#4581=LINE('',#38408,#5525);
#4582=LINE('',#38411,#5526);
#4583=LINE('',#38414,#5527);
#4584=LINE('',#38417,#5528);
#4585=LINE('',#38420,#5529);
#4586=LINE('',#38423,#5530);
#4587=LINE('',#38426,#5531);
#4588=LINE('',#38429,#5532);
#4589=LINE('',#38432,#5533);
#4590=LINE('',#38435,#5534);
#4591=LINE('',#38438,#5535);
#4592=LINE('',#38441,#5536);
#4593=LINE('',#38444,#5537);
#4594=LINE('',#38447,#5538);
#4595=LINE('',#38450,#5539);
#4596=LINE('',#38453,#5540);
#4597=LINE('',#38456,#5541);
#4598=LINE('',#38459,#5542);
#4599=LINE('',#38462,#5543);
#4600=LINE('',#38465,#5544);
#4601=LINE('',#38468,#5545);
#4602=LINE('',#38471,#5546);
#4603=LINE('',#38474,#5547);
#4604=LINE('',#38477,#5548);
#4605=LINE('',#38480,#5549);
#4606=LINE('',#38483,#5550);
#4607=LINE('',#38486,#5551);
#4608=LINE('',#38489,#5552);
#4609=LINE('',#38492,#5553);
#4610=LINE('',#38495,#5554);
#4611=LINE('',#38498,#5555);
#4612=LINE('',#38501,#5556);
#4613=LINE('',#38504,#5557);
#4614=LINE('',#38507,#5558);
#4615=LINE('',#38510,#5559);
#4616=LINE('',#38513,#5560);
#4617=LINE('',#38516,#5561);
#4618=LINE('',#38519,#5562);
#4619=LINE('',#38522,#5563);
#4620=LINE('',#38525,#5564);
#4621=LINE('',#38528,#5565);
#4622=LINE('',#38531,#5566);
#4623=LINE('',#38534,#5567);
#4624=LINE('',#38537,#5568);
#4625=LINE('',#38540,#5569);
#4626=LINE('',#38543,#5570);
#4627=LINE('',#38546,#5571);
#4628=LINE('',#38549,#5572);
#4629=LINE('',#38552,#5573);
#4630=LINE('',#38555,#5574);
#4631=LINE('',#38558,#5575);
#4632=LINE('',#38561,#5576);
#4633=LINE('',#38564,#5577);
#4634=LINE('',#38567,#5578);
#4635=LINE('',#38570,#5579);
#4636=LINE('',#38573,#5580);
#4637=LINE('',#38576,#5581);
#4638=LINE('',#38579,#5582);
#4639=LINE('',#38582,#5583);
#4640=LINE('',#38585,#5584);
#4641=LINE('',#38588,#5585);
#4888=VECTOR('',#21315,2.);
#4889=VECTOR('',#21324,1.80000000000002);
#4890=VECTOR('',#21333,2.3);
#4891=VECTOR('',#21340,1.2);
#4892=VECTOR('',#21355,1.50000000000001);
#4893=VECTOR('',#21364,2.3);
#4894=VECTOR('',#21371,2.);
#4895=VECTOR('',#21378,1.5);
#4896=VECTOR('',#21389,2.);
#4897=VECTOR('',#21398,2.);
#4898=VECTOR('',#21401,1.2);
#4899=VECTOR('',#21404,1000.);
#4900=VECTOR('',#21405,1000.);
#4901=VECTOR('',#21406,1000.);
#4902=VECTOR('',#21409,2.);
#4903=VECTOR('',#21412,1.5);
#4904=VECTOR('',#21415,1000.);
#4905=VECTOR('',#21416,1000.);
#4906=VECTOR('',#21417,1000.);
#4907=VECTOR('',#21418,1000.);
#4908=VECTOR('',#21421,1000.);
#4909=VECTOR('',#21422,1000.);
#4910=VECTOR('',#21423,1000.);
#4911=VECTOR('',#21424,1000.);
#4912=VECTOR('',#21427,1000.);
#4913=VECTOR('',#21430,1000.);
#4914=VECTOR('',#21431,1000.);
#4915=VECTOR('',#21432,1000.);
#4916=VECTOR('',#21433,1000.);
#4917=VECTOR('',#21434,1000.);
#4918=VECTOR('',#21435,1000.);
#4919=VECTOR('',#21436,1000.);
#4920=VECTOR('',#21437,1000.);
#4921=VECTOR('',#21438,1000.);
#4922=VECTOR('',#21439,1000.);
#4923=VECTOR('',#21442,1000.);
#4924=VECTOR('',#21445,1000.);
#4925=VECTOR('',#21446,1000.);
#4926=VECTOR('',#21447,1000.);
#4927=VECTOR('',#21450,1000.);
#4928=VECTOR('',#21451,1000.);
#4929=VECTOR('',#21454,1000.);
#4930=VECTOR('',#21455,1000.);
#4931=VECTOR('',#21456,1000.);
#4932=VECTOR('',#21457,1000.);
#4933=VECTOR('',#21458,1000.);
#4934=VECTOR('',#21459,1000.);
#4935=VECTOR('',#21460,1000.);
#4936=VECTOR('',#21461,1000.);
#4937=VECTOR('',#21462,1000.);
#4938=VECTOR('',#21463,1000.);
#4939=VECTOR('',#21464,1000.);
#4940=VECTOR('',#21465,1000.);
#4941=VECTOR('',#21466,1000.);
#4942=VECTOR('',#21471,1000.);
#4943=VECTOR('',#21472,1000.);
#4944=VECTOR('',#21473,1000.);
#4945=VECTOR('',#21474,1000.);
#4946=VECTOR('',#21477,1000.);
#4947=VECTOR('',#21478,1000.);
#4948=VECTOR('',#21479,1000.);
#4949=VECTOR('',#21480,1000.);
#4950=VECTOR('',#21481,1000.);
#4951=VECTOR('',#21482,1000.);
#4952=VECTOR('',#21483,1000.);
#4953=VECTOR('',#21486,1000.);
#4954=VECTOR('',#21487,1000.);
#4955=VECTOR('',#21488,1000.);
#4956=VECTOR('',#21489,1000.);
#4957=VECTOR('',#21492,1000.);
#4958=VECTOR('',#21493,1000.);
#4959=VECTOR('',#21496,1000.);
#4960=VECTOR('',#21497,1000.);
#4961=VECTOR('',#21498,1000.);
#4962=VECTOR('',#21499,1000.);
#4963=VECTOR('',#21502,1000.);
#4964=VECTOR('',#21503,1000.);
#4965=VECTOR('',#21504,1000.);
#4966=VECTOR('',#21505,1000.);
#4967=VECTOR('',#21508,1000.);
#4968=VECTOR('',#21511,1000.);
#4969=VECTOR('',#21518,1000.);
#4970=VECTOR('',#21521,1000.);
#4971=VECTOR('',#21528,1000.);
#4972=VECTOR('',#21531,1000.);
#4973=VECTOR('',#21536,1000.);
#4974=VECTOR('',#21539,1000.);
#4975=VECTOR('',#21544,1000.);
#4976=VECTOR('',#21545,1000.);
#4977=VECTOR('',#21548,1000.);
#4978=VECTOR('',#21549,1000.);
#4979=VECTOR('',#21552,1000.);
#4980=VECTOR('',#21553,1000.);
#4981=VECTOR('',#21556,1000.);
#4982=VECTOR('',#21557,1000.);
#4983=VECTOR('',#21558,1000.);
#4984=VECTOR('',#21561,1000.);
#4985=VECTOR('',#21562,1000.);
#4986=VECTOR('',#21569,1000.);
#4987=VECTOR('',#21570,1000.);
#4988=VECTOR('',#21575,1000.);
#4989=VECTOR('',#21576,1000.);
#4990=VECTOR('',#21577,1000.);
#4991=VECTOR('',#21734,1.2);
#4992=VECTOR('',#21743,2.5);
#4993=VECTOR('',#21752,3.);
#4994=VECTOR('',#21761,4.25);
#4995=VECTOR('',#21768,1.2);
#4996=VECTOR('',#21775,1.2);
#4997=VECTOR('',#21782,2.);
#4998=VECTOR('',#21787,1000.);
#4999=VECTOR('',#21788,1000.);
#5000=VECTOR('',#21789,1000.);
#5001=VECTOR('',#21792,1000.);
#5002=VECTOR('',#21795,1000.);
#5003=VECTOR('',#21800,1000.);
#5004=VECTOR('',#21801,1000.);
#5005=VECTOR('',#21802,1000.);
#5006=VECTOR('',#21805,1000.);
#5007=VECTOR('',#21806,1000.);
#5008=VECTOR('',#21809,1000.);
#5009=VECTOR('',#21810,1000.);
#5010=VECTOR('',#21811,1000.);
#5011=VECTOR('',#21814,1000.);
#5012=VECTOR('',#21817,1000.);
#5013=VECTOR('',#21818,1000.);
#5014=VECTOR('',#21821,1000.);
#5015=VECTOR('',#21822,1000.);
#5016=VECTOR('',#21823,1000.);
#5017=VECTOR('',#21824,1000.);
#5018=VECTOR('',#21827,1000.);
#5019=VECTOR('',#21832,1000.);
#5020=VECTOR('',#21833,1000.);
#5021=VECTOR('',#21836,1000.);
#5022=VECTOR('',#21837,1000.);
#5023=VECTOR('',#21838,1000.);
#5024=VECTOR('',#21841,1000.);
#5025=VECTOR('',#21844,1000.);
#5026=VECTOR('',#21857,2.5);
#5027=VECTOR('',#21880,2.);
#5028=VECTOR('',#21889,1.61);
#5029=VECTOR('',#21896,2.);
#5030=VECTOR('',#21903,2.);
#5031=VECTOR('',#21910,1.61);
#5032=VECTOR('',#21917,2.);
#5033=VECTOR('',#21924,2.);
#5034=VECTOR('',#21931,1.61);
#5035=VECTOR('',#21938,2.);
#5036=VECTOR('',#21945,2.);
#5037=VECTOR('',#21952,1.61);
#5038=VECTOR('',#21959,2.);
#5039=VECTOR('',#21966,2.);
#5040=VECTOR('',#21973,1.61);
#5041=VECTOR('',#21980,2.);
#5042=VECTOR('',#21987,2.);
#5043=VECTOR('',#21994,1.61);
#5044=VECTOR('',#22001,2.);
#5045=VECTOR('',#22008,2.);
#5046=VECTOR('',#22015,1.61);
#5047=VECTOR('',#22022,2.);
#5048=VECTOR('',#22029,2.);
#5049=VECTOR('',#22036,1.61);
#5050=VECTOR('',#22043,2.);
#5051=VECTOR('',#22050,2.);
#5052=VECTOR('',#22057,1.61);
#5053=VECTOR('',#22064,2.);
#5054=VECTOR('',#22071,2.);
#5055=VECTOR('',#22078,1.61);
#5056=VECTOR('',#22085,2.);
#5057=VECTOR('',#22092,2.);
#5058=VECTOR('',#22099,1.61);
#5059=VECTOR('',#22106,2.);
#5060=VECTOR('',#22113,2.);
#5061=VECTOR('',#22120,1.61);
#5062=VECTOR('',#22127,2.);
#5063=VECTOR('',#22134,2.);
#5064=VECTOR('',#22141,1.61);
#5065=VECTOR('',#22148,2.);
#5066=VECTOR('',#22155,2.);
#5067=VECTOR('',#22162,1.61);
#5068=VECTOR('',#22169,2.);
#5069=VECTOR('',#22176,2.);
#5070=VECTOR('',#22183,1.61);
#5071=VECTOR('',#22190,2.);
#5072=VECTOR('',#22271,8.175);
#5073=VECTOR('',#22430,8.175);
#5074=VECTOR('',#22511,2.);
#5075=VECTOR('',#22514,1000.);
#5076=VECTOR('',#22515,1000.);
#5077=VECTOR('',#22518,1000.);
#5078=VECTOR('',#22519,1000.);
#5079=VECTOR('',#22522,1000.);
#5080=VECTOR('',#22523,1000.);
#5081=VECTOR('',#22526,1000.);
#5082=VECTOR('',#22527,1000.);
#5083=VECTOR('',#22530,1000.);
#5084=VECTOR('',#22531,1000.);
#5085=VECTOR('',#22534,1000.);
#5086=VECTOR('',#22535,1000.);
#5087=VECTOR('',#22538,1000.);
#5088=VECTOR('',#22539,1000.);
#5089=VECTOR('',#22542,1000.);
#5090=VECTOR('',#22543,1000.);
#5091=VECTOR('',#22546,1000.);
#5092=VECTOR('',#22547,1000.);
#5093=VECTOR('',#22550,1000.);
#5094=VECTOR('',#22551,1000.);
#5095=VECTOR('',#22554,1000.);
#5096=VECTOR('',#22555,1000.);
#5097=VECTOR('',#22558,1000.);
#5098=VECTOR('',#22559,1000.);
#5099=VECTOR('',#22562,1000.);
#5100=VECTOR('',#22563,1000.);
#5101=VECTOR('',#22566,1000.);
#5102=VECTOR('',#22567,1000.);
#5103=VECTOR('',#22570,1000.);
#5104=VECTOR('',#22571,1000.);
#5105=VECTOR('',#22574,1000.);
#5106=VECTOR('',#22575,1000.);
#5107=VECTOR('',#22578,1000.);
#5108=VECTOR('',#22579,1000.);
#5109=VECTOR('',#22582,1000.);
#5110=VECTOR('',#22583,1000.);
#5111=VECTOR('',#22586,1000.);
#5112=VECTOR('',#22587,1000.);
#5113=VECTOR('',#22590,1000.);
#5114=VECTOR('',#22591,1000.);
#5115=VECTOR('',#22594,1000.);
#5116=VECTOR('',#22595,1000.);
#5117=VECTOR('',#22598,1000.);
#5118=VECTOR('',#22599,1000.);
#5119=VECTOR('',#22602,1000.);
#5120=VECTOR('',#22603,1000.);
#5121=VECTOR('',#22606,1000.);
#5122=VECTOR('',#22607,1000.);
#5123=VECTOR('',#22610,1000.);
#5124=VECTOR('',#22611,1000.);
#5125=VECTOR('',#22614,1000.);
#5126=VECTOR('',#22615,1000.);
#5127=VECTOR('',#22618,1000.);
#5128=VECTOR('',#22619,1000.);
#5129=VECTOR('',#22622,1000.);
#5130=VECTOR('',#22623,1000.);
#5131=VECTOR('',#22626,1000.);
#5132=VECTOR('',#22627,1000.);
#5133=VECTOR('',#22630,1000.);
#5134=VECTOR('',#22631,1000.);
#5135=VECTOR('',#22634,1000.);
#5136=VECTOR('',#22635,1000.);
#5137=VECTOR('',#22638,1000.);
#5138=VECTOR('',#22639,1000.);
#5139=VECTOR('',#22642,1000.);
#5140=VECTOR('',#22643,1000.);
#5141=VECTOR('',#22646,1000.);
#5142=VECTOR('',#22647,1000.);
#5143=VECTOR('',#22650,1000.);
#5144=VECTOR('',#22651,1000.);
#5145=VECTOR('',#22654,1000.);
#5146=VECTOR('',#22655,1000.);
#5147=VECTOR('',#22658,1000.);
#5148=VECTOR('',#22659,1000.);
#5149=VECTOR('',#22662,1000.);
#5150=VECTOR('',#22663,1000.);
#5151=VECTOR('',#22666,1000.);
#5152=VECTOR('',#22667,1000.);
#5153=VECTOR('',#22670,1000.);
#5154=VECTOR('',#22671,1000.);
#5155=VECTOR('',#22674,1000.);
#5156=VECTOR('',#22675,1000.);
#5157=VECTOR('',#22678,1000.);
#5158=VECTOR('',#22679,1000.);
#5159=VECTOR('',#22682,1000.);
#5160=VECTOR('',#22683,1000.);
#5161=VECTOR('',#22686,1000.);
#5162=VECTOR('',#22687,1000.);
#5163=VECTOR('',#22690,1000.);
#5164=VECTOR('',#22691,1000.);
#5165=VECTOR('',#22694,1000.);
#5166=VECTOR('',#22695,1000.);
#5167=VECTOR('',#22698,1000.);
#5168=VECTOR('',#22699,1000.);
#5169=VECTOR('',#22702,1000.);
#5170=VECTOR('',#22703,1000.);
#5171=VECTOR('',#22706,1000.);
#5172=VECTOR('',#22707,1000.);
#5173=VECTOR('',#22710,1000.);
#5174=VECTOR('',#22711,1000.);
#5175=VECTOR('',#22714,1000.);
#5176=VECTOR('',#22715,1000.);
#5177=VECTOR('',#22718,1000.);
#5178=VECTOR('',#22719,1000.);
#5179=VECTOR('',#22722,1000.);
#5180=VECTOR('',#22723,1000.);
#5181=VECTOR('',#22726,1000.);
#5182=VECTOR('',#22727,1000.);
#5183=VECTOR('',#22730,1000.);
#5184=VECTOR('',#22731,1000.);
#5185=VECTOR('',#22734,1000.);
#5186=VECTOR('',#22735,1000.);
#5187=VECTOR('',#22738,1000.);
#5188=VECTOR('',#22739,1000.);
#5189=VECTOR('',#22742,1000.);
#5190=VECTOR('',#22743,1000.);
#5191=VECTOR('',#22746,1000.);
#5192=VECTOR('',#22747,1000.);
#5193=VECTOR('',#22750,1000.);
#5194=VECTOR('',#22751,1000.);
#5195=VECTOR('',#22754,1000.);
#5196=VECTOR('',#22755,1000.);
#5197=VECTOR('',#22758,1000.);
#5198=VECTOR('',#22759,1000.);
#5199=VECTOR('',#22762,1000.);
#5200=VECTOR('',#22763,1000.);
#5201=VECTOR('',#22766,1000.);
#5202=VECTOR('',#22767,1000.);
#5203=VECTOR('',#22770,1000.);
#5204=VECTOR('',#22771,1000.);
#5205=VECTOR('',#22774,1000.);
#5206=VECTOR('',#22775,1000.);
#5207=VECTOR('',#22778,1000.);
#5208=VECTOR('',#22779,1000.);
#5209=VECTOR('',#22782,1000.);
#5210=VECTOR('',#22783,1000.);
#5211=VECTOR('',#22786,1000.);
#5212=VECTOR('',#22787,1000.);
#5213=VECTOR('',#22790,1000.);
#5214=VECTOR('',#22791,1000.);
#5215=VECTOR('',#22794,1000.);
#5216=VECTOR('',#22795,1000.);
#5217=VECTOR('',#22798,1000.);
#5218=VECTOR('',#22799,1000.);
#5219=VECTOR('',#22802,1000.);
#5220=VECTOR('',#22803,1000.);
#5221=VECTOR('',#22806,1000.);
#5222=VECTOR('',#22807,1000.);
#5223=VECTOR('',#22810,1000.);
#5224=VECTOR('',#22811,1000.);
#5225=VECTOR('',#22814,1000.);
#5226=VECTOR('',#22815,1000.);
#5227=VECTOR('',#22820,1000.);
#5228=VECTOR('',#22821,1000.);
#5229=VECTOR('',#22828,1000.);
#5230=VECTOR('',#22833,1000.);
#5231=VECTOR('',#22838,1000.);
#5232=VECTOR('',#22843,1000.);
#5233=VECTOR('',#22848,1000.);
#5234=VECTOR('',#22853,1000.);
#5235=VECTOR('',#22858,1000.);
#5236=VECTOR('',#22863,1000.);
#5237=VECTOR('',#22868,1000.);
#5238=VECTOR('',#22873,1000.);
#5239=VECTOR('',#22878,1000.);
#5240=VECTOR('',#22883,1000.);
#5241=VECTOR('',#22888,1000.);
#5242=VECTOR('',#22893,1000.);
#5243=VECTOR('',#22898,1000.);
#5244=VECTOR('',#22903,1000.);
#5245=VECTOR('',#22908,1000.);
#5246=VECTOR('',#22913,1000.);
#5247=VECTOR('',#22918,1000.);
#5248=VECTOR('',#22923,1000.);
#5249=VECTOR('',#22928,1000.);
#5250=VECTOR('',#22933,1000.);
#5251=VECTOR('',#22938,1000.);
#5252=VECTOR('',#22943,1000.);
#5253=VECTOR('',#22948,1000.);
#5254=VECTOR('',#22953,1000.);
#5255=VECTOR('',#22958,1000.);
#5256=VECTOR('',#22963,1000.);
#5257=VECTOR('',#22968,1000.);
#5258=VECTOR('',#22973,1000.);
#5259=VECTOR('',#22978,1000.);
#5260=VECTOR('',#22983,1000.);
#5261=VECTOR('',#22988,1000.);
#5262=VECTOR('',#22993,1000.);
#5263=VECTOR('',#22998,1000.);
#5264=VECTOR('',#23003,1000.);
#5265=VECTOR('',#23008,1000.);
#5266=VECTOR('',#23013,1000.);
#5267=VECTOR('',#23018,1000.);
#5268=VECTOR('',#23023,1000.);
#5269=VECTOR('',#23028,1000.);
#5270=VECTOR('',#23033,1000.);
#5271=VECTOR('',#23038,1000.);
#5272=VECTOR('',#23043,1000.);
#5273=VECTOR('',#23048,1000.);
#5274=VECTOR('',#23053,1000.);
#5275=VECTOR('',#23058,1000.);
#5276=VECTOR('',#23063,1000.);
#5277=VECTOR('',#23068,1000.);
#5278=VECTOR('',#23073,1000.);
#5279=VECTOR('',#23078,1000.);
#5280=VECTOR('',#23083,1000.);
#5281=VECTOR('',#23088,1000.);
#5282=VECTOR('',#23093,1000.);
#5283=VECTOR('',#23098,1000.);
#5284=VECTOR('',#23103,1000.);
#5285=VECTOR('',#23108,1000.);
#5286=VECTOR('',#23113,1000.);
#5287=VECTOR('',#23118,1000.);
#5288=VECTOR('',#23123,1000.);
#5289=VECTOR('',#23128,1000.);
#5290=VECTOR('',#23133,1000.);
#5291=VECTOR('',#23138,1000.);
#5292=VECTOR('',#23143,1000.);
#5293=VECTOR('',#23148,1000.);
#5294=VECTOR('',#23153,1000.);
#5295=VECTOR('',#23158,1000.);
#5296=VECTOR('',#23163,1000.);
#5297=VECTOR('',#23168,1000.);
#5298=VECTOR('',#23173,1000.);
#5299=VECTOR('',#23178,1000.);
#5300=VECTOR('',#23183,1000.);
#5301=VECTOR('',#23188,1000.);
#5302=VECTOR('',#23193,1000.);
#5303=VECTOR('',#23198,1000.);
#5304=VECTOR('',#23203,1000.);
#5305=VECTOR('',#23208,1000.);
#5306=VECTOR('',#23233,2.64252040565333);
#5307=VECTOR('',#23238,1.5);
#5308=VECTOR('',#23243,1000.);
#5309=VECTOR('',#23248,1000.);
#5310=VECTOR('',#23253,1000.);
#5311=VECTOR('',#23256,1000.);
#5312=VECTOR('',#23273,2.);
#5313=VECTOR('',#23282,1.61);
#5314=VECTOR('',#23289,2.);
#5315=VECTOR('',#23296,2.);
#5316=VECTOR('',#23303,1.61);
#5317=VECTOR('',#23310,2.);
#5318=VECTOR('',#23317,2.);
#5319=VECTOR('',#23324,1.61);
#5320=VECTOR('',#23331,2.);
#5321=VECTOR('',#23338,2.);
#5322=VECTOR('',#23345,1.61);
#5323=VECTOR('',#23352,2.);
#5324=VECTOR('',#23359,2.);
#5325=VECTOR('',#23366,1.61);
#5326=VECTOR('',#23373,2.);
#5327=VECTOR('',#23380,2.);
#5328=VECTOR('',#23387,1.61);
#5329=VECTOR('',#23394,2.);
#5330=VECTOR('',#23401,2.);
#5331=VECTOR('',#23408,1.61);
#5332=VECTOR('',#23415,2.);
#5333=VECTOR('',#23422,2.);
#5334=VECTOR('',#23429,1.61);
#5335=VECTOR('',#23436,2.);
#5336=VECTOR('',#23443,2.);
#5337=VECTOR('',#23450,1.61);
#5338=VECTOR('',#23457,2.);
#5339=VECTOR('',#23464,2.);
#5340=VECTOR('',#23471,1.61);
#5341=VECTOR('',#23478,2.);
#5342=VECTOR('',#23485,2.);
#5343=VECTOR('',#23492,1.61);
#5344=VECTOR('',#23499,2.);
#5345=VECTOR('',#23506,2.);
#5346=VECTOR('',#23513,1.61);
#5347=VECTOR('',#23520,2.);
#5348=VECTOR('',#23527,2.);
#5349=VECTOR('',#23534,1.61);
#5350=VECTOR('',#23541,2.);
#5351=VECTOR('',#23544,4.);
#5352=VECTOR('',#23627,8.175);
#5353=VECTOR('',#23786,8.175);
#5354=VECTOR('',#23869,2.);
#5355=VECTOR('',#23872,1000.);
#5356=VECTOR('',#23873,1000.);
#5357=VECTOR('',#23876,1000.);
#5358=VECTOR('',#23877,1000.);
#5359=VECTOR('',#23880,1000.);
#5360=VECTOR('',#23881,1000.);
#5361=VECTOR('',#23884,1000.);
#5362=VECTOR('',#23885,1000.);
#5363=VECTOR('',#23888,1000.);
#5364=VECTOR('',#23889,1000.);
#5365=VECTOR('',#23892,1000.);
#5366=VECTOR('',#23893,1000.);
#5367=VECTOR('',#23896,1000.);
#5368=VECTOR('',#23897,1000.);
#5369=VECTOR('',#23900,1000.);
#5370=VECTOR('',#23901,1000.);
#5371=VECTOR('',#23904,1000.);
#5372=VECTOR('',#23905,1000.);
#5373=VECTOR('',#23908,1000.);
#5374=VECTOR('',#23909,1000.);
#5375=VECTOR('',#23912,1000.);
#5376=VECTOR('',#23913,1000.);
#5377=VECTOR('',#23916,1000.);
#5378=VECTOR('',#23917,1000.);
#5379=VECTOR('',#23920,1000.);
#5380=VECTOR('',#23921,1000.);
#5381=VECTOR('',#23924,1000.);
#5382=VECTOR('',#23925,1000.);
#5383=VECTOR('',#23928,1000.);
#5384=VECTOR('',#23929,1000.);
#5385=VECTOR('',#23932,1000.);
#5386=VECTOR('',#23933,1000.);
#5387=VECTOR('',#23936,1000.);
#5388=VECTOR('',#23937,1000.);
#5389=VECTOR('',#23940,1000.);
#5390=VECTOR('',#23941,1000.);
#5391=VECTOR('',#23944,1000.);
#5392=VECTOR('',#23945,1000.);
#5393=VECTOR('',#23948,1000.);
#5394=VECTOR('',#23949,1000.);
#5395=VECTOR('',#23952,1000.);
#5396=VECTOR('',#23953,1000.);
#5397=VECTOR('',#23956,1000.);
#5398=VECTOR('',#23957,1000.);
#5399=VECTOR('',#23960,1000.);
#5400=VECTOR('',#23961,1000.);
#5401=VECTOR('',#23964,1000.);
#5402=VECTOR('',#23965,1000.);
#5403=VECTOR('',#23968,1000.);
#5404=VECTOR('',#23969,1000.);
#5405=VECTOR('',#23972,1000.);
#5406=VECTOR('',#23973,1000.);
#5407=VECTOR('',#23976,1000.);
#5408=VECTOR('',#23977,1000.);
#5409=VECTOR('',#23980,1000.);
#5410=VECTOR('',#23981,1000.);
#5411=VECTOR('',#23984,1000.);
#5412=VECTOR('',#23985,1000.);
#5413=VECTOR('',#23988,1000.);
#5414=VECTOR('',#23989,1000.);
#5415=VECTOR('',#23992,1000.);
#5416=VECTOR('',#23993,1000.);
#5417=VECTOR('',#23996,1000.);
#5418=VECTOR('',#23997,1000.);
#5419=VECTOR('',#24000,1000.);
#5420=VECTOR('',#24001,1000.);
#5421=VECTOR('',#24004,1000.);
#5422=VECTOR('',#24005,1000.);
#5423=VECTOR('',#24008,1000.);
#5424=VECTOR('',#24009,1000.);
#5425=VECTOR('',#24012,1000.);
#5426=VECTOR('',#24013,1000.);
#5427=VECTOR('',#24016,1000.);
#5428=VECTOR('',#24017,1000.);
#5429=VECTOR('',#24020,1000.);
#5430=VECTOR('',#24021,1000.);
#5431=VECTOR('',#24024,1000.);
#5432=VECTOR('',#24025,1000.);
#5433=VECTOR('',#24028,1000.);
#5434=VECTOR('',#24029,1000.);
#5435=VECTOR('',#24032,1000.);
#5436=VECTOR('',#24033,1000.);
#5437=VECTOR('',#24036,1000.);
#5438=VECTOR('',#24037,1000.);
#5439=VECTOR('',#24040,1000.);
#5440=VECTOR('',#24041,1000.);
#5441=VECTOR('',#24044,1000.);
#5442=VECTOR('',#24045,1000.);
#5443=VECTOR('',#24048,1000.);
#5444=VECTOR('',#24049,1000.);
#5445=VECTOR('',#24052,1000.);
#5446=VECTOR('',#24053,1000.);
#5447=VECTOR('',#24056,1000.);
#5448=VECTOR('',#24057,1000.);
#5449=VECTOR('',#24060,1000.);
#5450=VECTOR('',#24061,1000.);
#5451=VECTOR('',#24064,1000.);
#5452=VECTOR('',#24065,1000.);
#5453=VECTOR('',#24068,1000.);
#5454=VECTOR('',#24069,1000.);
#5455=VECTOR('',#24072,1000.);
#5456=VECTOR('',#24073,1000.);
#5457=VECTOR('',#24076,1000.);
#5458=VECTOR('',#24077,1000.);
#5459=VECTOR('',#24080,1000.);
#5460=VECTOR('',#24081,1000.);
#5461=VECTOR('',#24084,1000.);
#5462=VECTOR('',#24085,1000.);
#5463=VECTOR('',#24088,1000.);
#5464=VECTOR('',#24089,1000.);
#5465=VECTOR('',#24092,1000.);
#5466=VECTOR('',#24093,1000.);
#5467=VECTOR('',#24096,1000.);
#5468=VECTOR('',#24097,1000.);
#5469=VECTOR('',#24100,1000.);
#5470=VECTOR('',#24101,1000.);
#5471=VECTOR('',#24104,1000.);
#5472=VECTOR('',#24105,1000.);
#5473=VECTOR('',#24108,1000.);
#5474=VECTOR('',#24109,1000.);
#5475=VECTOR('',#24112,1000.);
#5476=VECTOR('',#24113,1000.);
#5477=VECTOR('',#24116,1000.);
#5478=VECTOR('',#24117,1000.);
#5479=VECTOR('',#24120,1000.);
#5480=VECTOR('',#24121,1000.);
#5481=VECTOR('',#24124,1000.);
#5482=VECTOR('',#24125,1000.);
#5483=VECTOR('',#24128,1000.);
#5484=VECTOR('',#24129,1000.);
#5485=VECTOR('',#24132,1000.);
#5486=VECTOR('',#24133,1000.);
#5487=VECTOR('',#24136,1000.);
#5488=VECTOR('',#24137,1000.);
#5489=VECTOR('',#24140,1000.);
#5490=VECTOR('',#24141,1000.);
#5491=VECTOR('',#24144,1000.);
#5492=VECTOR('',#24145,1000.);
#5493=VECTOR('',#24148,1000.);
#5494=VECTOR('',#24149,1000.);
#5495=VECTOR('',#24152,1000.);
#5496=VECTOR('',#24153,1000.);
#5497=VECTOR('',#24156,1000.);
#5498=VECTOR('',#24157,1000.);
#5499=VECTOR('',#24160,1000.);
#5500=VECTOR('',#24161,1000.);
#5501=VECTOR('',#24164,1000.);
#5502=VECTOR('',#24165,1000.);
#5503=VECTOR('',#24168,1000.);
#5504=VECTOR('',#24169,1000.);
#5505=VECTOR('',#24172,1000.);
#5506=VECTOR('',#24173,1000.);
#5507=VECTOR('',#24178,1000.);
#5508=VECTOR('',#24179,1000.);
#5509=VECTOR('',#24188,1000.);
#5510=VECTOR('',#24193,1000.);
#5511=VECTOR('',#24198,1000.);
#5512=VECTOR('',#24203,1000.);
#5513=VECTOR('',#24208,1000.);
#5514=VECTOR('',#24213,1000.);
#5515=VECTOR('',#24218,1000.);
#5516=VECTOR('',#24223,1000.);
#5517=VECTOR('',#24228,1000.);
#5518=VECTOR('',#24233,1000.);
#5519=VECTOR('',#24238,1000.);
#5520=VECTOR('',#24243,1000.);
#5521=VECTOR('',#24248,1000.);
#5522=VECTOR('',#24253,1000.);
#5523=VECTOR('',#24258,1000.);
#5524=VECTOR('',#24263,1000.);
#5525=VECTOR('',#24268,1000.);
#5526=VECTOR('',#24273,1000.);
#5527=VECTOR('',#24278,1000.);
#5528=VECTOR('',#24283,1000.);
#5529=VECTOR('',#24288,1000.);
#5530=VECTOR('',#24293,1000.);
#5531=VECTOR('',#24298,1000.);
#5532=VECTOR('',#24303,1000.);
#5533=VECTOR('',#24308,1000.);
#5534=VECTOR('',#24313,1000.);
#5535=VECTOR('',#24318,1000.);
#5536=VECTOR('',#24323,1000.);
#5537=VECTOR('',#24328,1000.);
#5538=VECTOR('',#24333,1000.);
#5539=VECTOR('',#24338,1000.);
#5540=VECTOR('',#24343,1000.);
#5541=VECTOR('',#24348,1000.);
#5542=VECTOR('',#24353,1000.);
#5543=VECTOR('',#24358,1000.);
#5544=VECTOR('',#24363,1000.);
#5545=VECTOR('',#24368,1000.);
#5546=VECTOR('',#24373,1000.);
#5547=VECTOR('',#24378,1000.);
#5548=VECTOR('',#24383,1000.);
#5549=VECTOR('',#24388,1000.);
#5550=VECTOR('',#24393,1000.);
#5551=VECTOR('',#24398,1000.);
#5552=VECTOR('',#24403,1000.);
#5553=VECTOR('',#24408,1000.);
#5554=VECTOR('',#24413,1000.);
#5555=VECTOR('',#24418,1000.);
#5556=VECTOR('',#24423,1000.);
#5557=VECTOR('',#24428,1000.);
#5558=VECTOR('',#24433,1000.);
#5559=VECTOR('',#24438,1000.);
#5560=VECTOR('',#24443,1000.);
#5561=VECTOR('',#24448,1000.);
#5562=VECTOR('',#24453,1000.);
#5563=VECTOR('',#24458,1000.);
#5564=VECTOR('',#24463,1000.);
#5565=VECTOR('',#24468,1000.);
#5566=VECTOR('',#24473,1000.);
#5567=VECTOR('',#24478,1000.);
#5568=VECTOR('',#24483,1000.);
#5569=VECTOR('',#24488,1000.);
#5570=VECTOR('',#24493,1000.);
#5571=VECTOR('',#24498,1000.);
#5572=VECTOR('',#24503,1000.);
#5573=VECTOR('',#24508,1000.);
#5574=VECTOR('',#24513,1000.);
#5575=VECTOR('',#24518,1000.);
#5576=VECTOR('',#24523,1000.);
#5577=VECTOR('',#24528,1000.);
#5578=VECTOR('',#24533,1000.);
#5579=VECTOR('',#24538,1000.);
#5580=VECTOR('',#24543,1000.);
#5581=VECTOR('',#24548,1000.);
#5582=VECTOR('',#24553,1000.);
#5583=VECTOR('',#24558,1000.);
#5584=VECTOR('',#24563,1000.);
#5585=VECTOR('',#24568,1000.);
#5919=CIRCLE('',#18449,2.);
#5920=CIRCLE('',#18450,2.3);
#5921=CIRCLE('',#18452,1.5);
#5922=CIRCLE('',#18453,1.5);
#5923=CIRCLE('',#18454,1.80000000000002);
#5924=CIRCLE('',#18456,2.);
#5925=CIRCLE('',#18457,2.);
#5926=CIRCLE('',#18458,2.3);
#5927=CIRCLE('',#18460,1.2);
#5928=CIRCLE('',#18461,1.50000000000002);
#5929=CIRCLE('',#18463,3.2);
#5930=CIRCLE('',#18464,3.49999999999998);
#5931=CIRCLE('',#18466,1.2);
#5932=CIRCLE('',#18467,1.2);
#5933=CIRCLE('',#18468,1.50000000000001);
#5934=CIRCLE('',#18470,2.);
#5935=CIRCLE('',#18471,2.);
#5936=CIRCLE('',#18472,2.3);
#5937=CIRCLE('',#18474,2.);
#5938=CIRCLE('',#18475,2.29999999999998);
#5939=CIRCLE('',#18477,1.5);
#5940=CIRCLE('',#18478,1.8);
#5941=CIRCLE('',#18480,3.2);
#5942=CIRCLE('',#18481,3.50000000000001);
#5943=CIRCLE('',#18483,2.);
#5944=CIRCLE('',#18484,2.);
#5945=CIRCLE('',#18486,2.);
#5946=CIRCLE('',#18494,4.3);
#5947=CIRCLE('',#18495,4.3);
#5948=CIRCLE('',#18498,4.29999999999998);
#5949=CIRCLE('',#18499,4.29999999999999);
#5950=CIRCLE('',#18503,3.3);
#5951=CIRCLE('',#18505,3.3);
#5952=CIRCLE('',#18507,4.);
#5953=CIRCLE('',#18508,4.);
#5954=CIRCLE('',#18512,4.);
#5955=CIRCLE('',#18513,4.);
#5956=CIRCLE('',#18521,3.);
#5957=CIRCLE('',#18526,3.);
#5958=CIRCLE('',#18528,3.);
#5959=CIRCLE('',#18531,3.);
#5960=CIRCLE('',#18533,0.300000000000002);
#5961=CIRCLE('',#18538,0.300000000000002);
#5962=CIRCLE('',#18539,0.300000000000002);
#5963=CIRCLE('',#18541,0.300000000000002);
#5964=CIRCLE('',#18543,0.300000000000002);
#5965=CIRCLE('',#18546,0.300000000000002);
#5966=CIRCLE('',#18548,0.300000000000002);
#5967=CIRCLE('',#18549,0.300000000000002);
#5968=CIRCLE('',#18553,0.300000000000002);
#5969=CIRCLE('',#18554,0.300000000000002);
#5970=CIRCLE('',#18556,0.300000000000002);
#5971=CIRCLE('',#18558,0.300000000000002);
#5972=CIRCLE('',#18560,0.300000000000002);
#5973=CIRCLE('',#18562,0.300000000000002);
#5974=CIRCLE('',#18564,0.300000000000002);
#5975=CIRCLE('',#18566,0.300000000000002);
#5976=CIRCLE('',#18568,0.300000000000002);
#5977=CIRCLE('',#18572,0.300000000000002);
#5978=CIRCLE('',#18574,0.300000000000002);
#5979=CIRCLE('',#18578,0.300000000000002);
#5980=CIRCLE('',#18581,0.300000000000002);
#5981=CIRCLE('',#18591,0.300000000000002);
#5982=CIRCLE('',#18598,1.1);
#5983=CIRCLE('',#18599,0.1);
#5984=CIRCLE('',#18600,1.2);
#5985=CIRCLE('',#18601,1.2);
#5986=CIRCLE('',#18603,1.2);
#5987=CIRCLE('',#18604,1.2);
#5988=CIRCLE('',#18605,0.1);
#5989=CIRCLE('',#18606,1.1);
#5990=CIRCLE('',#18611,2.5);
#5991=CIRCLE('',#18612,2.5);
#5992=CIRCLE('',#18614,3.);
#5993=CIRCLE('',#18615,3.);
#5994=CIRCLE('',#18616,3.);
#5995=CIRCLE('',#18617,3.);
#5996=CIRCLE('',#18619,4.25);
#5997=CIRCLE('',#18620,4.25);
#5998=CIRCLE('',#18622,1.2);
#5999=CIRCLE('',#18623,1.2);
#6000=CIRCLE('',#18625,1.2);
#6001=CIRCLE('',#18626,1.2);
#6002=CIRCLE('',#18628,2.);
#6003=CIRCLE('',#18629,2.);
#6004=CIRCLE('',#18632,1.5);
#6005=CIRCLE('',#18633,1.5);
#6006=CIRCLE('',#18637,1.5);
#6007=CIRCLE('',#18641,1.5);
#6008=CIRCLE('',#18651,2.5);
#6009=CIRCLE('',#18652,2.5);
#6010=CIRCLE('',#18654,5.5);
#6011=CIRCLE('',#18657,2.5);
#6012=CIRCLE('',#18658,0.5);
#6013=CIRCLE('',#18659,2.);
#6014=CIRCLE('',#18661,1.99814869273444);
#6015=CIRCLE('',#18662,1.99814869273444);
#6016=CIRCLE('',#18663,1.61);
#6017=CIRCLE('',#18665,2.);
#6018=CIRCLE('',#18666,2.);
#6019=CIRCLE('',#18667,1.61);
#6020=CIRCLE('',#18668,1.61);
#6021=CIRCLE('',#18671,2.);
#6022=CIRCLE('',#18672,2.);
#6023=CIRCLE('',#18674,2.);
#6024=CIRCLE('',#18675,2.);
#6025=CIRCLE('',#18676,1.61);
#6026=CIRCLE('',#18677,1.61);
#6027=CIRCLE('',#18680,2.);
#6028=CIRCLE('',#18681,2.);
#6029=CIRCLE('',#18683,2.);
#6030=CIRCLE('',#18684,2.);
#6031=CIRCLE('',#18685,1.61);
#6032=CIRCLE('',#18686,1.61);
#6033=CIRCLE('',#18689,2.);
#6034=CIRCLE('',#18690,2.);
#6035=CIRCLE('',#18692,2.);
#6036=CIRCLE('',#18693,2.);
#6037=CIRCLE('',#18694,1.61);
#6038=CIRCLE('',#18695,1.61);
#6039=CIRCLE('',#18698,2.);
#6040=CIRCLE('',#18699,2.);
#6041=CIRCLE('',#18701,2.);
#6042=CIRCLE('',#18702,2.);
#6043=CIRCLE('',#18703,1.61);
#6044=CIRCLE('',#18704,1.61);
#6045=CIRCLE('',#18707,2.);
#6046=CIRCLE('',#18708,2.);
#6047=CIRCLE('',#18710,2.);
#6048=CIRCLE('',#18711,2.);
#6049=CIRCLE('',#18712,1.61);
#6050=CIRCLE('',#18713,1.61);
#6051=CIRCLE('',#18716,2.);
#6052=CIRCLE('',#18717,2.);
#6053=CIRCLE('',#18719,2.);
#6054=CIRCLE('',#18720,2.);
#6055=CIRCLE('',#18721,1.61);
#6056=CIRCLE('',#18722,1.61);
#6057=CIRCLE('',#18725,2.);
#6058=CIRCLE('',#18726,2.);
#6059=CIRCLE('',#18728,2.);
#6060=CIRCLE('',#18729,2.);
#6061=CIRCLE('',#18730,1.61);
#6062=CIRCLE('',#18731,1.61);
#6063=CIRCLE('',#18734,2.);
#6064=CIRCLE('',#18735,2.);
#6065=CIRCLE('',#18737,2.);
#6066=CIRCLE('',#18738,2.);
#6067=CIRCLE('',#18739,1.61);
#6068=CIRCLE('',#18740,1.61);
#6069=CIRCLE('',#18743,2.);
#6070=CIRCLE('',#18744,2.);
#6071=CIRCLE('',#18746,2.);
#6072=CIRCLE('',#18747,2.);
#6073=CIRCLE('',#18748,1.61);
#6074=CIRCLE('',#18749,1.61);
#6075=CIRCLE('',#18752,2.);
#6076=CIRCLE('',#18753,2.);
#6077=CIRCLE('',#18755,2.);
#6078=CIRCLE('',#18756,2.);
#6079=CIRCLE('',#18757,1.61);
#6080=CIRCLE('',#18758,1.61);
#6081=CIRCLE('',#18761,2.);
#6082=CIRCLE('',#18762,2.);
#6083=CIRCLE('',#18764,2.);
#6084=CIRCLE('',#18765,2.);
#6085=CIRCLE('',#18766,1.61);
#6086=CIRCLE('',#18767,1.61);
#6087=CIRCLE('',#18770,2.);
#6088=CIRCLE('',#18771,2.);
#6089=CIRCLE('',#18773,2.);
#6090=CIRCLE('',#18774,2.);
#6091=CIRCLE('',#18775,1.61);
#6092=CIRCLE('',#18776,1.61);
#6093=CIRCLE('',#18779,2.);
#6094=CIRCLE('',#18780,2.);
#6095=CIRCLE('',#18782,2.);
#6096=CIRCLE('',#18783,2.);
#6097=CIRCLE('',#18784,1.61);
#6098=CIRCLE('',#18785,1.61);
#6099=CIRCLE('',#18788,2.);
#6100=CIRCLE('',#18789,2.);
#6101=CIRCLE('',#18791,2.);
#6102=CIRCLE('',#18792,2.);
#6103=CIRCLE('',#18793,1.61);
#6104=CIRCLE('',#18794,1.61);
#6105=CIRCLE('',#18797,8.175);
#6106=CIRCLE('',#18798,8.175);
#6107=CIRCLE('',#18799,8.175);
#6108=CIRCLE('',#18800,8.175);
#6109=CIRCLE('',#18801,8.175);
#6110=CIRCLE('',#18802,8.175);
#6111=CIRCLE('',#18803,8.175);
#6112=CIRCLE('',#18804,8.175);
#6113=CIRCLE('',#18805,8.175);
#6114=CIRCLE('',#18806,8.175);
#6115=CIRCLE('',#18807,8.175);
#6116=CIRCLE('',#18808,8.175);
#6117=CIRCLE('',#18809,8.175);
#6118=CIRCLE('',#18810,8.175);
#6119=CIRCLE('',#18811,8.175);
#6120=CIRCLE('',#18812,8.175);
#6121=CIRCLE('',#18813,8.175);
#6122=CIRCLE('',#18814,8.175);
#6123=CIRCLE('',#18815,8.175);
#6124=CIRCLE('',#18816,8.175);
#6125=CIRCLE('',#18817,8.175);
#6126=CIRCLE('',#18818,8.175);
#6127=CIRCLE('',#18819,8.175);
#6128=CIRCLE('',#18820,8.175);
#6129=CIRCLE('',#18821,8.175);
#6130=CIRCLE('',#18822,8.175);
#6131=CIRCLE('',#18823,8.175);
#6132=CIRCLE('',#18824,8.175);
#6133=CIRCLE('',#18825,8.175);
#6134=CIRCLE('',#18826,8.175);
#6135=CIRCLE('',#18827,8.175);
#6136=CIRCLE('',#18828,8.175);
#6137=CIRCLE('',#18829,8.175);
#6138=CIRCLE('',#18830,8.175);
#6139=CIRCLE('',#18831,8.175);
#6140=CIRCLE('',#18832,8.175);
#6141=CIRCLE('',#18833,8.175);
#6142=CIRCLE('',#18834,8.175);
#6143=CIRCLE('',#18835,8.175);
#6144=CIRCLE('',#18836,7.775);
#6145=CIRCLE('',#18837,8.175);
#6146=CIRCLE('',#18838,8.175);
#6147=CIRCLE('',#18839,8.175);
#6148=CIRCLE('',#18840,8.175);
#6149=CIRCLE('',#18841,8.175);
#6150=CIRCLE('',#18842,8.175);
#6151=CIRCLE('',#18843,8.175);
#6152=CIRCLE('',#18844,8.175);
#6153=CIRCLE('',#18845,8.175);
#6154=CIRCLE('',#18846,8.175);
#6155=CIRCLE('',#18847,8.175);
#6156=CIRCLE('',#18848,8.175);
#6157=CIRCLE('',#18849,8.175);
#6158=CIRCLE('',#18850,8.175);
#6159=CIRCLE('',#18851,8.175);
#6160=CIRCLE('',#18852,8.175);
#6161=CIRCLE('',#18853,8.175);
#6162=CIRCLE('',#18854,8.175);
#6163=CIRCLE('',#18855,8.175);
#6164=CIRCLE('',#18856,8.175);
#6165=CIRCLE('',#18857,8.175);
#6166=CIRCLE('',#18858,8.175);
#6167=CIRCLE('',#18859,8.175);
#6168=CIRCLE('',#18860,8.175);
#6169=CIRCLE('',#18861,8.175);
#6170=CIRCLE('',#18862,8.175);
#6171=CIRCLE('',#18863,8.175);
#6172=CIRCLE('',#18864,8.175);
#6173=CIRCLE('',#18865,8.175);
#6174=CIRCLE('',#18866,8.175);
#6175=CIRCLE('',#18867,8.175);
#6176=CIRCLE('',#18868,8.175);
#6177=CIRCLE('',#18869,8.175);
#6178=CIRCLE('',#18870,8.175);
#6179=CIRCLE('',#18871,8.175);
#6180=CIRCLE('',#18872,8.175);
#6181=CIRCLE('',#18873,8.175);
#6182=CIRCLE('',#18874,8.175);
#6183=CIRCLE('',#18876,8.175);
#6184=CIRCLE('',#18877,8.175);
#6185=CIRCLE('',#18878,8.175);
#6186=CIRCLE('',#18879,8.175);
#6187=CIRCLE('',#18880,8.175);
#6188=CIRCLE('',#18881,8.175);
#6189=CIRCLE('',#18882,8.175);
#6190=CIRCLE('',#18883,8.175);
#6191=CIRCLE('',#18884,8.175);
#6192=CIRCLE('',#18885,8.175);
#6193=CIRCLE('',#18886,8.175);
#6194=CIRCLE('',#18887,8.175);
#6195=CIRCLE('',#18888,8.175);
#6196=CIRCLE('',#18889,8.175);
#6197=CIRCLE('',#18890,8.175);
#6198=CIRCLE('',#18891,8.175);
#6199=CIRCLE('',#18892,8.175);
#6200=CIRCLE('',#18893,8.175);
#6201=CIRCLE('',#18894,8.175);
#6202=CIRCLE('',#18895,8.175);
#6203=CIRCLE('',#18896,8.175);
#6204=CIRCLE('',#18897,8.175);
#6205=CIRCLE('',#18898,8.175);
#6206=CIRCLE('',#18899,8.175);
#6207=CIRCLE('',#18900,8.175);
#6208=CIRCLE('',#18901,8.175);
#6209=CIRCLE('',#18902,8.175);
#6210=CIRCLE('',#18903,8.175);
#6211=CIRCLE('',#18904,8.175);
#6212=CIRCLE('',#18905,8.175);
#6213=CIRCLE('',#18906,8.175);
#6214=CIRCLE('',#18907,8.175);
#6215=CIRCLE('',#18908,8.175);
#6216=CIRCLE('',#18909,8.175);
#6217=CIRCLE('',#18910,8.175);
#6218=CIRCLE('',#18911,8.175);
#6219=CIRCLE('',#18912,8.175);
#6220=CIRCLE('',#18913,8.175);
#6221=CIRCLE('',#18914,8.175);
#6222=CIRCLE('',#18915,7.775);
#6223=CIRCLE('',#18916,8.175);
#6224=CIRCLE('',#18917,8.175);
#6225=CIRCLE('',#18918,8.175);
#6226=CIRCLE('',#18919,8.175);
#6227=CIRCLE('',#18920,8.175);
#6228=CIRCLE('',#18921,8.175);
#6229=CIRCLE('',#18922,8.175);
#6230=CIRCLE('',#18923,8.175);
#6231=CIRCLE('',#18924,8.175);
#6232=CIRCLE('',#18925,8.175);
#6233=CIRCLE('',#18926,8.175);
#6234=CIRCLE('',#18927,8.175);
#6235=CIRCLE('',#18928,8.175);
#6236=CIRCLE('',#18929,8.175);
#6237=CIRCLE('',#18930,8.175);
#6238=CIRCLE('',#18931,8.175);
#6239=CIRCLE('',#18932,8.175);
#6240=CIRCLE('',#18933,8.175);
#6241=CIRCLE('',#18934,8.175);
#6242=CIRCLE('',#18935,8.175);
#6243=CIRCLE('',#18936,8.175);
#6244=CIRCLE('',#18937,8.175);
#6245=CIRCLE('',#18938,8.175);
#6246=CIRCLE('',#18939,8.175);
#6247=CIRCLE('',#18940,8.175);
#6248=CIRCLE('',#18941,8.175);
#6249=CIRCLE('',#18942,8.175);
#6250=CIRCLE('',#18943,8.175);
#6251=CIRCLE('',#18944,8.175);
#6252=CIRCLE('',#18945,8.175);
#6253=CIRCLE('',#18946,8.175);
#6254=CIRCLE('',#18947,8.175);
#6255=CIRCLE('',#18948,8.175);
#6256=CIRCLE('',#18949,8.175);
#6257=CIRCLE('',#18950,8.175);
#6258=CIRCLE('',#18951,8.175);
#6259=CIRCLE('',#18952,8.175);
#6260=CIRCLE('',#18953,8.175);
#6261=CIRCLE('',#19190,2.69531878777687);
#6262=CIRCLE('',#19191,1.81782234903766);
#6263=CIRCLE('',#19192,2.69531878777687);
#6264=CIRCLE('',#19193,0.9);
#6265=CIRCLE('',#19194,2.71439757732023);
#6266=CIRCLE('',#19195,2.71439757732023);
#6267=CIRCLE('',#19196,2.69531878777687);
#6268=CIRCLE('',#19197,1.81782234903766);
#6269=CIRCLE('',#19199,2.8);
#6270=CIRCLE('',#19201,1.5);
#6271=CIRCLE('',#19202,1.5);
#6272=CIRCLE('',#19211,4.5);
#6273=CIRCLE('',#19212,0.5);
#6274=CIRCLE('',#19213,4.);
#6275=CIRCLE('',#19215,1.99909277054204);
#6276=CIRCLE('',#19216,1.99909277054204);
#6277=CIRCLE('',#19217,1.61);
#6278=CIRCLE('',#19219,2.);
#6279=CIRCLE('',#19220,2.);
#6280=CIRCLE('',#19221,1.61);
#6281=CIRCLE('',#19222,1.61);
#6282=CIRCLE('',#19225,2.);
#6283=CIRCLE('',#19226,2.);
#6284=CIRCLE('',#19228,2.);
#6285=CIRCLE('',#19229,2.);
#6286=CIRCLE('',#19230,1.61);
#6287=CIRCLE('',#19231,1.61);
#6288=CIRCLE('',#19234,2.);
#6289=CIRCLE('',#19235,2.);
#6290=CIRCLE('',#19237,2.);
#6291=CIRCLE('',#19238,2.);
#6292=CIRCLE('',#19239,1.61);
#6293=CIRCLE('',#19240,1.61);
#6294=CIRCLE('',#19243,2.);
#6295=CIRCLE('',#19244,2.);
#6296=CIRCLE('',#19246,2.);
#6297=CIRCLE('',#19247,2.);
#6298=CIRCLE('',#19248,1.61);
#6299=CIRCLE('',#19249,1.61);
#6300=CIRCLE('',#19252,2.);
#6301=CIRCLE('',#19253,2.);
#6302=CIRCLE('',#19255,2.);
#6303=CIRCLE('',#19256,2.);
#6304=CIRCLE('',#19257,1.61);
#6305=CIRCLE('',#19258,1.61);
#6306=CIRCLE('',#19261,2.);
#6307=CIRCLE('',#19262,2.);
#6308=CIRCLE('',#19264,2.);
#6309=CIRCLE('',#19265,2.);
#6310=CIRCLE('',#19266,1.61);
#6311=CIRCLE('',#19267,1.61);
#6312=CIRCLE('',#19270,2.);
#6313=CIRCLE('',#19271,2.);
#6314=CIRCLE('',#19273,2.);
#6315=CIRCLE('',#19274,2.);
#6316=CIRCLE('',#19275,1.61);
#6317=CIRCLE('',#19276,1.61);
#6318=CIRCLE('',#19279,2.);
#6319=CIRCLE('',#19280,2.);
#6320=CIRCLE('',#19282,2.);
#6321=CIRCLE('',#19283,2.);
#6322=CIRCLE('',#19284,1.61);
#6323=CIRCLE('',#19285,1.61);
#6324=CIRCLE('',#19288,2.);
#6325=CIRCLE('',#19289,2.);
#6326=CIRCLE('',#19291,2.);
#6327=CIRCLE('',#19292,2.);
#6328=CIRCLE('',#19293,1.61);
#6329=CIRCLE('',#19294,1.61);
#6330=CIRCLE('',#19297,2.);
#6331=CIRCLE('',#19298,2.);
#6332=CIRCLE('',#19300,2.);
#6333=CIRCLE('',#19301,2.);
#6334=CIRCLE('',#19302,1.61);
#6335=CIRCLE('',#19303,1.61);
#6336=CIRCLE('',#19306,2.);
#6337=CIRCLE('',#19307,2.);
#6338=CIRCLE('',#19309,2.);
#6339=CIRCLE('',#19310,2.);
#6340=CIRCLE('',#19311,1.61);
#6341=CIRCLE('',#19312,1.61);
#6342=CIRCLE('',#19315,2.);
#6343=CIRCLE('',#19316,2.);
#6344=CIRCLE('',#19318,2.);
#6345=CIRCLE('',#19319,2.);
#6346=CIRCLE('',#19320,1.61);
#6347=CIRCLE('',#19321,1.61);
#6348=CIRCLE('',#19324,2.);
#6349=CIRCLE('',#19325,2.);
#6350=CIRCLE('',#19327,2.);
#6351=CIRCLE('',#19328,2.);
#6352=CIRCLE('',#19329,1.61);
#6353=CIRCLE('',#19330,1.61);
#6354=CIRCLE('',#19333,4.);
#6355=CIRCLE('',#19335,8.175);
#6356=CIRCLE('',#19336,8.175);
#6357=CIRCLE('',#19337,8.175);
#6358=CIRCLE('',#19338,8.175);
#6359=CIRCLE('',#19339,8.175);
#6360=CIRCLE('',#19340,8.175);
#6361=CIRCLE('',#19341,8.175);
#6362=CIRCLE('',#19342,8.175);
#6363=CIRCLE('',#19343,8.175);
#6364=CIRCLE('',#19344,8.175);
#6365=CIRCLE('',#19345,8.175);
#6366=CIRCLE('',#19346,8.175);
#6367=CIRCLE('',#19347,8.175);
#6368=CIRCLE('',#19348,8.175);
#6369=CIRCLE('',#19349,8.175);
#6370=CIRCLE('',#19350,8.175);
#6371=CIRCLE('',#19351,8.175);
#6372=CIRCLE('',#19352,8.175);
#6373=CIRCLE('',#19353,8.175);
#6374=CIRCLE('',#19354,8.175);
#6375=CIRCLE('',#19355,8.175);
#6376=CIRCLE('',#19356,8.175);
#6377=CIRCLE('',#19357,8.175);
#6378=CIRCLE('',#19358,8.175);
#6379=CIRCLE('',#19359,8.175);
#6380=CIRCLE('',#19360,8.175);
#6381=CIRCLE('',#19361,8.175);
#6382=CIRCLE('',#19362,8.175);
#6383=CIRCLE('',#19363,8.175);
#6384=CIRCLE('',#19364,8.175);
#6385=CIRCLE('',#19365,8.175);
#6386=CIRCLE('',#19366,8.175);
#6387=CIRCLE('',#19367,8.175);
#6388=CIRCLE('',#19368,8.175);
#6389=CIRCLE('',#19369,8.175);
#6390=CIRCLE('',#19370,8.175);
#6391=CIRCLE('',#19371,8.175);
#6392=CIRCLE('',#19372,8.175);
#6393=CIRCLE('',#19373,8.175);
#6394=CIRCLE('',#19374,7.775);
#6395=CIRCLE('',#19375,8.175);
#6396=CIRCLE('',#19376,8.175);
#6397=CIRCLE('',#19377,8.175);
#6398=CIRCLE('',#19378,8.175);
#6399=CIRCLE('',#19379,8.175);
#6400=CIRCLE('',#19380,8.175);
#6401=CIRCLE('',#19381,8.175);
#6402=CIRCLE('',#19382,8.175);
#6403=CIRCLE('',#19383,8.175);
#6404=CIRCLE('',#19384,8.175);
#6405=CIRCLE('',#19385,8.175);
#6406=CIRCLE('',#19386,8.175);
#6407=CIRCLE('',#19387,8.175);
#6408=CIRCLE('',#19388,8.175);
#6409=CIRCLE('',#19389,8.175);
#6410=CIRCLE('',#19390,8.175);
#6411=CIRCLE('',#19391,8.175);
#6412=CIRCLE('',#19392,8.175);
#6413=CIRCLE('',#19393,8.175);
#6414=CIRCLE('',#19394,8.175);
#6415=CIRCLE('',#19395,8.175);
#6416=CIRCLE('',#19396,8.175);
#6417=CIRCLE('',#19397,8.175);
#6418=CIRCLE('',#19398,8.175);
#6419=CIRCLE('',#19399,8.175);
#6420=CIRCLE('',#19400,8.175);
#6421=CIRCLE('',#19401,8.175);
#6422=CIRCLE('',#19402,8.175);
#6423=CIRCLE('',#19403,8.175);
#6424=CIRCLE('',#19404,8.175);
#6425=CIRCLE('',#19405,8.175);
#6426=CIRCLE('',#19406,8.175);
#6427=CIRCLE('',#19407,8.175);
#6428=CIRCLE('',#19408,8.175);
#6429=CIRCLE('',#19409,8.175);
#6430=CIRCLE('',#19410,8.175);
#6431=CIRCLE('',#19411,8.175);
#6432=CIRCLE('',#19412,8.175);
#6433=CIRCLE('',#19414,8.175);
#6434=CIRCLE('',#19415,8.175);
#6435=CIRCLE('',#19416,8.175);
#6436=CIRCLE('',#19417,8.175);
#6437=CIRCLE('',#19418,8.175);
#6438=CIRCLE('',#19419,8.175);
#6439=CIRCLE('',#19420,8.175);
#6440=CIRCLE('',#19421,8.175);
#6441=CIRCLE('',#19422,8.175);
#6442=CIRCLE('',#19423,8.175);
#6443=CIRCLE('',#19424,8.175);
#6444=CIRCLE('',#19425,8.175);
#6445=CIRCLE('',#19426,8.175);
#6446=CIRCLE('',#19427,8.175);
#6447=CIRCLE('',#19428,8.175);
#6448=CIRCLE('',#19429,8.175);
#6449=CIRCLE('',#19430,8.175);
#6450=CIRCLE('',#19431,8.175);
#6451=CIRCLE('',#19432,8.175);
#6452=CIRCLE('',#19433,8.175);
#6453=CIRCLE('',#19434,8.175);
#6454=CIRCLE('',#19435,8.175);
#6455=CIRCLE('',#19436,8.175);
#6456=CIRCLE('',#19437,8.175);
#6457=CIRCLE('',#19438,8.175);
#6458=CIRCLE('',#19439,8.175);
#6459=CIRCLE('',#19440,8.175);
#6460=CIRCLE('',#19441,8.175);
#6461=CIRCLE('',#19442,8.175);
#6462=CIRCLE('',#19443,8.175);
#6463=CIRCLE('',#19444,8.175);
#6464=CIRCLE('',#19445,8.175);
#6465=CIRCLE('',#19446,8.175);
#6466=CIRCLE('',#19447,8.175);
#6467=CIRCLE('',#19448,8.175);
#6468=CIRCLE('',#19449,8.175);
#6469=CIRCLE('',#19450,8.175);
#6470=CIRCLE('',#19451,8.175);
#6471=CIRCLE('',#19452,8.175);
#6472=CIRCLE('',#19453,7.775);
#6473=CIRCLE('',#19454,8.175);
#6474=CIRCLE('',#19455,8.175);
#6475=CIRCLE('',#19456,8.175);
#6476=CIRCLE('',#19457,8.175);
#6477=CIRCLE('',#19458,8.175);
#6478=CIRCLE('',#19459,8.175);
#6479=CIRCLE('',#19460,8.175);
#6480=CIRCLE('',#19461,8.175);
#6481=CIRCLE('',#19462,8.175);
#6482=CIRCLE('',#19463,8.175);
#6483=CIRCLE('',#19464,8.175);
#6484=CIRCLE('',#19465,8.175);
#6485=CIRCLE('',#19466,8.175);
#6486=CIRCLE('',#19467,8.175);
#6487=CIRCLE('',#19468,8.175);
#6488=CIRCLE('',#19469,8.175);
#6489=CIRCLE('',#19470,8.175);
#6490=CIRCLE('',#19471,8.175);
#6491=CIRCLE('',#19472,8.175);
#6492=CIRCLE('',#19473,8.175);
#6493=CIRCLE('',#19474,8.175);
#6494=CIRCLE('',#19475,8.175);
#6495=CIRCLE('',#19476,8.175);
#6496=CIRCLE('',#19477,8.175);
#6497=CIRCLE('',#19478,8.175);
#6498=CIRCLE('',#19479,8.175);
#6499=CIRCLE('',#19480,8.175);
#6500=CIRCLE('',#19481,8.175);
#6501=CIRCLE('',#19482,8.175);
#6502=CIRCLE('',#19483,8.175);
#6503=CIRCLE('',#19484,8.175);
#6504=CIRCLE('',#19485,8.175);
#6505=CIRCLE('',#19486,8.175);
#6506=CIRCLE('',#19487,8.175);
#6507=CIRCLE('',#19488,8.175);
#6508=CIRCLE('',#19489,8.175);
#6509=CIRCLE('',#19490,8.175);
#6510=CIRCLE('',#19491,8.175);
#6511=CIRCLE('',#19493,2.);
#6961=VERTEX_POINT('',#33361);
#6962=VERTEX_POINT('',#33363);
#6963=VERTEX_POINT('',#33367);
#6964=VERTEX_POINT('',#33368);
#6965=VERTEX_POINT('',#33371);
#6966=VERTEX_POINT('',#33375);
#6967=VERTEX_POINT('',#33376);
#6968=VERTEX_POINT('',#33379);
#6969=VERTEX_POINT('',#33383);
#6970=VERTEX_POINT('',#33385);
#6971=VERTEX_POINT('',#33389);
#6972=VERTEX_POINT('',#33390);
#6973=VERTEX_POINT('',#33392);
#6974=VERTEX_POINT('',#33396);
#6975=VERTEX_POINT('',#33402);
#6976=VERTEX_POINT('',#33403);
#6977=VERTEX_POINT('',#33406);
#6978=VERTEX_POINT('',#33410);
#6979=VERTEX_POINT('',#33411);
#6980=VERTEX_POINT('',#33414);
#6981=VERTEX_POINT('',#33418);
#6982=VERTEX_POINT('',#33420);
#6983=VERTEX_POINT('',#33424);
#6984=VERTEX_POINT('',#33426);
#6985=VERTEX_POINT('',#33430);
#6986=VERTEX_POINT('',#33431);
#6987=VERTEX_POINT('',#33433);
#6988=VERTEX_POINT('',#33437);
#6989=VERTEX_POINT('',#33443);
#6990=VERTEX_POINT('',#33445);
#6991=VERTEX_POINT('',#33447);
#6992=VERTEX_POINT('',#33477);
#6993=VERTEX_POINT('',#33491);
#6994=VERTEX_POINT('',#33492);
#6995=VERTEX_POINT('',#33494);
#6996=VERTEX_POINT('',#33496);
#6997=VERTEX_POINT('',#33500);
#6998=VERTEX_POINT('',#33501);
#6999=VERTEX_POINT('',#33503);
#7000=VERTEX_POINT('',#33505);
#7001=VERTEX_POINT('',#33509);
#7002=VERTEX_POINT('',#33511);
#7003=VERTEX_POINT('',#33513);
#7004=VERTEX_POINT('',#33515);
#7005=VERTEX_POINT('',#33518);
#7006=VERTEX_POINT('',#33520);
#7007=VERTEX_POINT('',#33522);
#7008=VERTEX_POINT('',#33524);
#7009=VERTEX_POINT('',#33526);
#7010=VERTEX_POINT('',#33528);
#7011=VERTEX_POINT('',#33530);
#7012=VERTEX_POINT('',#33532);
#7013=VERTEX_POINT('',#33536);
#7014=VERTEX_POINT('',#33538);
#7015=VERTEX_POINT('',#33542);
#7016=VERTEX_POINT('',#33544);
#7017=VERTEX_POINT('',#33546);
#7018=VERTEX_POINT('',#33548);
#7019=VERTEX_POINT('',#33550);
#7020=VERTEX_POINT('',#33553);
#7021=VERTEX_POINT('',#33555);
#7022=VERTEX_POINT('',#33557);
#7023=VERTEX_POINT('',#33559);
#7024=VERTEX_POINT('',#33561);
#7025=VERTEX_POINT('',#33563);
#7026=VERTEX_POINT('',#33566);
#7027=VERTEX_POINT('',#33568);
#7028=VERTEX_POINT('',#33570);
#7029=VERTEX_POINT('',#33574);
#7030=VERTEX_POINT('',#33575);
#7031=VERTEX_POINT('',#33577);
#7032=VERTEX_POINT('',#33579);
#7033=VERTEX_POINT('',#33583);
#7034=VERTEX_POINT('',#33584);
#7035=VERTEX_POINT('',#33586);
#7036=VERTEX_POINT('',#33588);
#7037=VERTEX_POINT('',#33590);
#7038=VERTEX_POINT('',#33592);
#7039=VERTEX_POINT('',#33597);
#7040=VERTEX_POINT('',#33598);
#7041=VERTEX_POINT('',#33600);
#7042=VERTEX_POINT('',#33602);
#7043=VERTEX_POINT('',#33604);
#7044=VERTEX_POINT('',#33606);
#7045=VERTEX_POINT('',#33608);
#7046=VERTEX_POINT('',#33612);
#7047=VERTEX_POINT('',#33613);
#7048=VERTEX_POINT('',#33615);
#7049=VERTEX_POINT('',#33617);
#7050=VERTEX_POINT('',#33619);
#7051=VERTEX_POINT('',#33621);
#7052=VERTEX_POINT('',#33623);
#7053=VERTEX_POINT('',#33625);
#7054=VERTEX_POINT('',#33627);
#7055=VERTEX_POINT('',#33631);
#7056=VERTEX_POINT('',#33632);
#7057=VERTEX_POINT('',#33634);
#7058=VERTEX_POINT('',#33636);
#7059=VERTEX_POINT('',#33649);
#7060=VERTEX_POINT('',#33650);
#7061=VERTEX_POINT('',#33661);
#7062=VERTEX_POINT('',#33662);
#7063=VERTEX_POINT('',#33693);
#7064=VERTEX_POINT('',#33695);
#7065=VERTEX_POINT('',#33697);
#7066=VERTEX_POINT('',#33699);
#7067=VERTEX_POINT('',#33703);
#7068=VERTEX_POINT('',#33707);
#7069=VERTEX_POINT('',#33709);
#7070=VERTEX_POINT('',#33713);
#7071=VERTEX_POINT('',#33719);
#7072=VERTEX_POINT('',#33720);
#7073=VERTEX_POINT('',#33725);
#7074=VERTEX_POINT('',#33726);
#7075=VERTEX_POINT('',#33798);
#7076=VERTEX_POINT('',#33800);
#7077=VERTEX_POINT('',#33802);
#7078=VERTEX_POINT('',#33806);
#7079=VERTEX_POINT('',#33807);
#7080=VERTEX_POINT('',#33810);
#7081=VERTEX_POINT('',#33818);
#7082=VERTEX_POINT('',#33820);
#7083=VERTEX_POINT('',#33824);
#7084=VERTEX_POINT('',#33825);
#7085=VERTEX_POINT('',#33827);
#7086=VERTEX_POINT('',#33829);
#7087=VERTEX_POINT('',#33834);
#7088=VERTEX_POINT('',#33836);
#7089=VERTEX_POINT('',#33840);
#7090=VERTEX_POINT('',#33842);
#7091=VERTEX_POINT('',#33846);
#7092=VERTEX_POINT('',#33848);
#7093=VERTEX_POINT('',#33852);
#7094=VERTEX_POINT('',#33854);
#7095=VERTEX_POINT('',#33858);
#7096=VERTEX_POINT('',#33860);
#7097=VERTEX_POINT('',#33864);
#7098=VERTEX_POINT('',#33865);
#7099=VERTEX_POINT('',#33867);
#7100=VERTEX_POINT('',#33869);
#7101=VERTEX_POINT('',#33873);
#7102=VERTEX_POINT('',#33875);
#7103=VERTEX_POINT('',#33882);
#7104=VERTEX_POINT('',#33883);
#7105=VERTEX_POINT('',#33885);
#7106=VERTEX_POINT('',#33887);
#7107=VERTEX_POINT('',#33889);
#7108=VERTEX_POINT('',#33896);
#7109=VERTEX_POINT('',#33897);
#7110=VERTEX_POINT('',#33900);
#7111=VERTEX_POINT('',#33904);
#7112=VERTEX_POINT('',#33908);
#7113=VERTEX_POINT('',#33912);
#7114=VERTEX_POINT('',#33914);
#7115=VERTEX_POINT('',#33926);
#7116=VERTEX_POINT('',#33928);
#7117=VERTEX_POINT('',#33932);
#7118=VERTEX_POINT('',#33933);
#7119=VERTEX_POINT('',#33937);
#7120=VERTEX_POINT('',#33939);
#7121=VERTEX_POINT('',#33943);
#7122=VERTEX_POINT('',#33944);
#7123=VERTEX_POINT('',#33947);
#7124=VERTEX_POINT('',#33951);
#7125=VERTEX_POINT('',#33952);
#7126=VERTEX_POINT('',#33955);
#7127=VERTEX_POINT('',#33957);
#7128=VERTEX_POINT('',#33963);
#7129=VERTEX_POINT('',#33964);
#7130=VERTEX_POINT('',#33969);
#7131=VERTEX_POINT('',#33970);
#7132=VERTEX_POINT('',#33973);
#7133=VERTEX_POINT('',#33975);
#7134=VERTEX_POINT('',#33981);
#7135=VERTEX_POINT('',#33982);
#7136=VERTEX_POINT('',#33987);
#7137=VERTEX_POINT('',#33988);
#7138=VERTEX_POINT('',#33991);
#7139=VERTEX_POINT('',#33993);
#7140=VERTEX_POINT('',#33999);
#7141=VERTEX_POINT('',#34000);
#7142=VERTEX_POINT('',#34005);
#7143=VERTEX_POINT('',#34006);
#7144=VERTEX_POINT('',#34009);
#7145=VERTEX_POINT('',#34011);
#7146=VERTEX_POINT('',#34017);
#7147=VERTEX_POINT('',#34018);
#7148=VERTEX_POINT('',#34023);
#7149=VERTEX_POINT('',#34024);
#7150=VERTEX_POINT('',#34027);
#7151=VERTEX_POINT('',#34029);
#7152=VERTEX_POINT('',#34035);
#7153=VERTEX_POINT('',#34036);
#7154=VERTEX_POINT('',#34041);
#7155=VERTEX_POINT('',#34042);
#7156=VERTEX_POINT('',#34045);
#7157=VERTEX_POINT('',#34047);
#7158=VERTEX_POINT('',#34053);
#7159=VERTEX_POINT('',#34054);
#7160=VERTEX_POINT('',#34059);
#7161=VERTEX_POINT('',#34060);
#7162=VERTEX_POINT('',#34063);
#7163=VERTEX_POINT('',#34065);
#7164=VERTEX_POINT('',#34071);
#7165=VERTEX_POINT('',#34072);
#7166=VERTEX_POINT('',#34077);
#7167=VERTEX_POINT('',#34078);
#7168=VERTEX_POINT('',#34081);
#7169=VERTEX_POINT('',#34083);
#7170=VERTEX_POINT('',#34089);
#7171=VERTEX_POINT('',#34090);
#7172=VERTEX_POINT('',#34095);
#7173=VERTEX_POINT('',#34096);
#7174=VERTEX_POINT('',#34099);
#7175=VERTEX_POINT('',#34101);
#7176=VERTEX_POINT('',#34107);
#7177=VERTEX_POINT('',#34108);
#7178=VERTEX_POINT('',#34113);
#7179=VERTEX_POINT('',#34114);
#7180=VERTEX_POINT('',#34117);
#7181=VERTEX_POINT('',#34119);
#7182=VERTEX_POINT('',#34125);
#7183=VERTEX_POINT('',#34126);
#7184=VERTEX_POINT('',#34131);
#7185=VERTEX_POINT('',#34132);
#7186=VERTEX_POINT('',#34135);
#7187=VERTEX_POINT('',#34137);
#7188=VERTEX_POINT('',#34143);
#7189=VERTEX_POINT('',#34144);
#7190=VERTEX_POINT('',#34149);
#7191=VERTEX_POINT('',#34150);
#7192=VERTEX_POINT('',#34153);
#7193=VERTEX_POINT('',#34155);
#7194=VERTEX_POINT('',#34161);
#7195=VERTEX_POINT('',#34162);
#7196=VERTEX_POINT('',#34167);
#7197=VERTEX_POINT('',#34168);
#7198=VERTEX_POINT('',#34171);
#7199=VERTEX_POINT('',#34173);
#7200=VERTEX_POINT('',#34179);
#7201=VERTEX_POINT('',#34180);
#7202=VERTEX_POINT('',#34185);
#7203=VERTEX_POINT('',#34186);
#7204=VERTEX_POINT('',#34189);
#7205=VERTEX_POINT('',#34191);
#7206=VERTEX_POINT('',#34197);
#7207=VERTEX_POINT('',#34198);
#7208=VERTEX_POINT('',#34203);
#7209=VERTEX_POINT('',#34204);
#7210=VERTEX_POINT('',#34207);
#7211=VERTEX_POINT('',#34209);
#7212=VERTEX_POINT('',#34215);
#7213=VERTEX_POINT('',#34216);
#7214=VERTEX_POINT('',#34220);
#7215=VERTEX_POINT('',#34222);
#7216=VERTEX_POINT('',#34226);
#7217=VERTEX_POINT('',#34230);
#7218=VERTEX_POINT('',#34232);
#7219=VERTEX_POINT('',#34236);
#7220=VERTEX_POINT('',#34240);
#7221=VERTEX_POINT('',#34242);
#7222=VERTEX_POINT('',#34246);
#7223=VERTEX_POINT('',#34250);
#7224=VERTEX_POINT('',#34252);
#7225=VERTEX_POINT('',#34256);
#7226=VERTEX_POINT('',#34260);
#7227=VERTEX_POINT('',#34262);
#7228=VERTEX_POINT('',#34266);
#7229=VERTEX_POINT('',#34270);
#7230=VERTEX_POINT('',#34272);
#7231=VERTEX_POINT('',#34276);
#7232=VERTEX_POINT('',#34280);
#7233=VERTEX_POINT('',#34282);
#7234=VERTEX_POINT('',#34286);
#7235=VERTEX_POINT('',#34290);
#7236=VERTEX_POINT('',#34292);
#7237=VERTEX_POINT('',#34296);
#7238=VERTEX_POINT('',#34300);
#7239=VERTEX_POINT('',#34302);
#7240=VERTEX_POINT('',#34306);
#7241=VERTEX_POINT('',#34310);
#7242=VERTEX_POINT('',#34312);
#7243=VERTEX_POINT('',#34316);
#7244=VERTEX_POINT('',#34320);
#7245=VERTEX_POINT('',#34322);
#7246=VERTEX_POINT('',#34326);
#7247=VERTEX_POINT('',#34330);
#7248=VERTEX_POINT('',#34332);
#7249=VERTEX_POINT('',#34336);
#7250=VERTEX_POINT('',#34340);
#7251=VERTEX_POINT('',#34342);
#7252=VERTEX_POINT('',#34346);
#7253=VERTEX_POINT('',#34350);
#7254=VERTEX_POINT('',#34352);
#7255=VERTEX_POINT('',#34356);
#7256=VERTEX_POINT('',#34360);
#7257=VERTEX_POINT('',#34362);
#7258=VERTEX_POINT('',#34366);
#7259=VERTEX_POINT('',#34370);
#7260=VERTEX_POINT('',#34372);
#7261=VERTEX_POINT('',#34376);
#7262=VERTEX_POINT('',#34380);
#7263=VERTEX_POINT('',#34382);
#7264=VERTEX_POINT('',#34386);
#7265=VERTEX_POINT('',#34390);
#7266=VERTEX_POINT('',#34392);
#7267=VERTEX_POINT('',#34396);
#7268=VERTEX_POINT('',#34400);
#7269=VERTEX_POINT('',#34402);
#7270=VERTEX_POINT('',#34406);
#7271=VERTEX_POINT('',#34410);
#7272=VERTEX_POINT('',#34412);
#7273=VERTEX_POINT('',#34416);
#7274=VERTEX_POINT('',#34420);
#7275=VERTEX_POINT('',#34422);
#7276=VERTEX_POINT('',#34426);
#7277=VERTEX_POINT('',#34430);
#7278=VERTEX_POINT('',#34432);
#7279=VERTEX_POINT('',#34436);
#7280=VERTEX_POINT('',#34440);
#7281=VERTEX_POINT('',#34442);
#7282=VERTEX_POINT('',#34446);
#7283=VERTEX_POINT('',#34450);
#7284=VERTEX_POINT('',#34452);
#7285=VERTEX_POINT('',#34456);
#7286=VERTEX_POINT('',#34460);
#7287=VERTEX_POINT('',#34462);
#7288=VERTEX_POINT('',#34466);
#7289=VERTEX_POINT('',#34470);
#7290=VERTEX_POINT('',#34472);
#7291=VERTEX_POINT('',#34476);
#7292=VERTEX_POINT('',#34480);
#7293=VERTEX_POINT('',#34482);
#7294=VERTEX_POINT('',#34486);
#7295=VERTEX_POINT('',#34490);
#7296=VERTEX_POINT('',#34492);
#7297=VERTEX_POINT('',#34496);
#7298=VERTEX_POINT('',#34500);
#7299=VERTEX_POINT('',#34502);
#7300=VERTEX_POINT('',#34506);
#7301=VERTEX_POINT('',#34510);
#7302=VERTEX_POINT('',#34512);
#7303=VERTEX_POINT('',#34516);
#7304=VERTEX_POINT('',#34520);
#7305=VERTEX_POINT('',#34522);
#7306=VERTEX_POINT('',#34526);
#7307=VERTEX_POINT('',#34530);
#7308=VERTEX_POINT('',#34532);
#7309=VERTEX_POINT('',#34536);
#7310=VERTEX_POINT('',#34540);
#7311=VERTEX_POINT('',#34542);
#7312=VERTEX_POINT('',#34546);
#7313=VERTEX_POINT('',#34550);
#7314=VERTEX_POINT('',#34552);
#7315=VERTEX_POINT('',#34556);
#7316=VERTEX_POINT('',#34560);
#7317=VERTEX_POINT('',#34562);
#7318=VERTEX_POINT('',#34566);
#7319=VERTEX_POINT('',#34570);
#7320=VERTEX_POINT('',#34572);
#7321=VERTEX_POINT('',#34576);
#7322=VERTEX_POINT('',#34580);
#7323=VERTEX_POINT('',#34582);
#7324=VERTEX_POINT('',#34586);
#7325=VERTEX_POINT('',#34590);
#7326=VERTEX_POINT('',#34592);
#7327=VERTEX_POINT('',#34596);
#7328=VERTEX_POINT('',#34600);
#7329=VERTEX_POINT('',#34602);
#7330=VERTEX_POINT('',#34606);
#7331=VERTEX_POINT('',#34609);
#7332=VERTEX_POINT('',#34613);
#7333=VERTEX_POINT('',#34617);
#7334=VERTEX_POINT('',#34619);
#7335=VERTEX_POINT('',#34623);
#7336=VERTEX_POINT('',#34627);
#7337=VERTEX_POINT('',#34629);
#7338=VERTEX_POINT('',#34633);
#7339=VERTEX_POINT('',#34637);
#7340=VERTEX_POINT('',#34639);
#7341=VERTEX_POINT('',#34643);
#7342=VERTEX_POINT('',#34647);
#7343=VERTEX_POINT('',#34649);
#7344=VERTEX_POINT('',#34653);
#7345=VERTEX_POINT('',#34657);
#7346=VERTEX_POINT('',#34659);
#7347=VERTEX_POINT('',#34663);
#7348=VERTEX_POINT('',#34667);
#7349=VERTEX_POINT('',#34669);
#7350=VERTEX_POINT('',#34673);
#7351=VERTEX_POINT('',#34677);
#7352=VERTEX_POINT('',#34679);
#7353=VERTEX_POINT('',#34683);
#7354=VERTEX_POINT('',#34687);
#7355=VERTEX_POINT('',#34689);
#7356=VERTEX_POINT('',#34693);
#7357=VERTEX_POINT('',#34697);
#7358=VERTEX_POINT('',#34699);
#7359=VERTEX_POINT('',#34703);
#7360=VERTEX_POINT('',#34707);
#7361=VERTEX_POINT('',#34709);
#7362=VERTEX_POINT('',#34713);
#7363=VERTEX_POINT('',#34717);
#7364=VERTEX_POINT('',#34719);
#7365=VERTEX_POINT('',#34723);
#7366=VERTEX_POINT('',#34727);
#7367=VERTEX_POINT('',#34729);
#7368=VERTEX_POINT('',#34733);
#7369=VERTEX_POINT('',#34737);
#7370=VERTEX_POINT('',#34739);
#7371=VERTEX_POINT('',#34743);
#7372=VERTEX_POINT('',#34747);
#7373=VERTEX_POINT('',#34749);
#7374=VERTEX_POINT('',#34753);
#7375=VERTEX_POINT('',#34757);
#7376=VERTEX_POINT('',#34759);
#7377=VERTEX_POINT('',#34763);
#7378=VERTEX_POINT('',#34767);
#7379=VERTEX_POINT('',#34769);
#7380=VERTEX_POINT('',#34773);
#7381=VERTEX_POINT('',#34777);
#7382=VERTEX_POINT('',#34779);
#7383=VERTEX_POINT('',#34783);
#7384=VERTEX_POINT('',#34787);
#7385=VERTEX_POINT('',#34789);
#7386=VERTEX_POINT('',#34793);
#7387=VERTEX_POINT('',#34797);
#7388=VERTEX_POINT('',#34799);
#7389=VERTEX_POINT('',#34803);
#7390=VERTEX_POINT('',#34807);
#7391=VERTEX_POINT('',#34809);
#7392=VERTEX_POINT('',#34813);
#7393=VERTEX_POINT('',#34817);
#7394=VERTEX_POINT('',#34819);
#7395=VERTEX_POINT('',#34823);
#7396=VERTEX_POINT('',#34827);
#7397=VERTEX_POINT('',#34829);
#7398=VERTEX_POINT('',#34833);
#7399=VERTEX_POINT('',#34837);
#7400=VERTEX_POINT('',#34839);
#7401=VERTEX_POINT('',#34843);
#7402=VERTEX_POINT('',#34847);
#7403=VERTEX_POINT('',#34849);
#7404=VERTEX_POINT('',#34853);
#7405=VERTEX_POINT('',#34857);
#7406=VERTEX_POINT('',#34859);
#7407=VERTEX_POINT('',#34863);
#7408=VERTEX_POINT('',#34867);
#7409=VERTEX_POINT('',#34869);
#7410=VERTEX_POINT('',#34873);
#7411=VERTEX_POINT('',#34877);
#7412=VERTEX_POINT('',#34879);
#7413=VERTEX_POINT('',#34883);
#7414=VERTEX_POINT('',#34887);
#7415=VERTEX_POINT('',#34889);
#7416=VERTEX_POINT('',#34893);
#7417=VERTEX_POINT('',#34897);
#7418=VERTEX_POINT('',#34899);
#7419=VERTEX_POINT('',#34903);
#7420=VERTEX_POINT('',#34907);
#7421=VERTEX_POINT('',#34909);
#7422=VERTEX_POINT('',#34913);
#7423=VERTEX_POINT('',#34917);
#7424=VERTEX_POINT('',#34919);
#7425=VERTEX_POINT('',#34923);
#7426=VERTEX_POINT('',#34927);
#7427=VERTEX_POINT('',#34929);
#7428=VERTEX_POINT('',#34933);
#7429=VERTEX_POINT('',#34937);
#7430=VERTEX_POINT('',#34939);
#7431=VERTEX_POINT('',#34943);
#7432=VERTEX_POINT('',#34947);
#7433=VERTEX_POINT('',#34949);
#7434=VERTEX_POINT('',#34953);
#7435=VERTEX_POINT('',#34957);
#7436=VERTEX_POINT('',#34959);
#7437=VERTEX_POINT('',#34963);
#7438=VERTEX_POINT('',#34967);
#7439=VERTEX_POINT('',#34969);
#7440=VERTEX_POINT('',#34973);
#7441=VERTEX_POINT('',#34977);
#7442=VERTEX_POINT('',#34979);
#7443=VERTEX_POINT('',#34983);
#7444=VERTEX_POINT('',#34987);
#7445=VERTEX_POINT('',#34993);
#7446=VERTEX_POINT('',#34994);
#7447=VERTEX_POINT('',#34998);
#7448=VERTEX_POINT('',#35000);
#7449=VERTEX_POINT('',#35004);
#7450=VERTEX_POINT('',#35008);
#7451=VERTEX_POINT('',#35010);
#7452=VERTEX_POINT('',#35014);
#7453=VERTEX_POINT('',#35018);
#7454=VERTEX_POINT('',#35020);
#7455=VERTEX_POINT('',#35024);
#7456=VERTEX_POINT('',#35028);
#7457=VERTEX_POINT('',#35030);
#7458=VERTEX_POINT('',#35034);
#7459=VERTEX_POINT('',#35038);
#7460=VERTEX_POINT('',#35040);
#7461=VERTEX_POINT('',#35044);
#7462=VERTEX_POINT('',#35048);
#7463=VERTEX_POINT('',#35050);
#7464=VERTEX_POINT('',#35054);
#7465=VERTEX_POINT('',#35058);
#7466=VERTEX_POINT('',#35060);
#7467=VERTEX_POINT('',#35064);
#7468=VERTEX_POINT('',#35068);
#7469=VERTEX_POINT('',#35070);
#7470=VERTEX_POINT('',#35074);
#7471=VERTEX_POINT('',#35078);
#7472=VERTEX_POINT('',#35080);
#7473=VERTEX_POINT('',#35084);
#7474=VERTEX_POINT('',#35088);
#7475=VERTEX_POINT('',#35090);
#7476=VERTEX_POINT('',#35094);
#7477=VERTEX_POINT('',#35098);
#7478=VERTEX_POINT('',#35100);
#7479=VERTEX_POINT('',#35104);
#7480=VERTEX_POINT('',#35108);
#7481=VERTEX_POINT('',#35110);
#7482=VERTEX_POINT('',#35114);
#7483=VERTEX_POINT('',#35118);
#7484=VERTEX_POINT('',#35120);
#7485=VERTEX_POINT('',#35124);
#7486=VERTEX_POINT('',#35128);
#7487=VERTEX_POINT('',#35130);
#7488=VERTEX_POINT('',#35134);
#7489=VERTEX_POINT('',#35138);
#7490=VERTEX_POINT('',#35140);
#7491=VERTEX_POINT('',#35144);
#7492=VERTEX_POINT('',#35148);
#7493=VERTEX_POINT('',#35150);
#7494=VERTEX_POINT('',#35154);
#7495=VERTEX_POINT('',#35158);
#7496=VERTEX_POINT('',#35160);
#7497=VERTEX_POINT('',#35164);
#7498=VERTEX_POINT('',#35168);
#7499=VERTEX_POINT('',#35170);
#7500=VERTEX_POINT('',#35174);
#7501=VERTEX_POINT('',#35178);
#7502=VERTEX_POINT('',#35180);
#7503=VERTEX_POINT('',#35184);
#7504=VERTEX_POINT('',#35188);
#7505=VERTEX_POINT('',#35190);
#7506=VERTEX_POINT('',#35194);
#7507=VERTEX_POINT('',#35198);
#7508=VERTEX_POINT('',#35200);
#7509=VERTEX_POINT('',#35204);
#7510=VERTEX_POINT('',#35208);
#7511=VERTEX_POINT('',#35210);
#7512=VERTEX_POINT('',#35214);
#7513=VERTEX_POINT('',#35218);
#7514=VERTEX_POINT('',#35220);
#7515=VERTEX_POINT('',#35224);
#7516=VERTEX_POINT('',#35228);
#7517=VERTEX_POINT('',#35230);
#7518=VERTEX_POINT('',#35234);
#7519=VERTEX_POINT('',#35238);
#7520=VERTEX_POINT('',#35240);
#7521=VERTEX_POINT('',#35244);
#7522=VERTEX_POINT('',#35248);
#7523=VERTEX_POINT('',#35250);
#7524=VERTEX_POINT('',#35254);
#7525=VERTEX_POINT('',#35258);
#7526=VERTEX_POINT('',#35260);
#7527=VERTEX_POINT('',#35264);
#7528=VERTEX_POINT('',#35268);
#7529=VERTEX_POINT('',#35270);
#7530=VERTEX_POINT('',#35274);
#7531=VERTEX_POINT('',#35278);
#7532=VERTEX_POINT('',#35280);
#7533=VERTEX_POINT('',#35284);
#7534=VERTEX_POINT('',#35288);
#7535=VERTEX_POINT('',#35290);
#7536=VERTEX_POINT('',#35294);
#7537=VERTEX_POINT('',#35298);
#7538=VERTEX_POINT('',#35300);
#7539=VERTEX_POINT('',#35304);
#7540=VERTEX_POINT('',#35308);
#7541=VERTEX_POINT('',#35310);
#7542=VERTEX_POINT('',#35314);
#7543=VERTEX_POINT('',#35318);
#7544=VERTEX_POINT('',#35320);
#7545=VERTEX_POINT('',#35324);
#7546=VERTEX_POINT('',#35328);
#7547=VERTEX_POINT('',#35330);
#7548=VERTEX_POINT('',#35334);
#7549=VERTEX_POINT('',#35338);
#7550=VERTEX_POINT('',#35340);
#7551=VERTEX_POINT('',#35344);
#7552=VERTEX_POINT('',#35348);
#7553=VERTEX_POINT('',#35350);
#7554=VERTEX_POINT('',#35354);
#7555=VERTEX_POINT('',#35358);
#7556=VERTEX_POINT('',#35360);
#7557=VERTEX_POINT('',#35364);
#7558=VERTEX_POINT('',#35368);
#7559=VERTEX_POINT('',#35370);
#7560=VERTEX_POINT('',#35374);
#7561=VERTEX_POINT('',#35378);
#7562=VERTEX_POINT('',#35380);
#7563=VERTEX_POINT('',#35384);
#7564=VERTEX_POINT('',#35387);
#7565=VERTEX_POINT('',#35391);
#7566=VERTEX_POINT('',#35395);
#7567=VERTEX_POINT('',#35397);
#7568=VERTEX_POINT('',#35401);
#7569=VERTEX_POINT('',#35405);
#7570=VERTEX_POINT('',#35407);
#7571=VERTEX_POINT('',#35411);
#7572=VERTEX_POINT('',#35415);
#7573=VERTEX_POINT('',#35417);
#7574=VERTEX_POINT('',#35421);
#7575=VERTEX_POINT('',#35425);
#7576=VERTEX_POINT('',#35427);
#7577=VERTEX_POINT('',#35431);
#7578=VERTEX_POINT('',#35435);
#7579=VERTEX_POINT('',#35437);
#7580=VERTEX_POINT('',#35441);
#7581=VERTEX_POINT('',#35445);
#7582=VERTEX_POINT('',#35447);
#7583=VERTEX_POINT('',#35451);
#7584=VERTEX_POINT('',#35455);
#7585=VERTEX_POINT('',#35457);
#7586=VERTEX_POINT('',#35461);
#7587=VERTEX_POINT('',#35465);
#7588=VERTEX_POINT('',#35467);
#7589=VERTEX_POINT('',#35471);
#7590=VERTEX_POINT('',#35475);
#7591=VERTEX_POINT('',#35477);
#7592=VERTEX_POINT('',#35481);
#7593=VERTEX_POINT('',#35485);
#7594=VERTEX_POINT('',#35487);
#7595=VERTEX_POINT('',#35491);
#7596=VERTEX_POINT('',#35495);
#7597=VERTEX_POINT('',#35497);
#7598=VERTEX_POINT('',#35501);
#7599=VERTEX_POINT('',#35505);
#7600=VERTEX_POINT('',#35507);
#7601=VERTEX_POINT('',#35511);
#7602=VERTEX_POINT('',#35515);
#7603=VERTEX_POINT('',#35517);
#7604=VERTEX_POINT('',#35521);
#7605=VERTEX_POINT('',#35525);
#7606=VERTEX_POINT('',#35527);
#7607=VERTEX_POINT('',#35531);
#7608=VERTEX_POINT('',#35535);
#7609=VERTEX_POINT('',#35537);
#7610=VERTEX_POINT('',#35541);
#7611=VERTEX_POINT('',#35545);
#7612=VERTEX_POINT('',#35547);
#7613=VERTEX_POINT('',#35551);
#7614=VERTEX_POINT('',#35555);
#7615=VERTEX_POINT('',#35557);
#7616=VERTEX_POINT('',#35561);
#7617=VERTEX_POINT('',#35565);
#7618=VERTEX_POINT('',#35567);
#7619=VERTEX_POINT('',#35571);
#7620=VERTEX_POINT('',#35575);
#7621=VERTEX_POINT('',#35577);
#7622=VERTEX_POINT('',#35581);
#7623=VERTEX_POINT('',#35585);
#7624=VERTEX_POINT('',#35587);
#7625=VERTEX_POINT('',#35591);
#7626=VERTEX_POINT('',#35595);
#7627=VERTEX_POINT('',#35597);
#7628=VERTEX_POINT('',#35601);
#7629=VERTEX_POINT('',#35605);
#7630=VERTEX_POINT('',#35607);
#7631=VERTEX_POINT('',#35611);
#7632=VERTEX_POINT('',#35615);
#7633=VERTEX_POINT('',#35617);
#7634=VERTEX_POINT('',#35621);
#7635=VERTEX_POINT('',#35625);
#7636=VERTEX_POINT('',#35627);
#7637=VERTEX_POINT('',#35631);
#7638=VERTEX_POINT('',#35635);
#7639=VERTEX_POINT('',#35637);
#7640=VERTEX_POINT('',#35641);
#7641=VERTEX_POINT('',#35645);
#7642=VERTEX_POINT('',#35647);
#7643=VERTEX_POINT('',#35651);
#7644=VERTEX_POINT('',#35655);
#7645=VERTEX_POINT('',#35657);
#7646=VERTEX_POINT('',#35661);
#7647=VERTEX_POINT('',#35665);
#7648=VERTEX_POINT('',#35667);
#7649=VERTEX_POINT('',#35671);
#7650=VERTEX_POINT('',#35675);
#7651=VERTEX_POINT('',#35677);
#7652=VERTEX_POINT('',#35681);
#7653=VERTEX_POINT('',#35685);
#7654=VERTEX_POINT('',#35687);
#7655=VERTEX_POINT('',#35691);
#7656=VERTEX_POINT('',#35695);
#7657=VERTEX_POINT('',#35697);
#7658=VERTEX_POINT('',#35701);
#7659=VERTEX_POINT('',#35705);
#7660=VERTEX_POINT('',#35707);
#7661=VERTEX_POINT('',#35711);
#7662=VERTEX_POINT('',#35715);
#7663=VERTEX_POINT('',#35717);
#7664=VERTEX_POINT('',#35721);
#7665=VERTEX_POINT('',#35725);
#7666=VERTEX_POINT('',#35727);
#7667=VERTEX_POINT('',#35731);
#7668=VERTEX_POINT('',#35735);
#7669=VERTEX_POINT('',#35737);
#7670=VERTEX_POINT('',#35741);
#7671=VERTEX_POINT('',#35745);
#7672=VERTEX_POINT('',#35747);
#7673=VERTEX_POINT('',#35751);
#7674=VERTEX_POINT('',#35755);
#7675=VERTEX_POINT('',#35757);
#7676=VERTEX_POINT('',#35761);
#7677=VERTEX_POINT('',#35765);
#7678=VERTEX_POINT('',#36238);
#7679=VERTEX_POINT('',#36239);
#7680=VERTEX_POINT('',#36241);
#7681=VERTEX_POINT('',#36252);
#7682=VERTEX_POINT('',#36254);
#7683=VERTEX_POINT('',#36265);
#7684=VERTEX_POINT('',#36267);
#7685=VERTEX_POINT('',#36269);
#7686=VERTEX_POINT('',#36272);
#7687=VERTEX_POINT('',#36274);
#7688=VERTEX_POINT('',#36285);
#7689=VERTEX_POINT('',#36298);
#7690=VERTEX_POINT('',#36302);
#7691=VERTEX_POINT('',#36304);
#7692=VERTEX_POINT('',#36319);
#7693=VERTEX_POINT('',#36321);
#7694=VERTEX_POINT('',#36325);
#7695=VERTEX_POINT('',#36326);
#7696=VERTEX_POINT('',#36329);
#7697=VERTEX_POINT('',#36333);
#7698=VERTEX_POINT('',#36334);
#7699=VERTEX_POINT('',#36337);
#7700=VERTEX_POINT('',#36339);
#7701=VERTEX_POINT('',#36345);
#7702=VERTEX_POINT('',#36346);
#7703=VERTEX_POINT('',#36351);
#7704=VERTEX_POINT('',#36352);
#7705=VERTEX_POINT('',#36355);
#7706=VERTEX_POINT('',#36357);
#7707=VERTEX_POINT('',#36363);
#7708=VERTEX_POINT('',#36364);
#7709=VERTEX_POINT('',#36369);
#7710=VERTEX_POINT('',#36370);
#7711=VERTEX_POINT('',#36373);
#7712=VERTEX_POINT('',#36375);
#7713=VERTEX_POINT('',#36381);
#7714=VERTEX_POINT('',#36382);
#7715=VERTEX_POINT('',#36387);
#7716=VERTEX_POINT('',#36388);
#7717=VERTEX_POINT('',#36391);
#7718=VERTEX_POINT('',#36393);
#7719=VERTEX_POINT('',#36399);
#7720=VERTEX_POINT('',#36400);
#7721=VERTEX_POINT('',#36405);
#7722=VERTEX_POINT('',#36406);
#7723=VERTEX_POINT('',#36409);
#7724=VERTEX_POINT('',#36411);
#7725=VERTEX_POINT('',#36417);
#7726=VERTEX_POINT('',#36418);
#7727=VERTEX_POINT('',#36423);
#7728=VERTEX_POINT('',#36424);
#7729=VERTEX_POINT('',#36427);
#7730=VERTEX_POINT('',#36429);
#7731=VERTEX_POINT('',#36435);
#7732=VERTEX_POINT('',#36436);
#7733=VERTEX_POINT('',#36441);
#7734=VERTEX_POINT('',#36442);
#7735=VERTEX_POINT('',#36445);
#7736=VERTEX_POINT('',#36447);
#7737=VERTEX_POINT('',#36453);
#7738=VERTEX_POINT('',#36454);
#7739=VERTEX_POINT('',#36459);
#7740=VERTEX_POINT('',#36460);
#7741=VERTEX_POINT('',#36463);
#7742=VERTEX_POINT('',#36465);
#7743=VERTEX_POINT('',#36471);
#7744=VERTEX_POINT('',#36472);
#7745=VERTEX_POINT('',#36477);
#7746=VERTEX_POINT('',#36478);
#7747=VERTEX_POINT('',#36481);
#7748=VERTEX_POINT('',#36483);
#7749=VERTEX_POINT('',#36489);
#7750=VERTEX_POINT('',#36490);
#7751=VERTEX_POINT('',#36495);
#7752=VERTEX_POINT('',#36496);
#7753=VERTEX_POINT('',#36499);
#7754=VERTEX_POINT('',#36501);
#7755=VERTEX_POINT('',#36507);
#7756=VERTEX_POINT('',#36508);
#7757=VERTEX_POINT('',#36513);
#7758=VERTEX_POINT('',#36514);
#7759=VERTEX_POINT('',#36517);
#7760=VERTEX_POINT('',#36519);
#7761=VERTEX_POINT('',#36525);
#7762=VERTEX_POINT('',#36526);
#7763=VERTEX_POINT('',#36531);
#7764=VERTEX_POINT('',#36532);
#7765=VERTEX_POINT('',#36535);
#7766=VERTEX_POINT('',#36537);
#7767=VERTEX_POINT('',#36543);
#7768=VERTEX_POINT('',#36544);
#7769=VERTEX_POINT('',#36549);
#7770=VERTEX_POINT('',#36550);
#7771=VERTEX_POINT('',#36553);
#7772=VERTEX_POINT('',#36555);
#7773=VERTEX_POINT('',#36561);
#7774=VERTEX_POINT('',#36565);
#7775=VERTEX_POINT('',#36566);
#7776=VERTEX_POINT('',#36570);
#7777=VERTEX_POINT('',#36572);
#7778=VERTEX_POINT('',#36576);
#7779=VERTEX_POINT('',#36580);
#7780=VERTEX_POINT('',#36582);
#7781=VERTEX_POINT('',#36586);
#7782=VERTEX_POINT('',#36590);
#7783=VERTEX_POINT('',#36592);
#7784=VERTEX_POINT('',#36596);
#7785=VERTEX_POINT('',#36600);
#7786=VERTEX_POINT('',#36602);
#7787=VERTEX_POINT('',#36606);
#7788=VERTEX_POINT('',#36610);
#7789=VERTEX_POINT('',#36612);
#7790=VERTEX_POINT('',#36616);
#7791=VERTEX_POINT('',#36620);
#7792=VERTEX_POINT('',#36622);
#7793=VERTEX_POINT('',#36626);
#7794=VERTEX_POINT('',#36630);
#7795=VERTEX_POINT('',#36632);
#7796=VERTEX_POINT('',#36636);
#7797=VERTEX_POINT('',#36640);
#7798=VERTEX_POINT('',#36642);
#7799=VERTEX_POINT('',#36646);
#7800=VERTEX_POINT('',#36650);
#7801=VERTEX_POINT('',#36652);
#7802=VERTEX_POINT('',#36656);
#7803=VERTEX_POINT('',#36660);
#7804=VERTEX_POINT('',#36662);
#7805=VERTEX_POINT('',#36666);
#7806=VERTEX_POINT('',#36670);
#7807=VERTEX_POINT('',#36672);
#7808=VERTEX_POINT('',#36676);
#7809=VERTEX_POINT('',#36680);
#7810=VERTEX_POINT('',#36682);
#7811=VERTEX_POINT('',#36686);
#7812=VERTEX_POINT('',#36690);
#7813=VERTEX_POINT('',#36692);
#7814=VERTEX_POINT('',#36696);
#7815=VERTEX_POINT('',#36700);
#7816=VERTEX_POINT('',#36702);
#7817=VERTEX_POINT('',#36706);
#7818=VERTEX_POINT('',#36710);
#7819=VERTEX_POINT('',#36712);
#7820=VERTEX_POINT('',#36716);
#7821=VERTEX_POINT('',#36720);
#7822=VERTEX_POINT('',#36722);
#7823=VERTEX_POINT('',#36726);
#7824=VERTEX_POINT('',#36730);
#7825=VERTEX_POINT('',#36732);
#7826=VERTEX_POINT('',#36736);
#7827=VERTEX_POINT('',#36740);
#7828=VERTEX_POINT('',#36742);
#7829=VERTEX_POINT('',#36746);
#7830=VERTEX_POINT('',#36750);
#7831=VERTEX_POINT('',#36752);
#7832=VERTEX_POINT('',#36756);
#7833=VERTEX_POINT('',#36760);
#7834=VERTEX_POINT('',#36762);
#7835=VERTEX_POINT('',#36766);
#7836=VERTEX_POINT('',#36770);
#7837=VERTEX_POINT('',#36772);
#7838=VERTEX_POINT('',#36776);
#7839=VERTEX_POINT('',#36780);
#7840=VERTEX_POINT('',#36782);
#7841=VERTEX_POINT('',#36786);
#7842=VERTEX_POINT('',#36790);
#7843=VERTEX_POINT('',#36792);
#7844=VERTEX_POINT('',#36796);
#7845=VERTEX_POINT('',#36800);
#7846=VERTEX_POINT('',#36802);
#7847=VERTEX_POINT('',#36806);
#7848=VERTEX_POINT('',#36810);
#7849=VERTEX_POINT('',#36812);
#7850=VERTEX_POINT('',#36816);
#7851=VERTEX_POINT('',#36820);
#7852=VERTEX_POINT('',#36822);
#7853=VERTEX_POINT('',#36826);
#7854=VERTEX_POINT('',#36830);
#7855=VERTEX_POINT('',#36832);
#7856=VERTEX_POINT('',#36836);
#7857=VERTEX_POINT('',#36840);
#7858=VERTEX_POINT('',#36842);
#7859=VERTEX_POINT('',#36846);
#7860=VERTEX_POINT('',#36850);
#7861=VERTEX_POINT('',#36852);
#7862=VERTEX_POINT('',#36856);
#7863=VERTEX_POINT('',#36860);
#7864=VERTEX_POINT('',#36862);
#7865=VERTEX_POINT('',#36866);
#7866=VERTEX_POINT('',#36870);
#7867=VERTEX_POINT('',#36872);
#7868=VERTEX_POINT('',#36876);
#7869=VERTEX_POINT('',#36880);
#7870=VERTEX_POINT('',#36882);
#7871=VERTEX_POINT('',#36886);
#7872=VERTEX_POINT('',#36890);
#7873=VERTEX_POINT('',#36892);
#7874=VERTEX_POINT('',#36896);
#7875=VERTEX_POINT('',#36900);
#7876=VERTEX_POINT('',#36902);
#7877=VERTEX_POINT('',#36906);
#7878=VERTEX_POINT('',#36910);
#7879=VERTEX_POINT('',#36912);
#7880=VERTEX_POINT('',#36916);
#7881=VERTEX_POINT('',#36920);
#7882=VERTEX_POINT('',#36922);
#7883=VERTEX_POINT('',#36926);
#7884=VERTEX_POINT('',#36930);
#7885=VERTEX_POINT('',#36932);
#7886=VERTEX_POINT('',#36936);
#7887=VERTEX_POINT('',#36940);
#7888=VERTEX_POINT('',#36942);
#7889=VERTEX_POINT('',#36946);
#7890=VERTEX_POINT('',#36950);
#7891=VERTEX_POINT('',#36952);
#7892=VERTEX_POINT('',#36956);
#7893=VERTEX_POINT('',#36959);
#7894=VERTEX_POINT('',#36963);
#7895=VERTEX_POINT('',#36967);
#7896=VERTEX_POINT('',#36969);
#7897=VERTEX_POINT('',#36973);
#7898=VERTEX_POINT('',#36977);
#7899=VERTEX_POINT('',#36979);
#7900=VERTEX_POINT('',#36983);
#7901=VERTEX_POINT('',#36987);
#7902=VERTEX_POINT('',#36989);
#7903=VERTEX_POINT('',#36993);
#7904=VERTEX_POINT('',#36997);
#7905=VERTEX_POINT('',#36999);
#7906=VERTEX_POINT('',#37003);
#7907=VERTEX_POINT('',#37007);
#7908=VERTEX_POINT('',#37009);
#7909=VERTEX_POINT('',#37013);
#7910=VERTEX_POINT('',#37017);
#7911=VERTEX_POINT('',#37019);
#7912=VERTEX_POINT('',#37023);
#7913=VERTEX_POINT('',#37027);
#7914=VERTEX_POINT('',#37029);
#7915=VERTEX_POINT('',#37033);
#7916=VERTEX_POINT('',#37037);
#7917=VERTEX_POINT('',#37039);
#7918=VERTEX_POINT('',#37043);
#7919=VERTEX_POINT('',#37047);
#7920=VERTEX_POINT('',#37049);
#7921=VERTEX_POINT('',#37053);
#7922=VERTEX_POINT('',#37057);
#7923=VERTEX_POINT('',#37059);
#7924=VERTEX_POINT('',#37063);
#7925=VERTEX_POINT('',#37067);
#7926=VERTEX_POINT('',#37069);
#7927=VERTEX_POINT('',#37073);
#7928=VERTEX_POINT('',#37077);
#7929=VERTEX_POINT('',#37079);
#7930=VERTEX_POINT('',#37083);
#7931=VERTEX_POINT('',#37087);
#7932=VERTEX_POINT('',#37089);
#7933=VERTEX_POINT('',#37093);
#7934=VERTEX_POINT('',#37097);
#7935=VERTEX_POINT('',#37099);
#7936=VERTEX_POINT('',#37103);
#7937=VERTEX_POINT('',#37107);
#7938=VERTEX_POINT('',#37109);
#7939=VERTEX_POINT('',#37113);
#7940=VERTEX_POINT('',#37117);
#7941=VERTEX_POINT('',#37119);
#7942=VERTEX_POINT('',#37123);
#7943=VERTEX_POINT('',#37127);
#7944=VERTEX_POINT('',#37129);
#7945=VERTEX_POINT('',#37133);
#7946=VERTEX_POINT('',#37137);
#7947=VERTEX_POINT('',#37139);
#7948=VERTEX_POINT('',#37143);
#7949=VERTEX_POINT('',#37147);
#7950=VERTEX_POINT('',#37149);
#7951=VERTEX_POINT('',#37153);
#7952=VERTEX_POINT('',#37157);
#7953=VERTEX_POINT('',#37159);
#7954=VERTEX_POINT('',#37163);
#7955=VERTEX_POINT('',#37167);
#7956=VERTEX_POINT('',#37169);
#7957=VERTEX_POINT('',#37173);
#7958=VERTEX_POINT('',#37177);
#7959=VERTEX_POINT('',#37179);
#7960=VERTEX_POINT('',#37183);
#7961=VERTEX_POINT('',#37187);
#7962=VERTEX_POINT('',#37189);
#7963=VERTEX_POINT('',#37193);
#7964=VERTEX_POINT('',#37197);
#7965=VERTEX_POINT('',#37199);
#7966=VERTEX_POINT('',#37203);
#7967=VERTEX_POINT('',#37207);
#7968=VERTEX_POINT('',#37209);
#7969=VERTEX_POINT('',#37213);
#7970=VERTEX_POINT('',#37217);
#7971=VERTEX_POINT('',#37219);
#7972=VERTEX_POINT('',#37223);
#7973=VERTEX_POINT('',#37227);
#7974=VERTEX_POINT('',#37229);
#7975=VERTEX_POINT('',#37233);
#7976=VERTEX_POINT('',#37237);
#7977=VERTEX_POINT('',#37239);
#7978=VERTEX_POINT('',#37243);
#7979=VERTEX_POINT('',#37247);
#7980=VERTEX_POINT('',#37249);
#7981=VERTEX_POINT('',#37253);
#7982=VERTEX_POINT('',#37257);
#7983=VERTEX_POINT('',#37259);
#7984=VERTEX_POINT('',#37263);
#7985=VERTEX_POINT('',#37267);
#7986=VERTEX_POINT('',#37269);
#7987=VERTEX_POINT('',#37273);
#7988=VERTEX_POINT('',#37277);
#7989=VERTEX_POINT('',#37279);
#7990=VERTEX_POINT('',#37283);
#7991=VERTEX_POINT('',#37287);
#7992=VERTEX_POINT('',#37289);
#7993=VERTEX_POINT('',#37293);
#7994=VERTEX_POINT('',#37297);
#7995=VERTEX_POINT('',#37299);
#7996=VERTEX_POINT('',#37303);
#7997=VERTEX_POINT('',#37307);
#7998=VERTEX_POINT('',#37309);
#7999=VERTEX_POINT('',#37313);
#8000=VERTEX_POINT('',#37317);
#8001=VERTEX_POINT('',#37319);
#8002=VERTEX_POINT('',#37323);
#8003=VERTEX_POINT('',#37327);
#8004=VERTEX_POINT('',#37329);
#8005=VERTEX_POINT('',#37333);
#8006=VERTEX_POINT('',#37337);
#8007=VERTEX_POINT('',#37343);
#8008=VERTEX_POINT('',#37344);
#8009=VERTEX_POINT('',#37348);
#8010=VERTEX_POINT('',#37350);
#8011=VERTEX_POINT('',#37354);
#8012=VERTEX_POINT('',#37358);
#8013=VERTEX_POINT('',#37360);
#8014=VERTEX_POINT('',#37364);
#8015=VERTEX_POINT('',#37368);
#8016=VERTEX_POINT('',#37370);
#8017=VERTEX_POINT('',#37374);
#8018=VERTEX_POINT('',#37378);
#8019=VERTEX_POINT('',#37380);
#8020=VERTEX_POINT('',#37384);
#8021=VERTEX_POINT('',#37388);
#8022=VERTEX_POINT('',#37390);
#8023=VERTEX_POINT('',#37394);
#8024=VERTEX_POINT('',#37398);
#8025=VERTEX_POINT('',#37400);
#8026=VERTEX_POINT('',#37404);
#8027=VERTEX_POINT('',#37408);
#8028=VERTEX_POINT('',#37410);
#8029=VERTEX_POINT('',#37414);
#8030=VERTEX_POINT('',#37418);
#8031=VERTEX_POINT('',#37420);
#8032=VERTEX_POINT('',#37424);
#8033=VERTEX_POINT('',#37428);
#8034=VERTEX_POINT('',#37430);
#8035=VERTEX_POINT('',#37434);
#8036=VERTEX_POINT('',#37438);
#8037=VERTEX_POINT('',#37440);
#8038=VERTEX_POINT('',#37444);
#8039=VERTEX_POINT('',#37448);
#8040=VERTEX_POINT('',#37450);
#8041=VERTEX_POINT('',#37454);
#8042=VERTEX_POINT('',#37458);
#8043=VERTEX_POINT('',#37460);
#8044=VERTEX_POINT('',#37464);
#8045=VERTEX_POINT('',#37468);
#8046=VERTEX_POINT('',#37470);
#8047=VERTEX_POINT('',#37474);
#8048=VERTEX_POINT('',#37478);
#8049=VERTEX_POINT('',#37480);
#8050=VERTEX_POINT('',#37484);
#8051=VERTEX_POINT('',#37488);
#8052=VERTEX_POINT('',#37490);
#8053=VERTEX_POINT('',#37494);
#8054=VERTEX_POINT('',#37498);
#8055=VERTEX_POINT('',#37500);
#8056=VERTEX_POINT('',#37504);
#8057=VERTEX_POINT('',#37508);
#8058=VERTEX_POINT('',#37510);
#8059=VERTEX_POINT('',#37514);
#8060=VERTEX_POINT('',#37518);
#8061=VERTEX_POINT('',#37520);
#8062=VERTEX_POINT('',#37524);
#8063=VERTEX_POINT('',#37528);
#8064=VERTEX_POINT('',#37530);
#8065=VERTEX_POINT('',#37534);
#8066=VERTEX_POINT('',#37538);
#8067=VERTEX_POINT('',#37540);
#8068=VERTEX_POINT('',#37544);
#8069=VERTEX_POINT('',#37548);
#8070=VERTEX_POINT('',#37550);
#8071=VERTEX_POINT('',#37554);
#8072=VERTEX_POINT('',#37558);
#8073=VERTEX_POINT('',#37560);
#8074=VERTEX_POINT('',#37564);
#8075=VERTEX_POINT('',#37568);
#8076=VERTEX_POINT('',#37570);
#8077=VERTEX_POINT('',#37574);
#8078=VERTEX_POINT('',#37578);
#8079=VERTEX_POINT('',#37580);
#8080=VERTEX_POINT('',#37584);
#8081=VERTEX_POINT('',#37588);
#8082=VERTEX_POINT('',#37590);
#8083=VERTEX_POINT('',#37594);
#8084=VERTEX_POINT('',#37598);
#8085=VERTEX_POINT('',#37600);
#8086=VERTEX_POINT('',#37604);
#8087=VERTEX_POINT('',#37608);
#8088=VERTEX_POINT('',#37610);
#8089=VERTEX_POINT('',#37614);
#8090=VERTEX_POINT('',#37618);
#8091=VERTEX_POINT('',#37620);
#8092=VERTEX_POINT('',#37624);
#8093=VERTEX_POINT('',#37628);
#8094=VERTEX_POINT('',#37630);
#8095=VERTEX_POINT('',#37634);
#8096=VERTEX_POINT('',#37638);
#8097=VERTEX_POINT('',#37640);
#8098=VERTEX_POINT('',#37644);
#8099=VERTEX_POINT('',#37648);
#8100=VERTEX_POINT('',#37650);
#8101=VERTEX_POINT('',#37654);
#8102=VERTEX_POINT('',#37658);
#8103=VERTEX_POINT('',#37660);
#8104=VERTEX_POINT('',#37664);
#8105=VERTEX_POINT('',#37668);
#8106=VERTEX_POINT('',#37670);
#8107=VERTEX_POINT('',#37674);
#8108=VERTEX_POINT('',#37678);
#8109=VERTEX_POINT('',#37680);
#8110=VERTEX_POINT('',#37684);
#8111=VERTEX_POINT('',#37688);
#8112=VERTEX_POINT('',#37690);
#8113=VERTEX_POINT('',#37694);
#8114=VERTEX_POINT('',#37698);
#8115=VERTEX_POINT('',#37700);
#8116=VERTEX_POINT('',#37704);
#8117=VERTEX_POINT('',#37708);
#8118=VERTEX_POINT('',#37710);
#8119=VERTEX_POINT('',#37714);
#8120=VERTEX_POINT('',#37718);
#8121=VERTEX_POINT('',#37720);
#8122=VERTEX_POINT('',#37724);
#8123=VERTEX_POINT('',#37728);
#8124=VERTEX_POINT('',#37730);
#8125=VERTEX_POINT('',#37734);
#8126=VERTEX_POINT('',#37737);
#8127=VERTEX_POINT('',#37741);
#8128=VERTEX_POINT('',#37745);
#8129=VERTEX_POINT('',#37747);
#8130=VERTEX_POINT('',#37751);
#8131=VERTEX_POINT('',#37755);
#8132=VERTEX_POINT('',#37757);
#8133=VERTEX_POINT('',#37761);
#8134=VERTEX_POINT('',#37765);
#8135=VERTEX_POINT('',#37767);
#8136=VERTEX_POINT('',#37771);
#8137=VERTEX_POINT('',#37775);
#8138=VERTEX_POINT('',#37777);
#8139=VERTEX_POINT('',#37781);
#8140=VERTEX_POINT('',#37785);
#8141=VERTEX_POINT('',#37787);
#8142=VERTEX_POINT('',#37791);
#8143=VERTEX_POINT('',#37795);
#8144=VERTEX_POINT('',#37797);
#8145=VERTEX_POINT('',#37801);
#8146=VERTEX_POINT('',#37805);
#8147=VERTEX_POINT('',#37807);
#8148=VERTEX_POINT('',#37811);
#8149=VERTEX_POINT('',#37815);
#8150=VERTEX_POINT('',#37817);
#8151=VERTEX_POINT('',#37821);
#8152=VERTEX_POINT('',#37825);
#8153=VERTEX_POINT('',#37827);
#8154=VERTEX_POINT('',#37831);
#8155=VERTEX_POINT('',#37835);
#8156=VERTEX_POINT('',#37837);
#8157=VERTEX_POINT('',#37841);
#8158=VERTEX_POINT('',#37845);
#8159=VERTEX_POINT('',#37847);
#8160=VERTEX_POINT('',#37851);
#8161=VERTEX_POINT('',#37855);
#8162=VERTEX_POINT('',#37857);
#8163=VERTEX_POINT('',#37861);
#8164=VERTEX_POINT('',#37865);
#8165=VERTEX_POINT('',#37867);
#8166=VERTEX_POINT('',#37871);
#8167=VERTEX_POINT('',#37875);
#8168=VERTEX_POINT('',#37877);
#8169=VERTEX_POINT('',#37881);
#8170=VERTEX_POINT('',#37885);
#8171=VERTEX_POINT('',#37887);
#8172=VERTEX_POINT('',#37891);
#8173=VERTEX_POINT('',#37895);
#8174=VERTEX_POINT('',#37897);
#8175=VERTEX_POINT('',#37901);
#8176=VERTEX_POINT('',#37905);
#8177=VERTEX_POINT('',#37907);
#8178=VERTEX_POINT('',#37911);
#8179=VERTEX_POINT('',#37915);
#8180=VERTEX_POINT('',#37917);
#8181=VERTEX_POINT('',#37921);
#8182=VERTEX_POINT('',#37925);
#8183=VERTEX_POINT('',#37927);
#8184=VERTEX_POINT('',#37931);
#8185=VERTEX_POINT('',#37935);
#8186=VERTEX_POINT('',#37937);
#8187=VERTEX_POINT('',#37941);
#8188=VERTEX_POINT('',#37945);
#8189=VERTEX_POINT('',#37947);
#8190=VERTEX_POINT('',#37951);
#8191=VERTEX_POINT('',#37955);
#8192=VERTEX_POINT('',#37957);
#8193=VERTEX_POINT('',#37961);
#8194=VERTEX_POINT('',#37965);
#8195=VERTEX_POINT('',#37967);
#8196=VERTEX_POINT('',#37971);
#8197=VERTEX_POINT('',#37975);
#8198=VERTEX_POINT('',#37977);
#8199=VERTEX_POINT('',#37981);
#8200=VERTEX_POINT('',#37985);
#8201=VERTEX_POINT('',#37987);
#8202=VERTEX_POINT('',#37991);
#8203=VERTEX_POINT('',#37995);
#8204=VERTEX_POINT('',#37997);
#8205=VERTEX_POINT('',#38001);
#8206=VERTEX_POINT('',#38005);
#8207=VERTEX_POINT('',#38007);
#8208=VERTEX_POINT('',#38011);
#8209=VERTEX_POINT('',#38015);
#8210=VERTEX_POINT('',#38017);
#8211=VERTEX_POINT('',#38021);
#8212=VERTEX_POINT('',#38025);
#8213=VERTEX_POINT('',#38027);
#8214=VERTEX_POINT('',#38031);
#8215=VERTEX_POINT('',#38035);
#8216=VERTEX_POINT('',#38037);
#8217=VERTEX_POINT('',#38041);
#8218=VERTEX_POINT('',#38045);
#8219=VERTEX_POINT('',#38047);
#8220=VERTEX_POINT('',#38051);
#8221=VERTEX_POINT('',#38055);
#8222=VERTEX_POINT('',#38057);
#8223=VERTEX_POINT('',#38061);
#8224=VERTEX_POINT('',#38065);
#8225=VERTEX_POINT('',#38067);
#8226=VERTEX_POINT('',#38071);
#8227=VERTEX_POINT('',#38075);
#8228=VERTEX_POINT('',#38077);
#8229=VERTEX_POINT('',#38081);
#8230=VERTEX_POINT('',#38085);
#8231=VERTEX_POINT('',#38087);
#8232=VERTEX_POINT('',#38091);
#8233=VERTEX_POINT('',#38095);
#8234=VERTEX_POINT('',#38097);
#8235=VERTEX_POINT('',#38101);
#8236=VERTEX_POINT('',#38105);
#8237=VERTEX_POINT('',#38107);
#8238=VERTEX_POINT('',#38111);
#8239=VERTEX_POINT('',#38115);
#8240=VERTEX_POINT('',#38121);
#8971=EDGE_CURVE('',#6961,#6961,#5919,.T.);
#8972=EDGE_CURVE('',#6961,#6962,#3944,.T.);
#8973=EDGE_CURVE('',#6962,#6962,#5920,.T.);
#8974=EDGE_CURVE('',#6963,#6964,#5921,.T.);
#8975=EDGE_CURVE('',#6964,#6963,#5922,.T.);
#8976=EDGE_CURVE('',#6964,#6965,#3945,.T.);
#8977=EDGE_CURVE('',#6965,#6965,#5923,.T.);
#8978=EDGE_CURVE('',#6966,#6967,#5924,.T.);
#8979=EDGE_CURVE('',#6967,#6966,#5925,.T.);
#8980=EDGE_CURVE('',#6967,#6968,#3946,.T.);
#8981=EDGE_CURVE('',#6968,#6968,#5926,.T.);
#8982=EDGE_CURVE('',#6969,#6969,#5927,.T.);
#8983=EDGE_CURVE('',#6969,#6970,#3947,.T.);
#8984=EDGE_CURVE('',#6970,#6970,#5928,.T.);
#8985=EDGE_CURVE('',#6971,#6972,#5929,.T.);
#8986=EDGE_CURVE('',#6973,#6971,#238,.T.);
#8987=EDGE_CURVE('',#6974,#6973,#5930,.T.);
#8988=EDGE_CURVE('',#6972,#6974,#239,.T.);
#8989=EDGE_CURVE('',#6975,#6976,#5931,.T.);
#8990=EDGE_CURVE('',#6976,#6975,#5932,.T.);
#8991=EDGE_CURVE('',#6976,#6977,#3948,.T.);
#8992=EDGE_CURVE('',#6977,#6977,#5933,.T.);
#8993=EDGE_CURVE('',#6978,#6979,#5934,.T.);
#8994=EDGE_CURVE('',#6979,#6978,#5935,.T.);
#8995=EDGE_CURVE('',#6979,#6980,#3949,.T.);
#8996=EDGE_CURVE('',#6980,#6980,#5936,.T.);
#8997=EDGE_CURVE('',#6981,#6981,#5937,.T.);
#8998=EDGE_CURVE('',#6981,#6982,#3950,.T.);
#8999=EDGE_CURVE('',#6982,#6982,#5938,.T.);
#9000=EDGE_CURVE('',#6983,#6983,#5939,.T.);
#9001=EDGE_CURVE('',#6983,#6984,#3951,.T.);
#9002=EDGE_CURVE('',#6984,#6984,#5940,.T.);
#9003=EDGE_CURVE('',#6985,#6986,#5941,.T.);
#9004=EDGE_CURVE('',#6987,#6985,#240,.T.);
#9005=EDGE_CURVE('',#6988,#6987,#5942,.T.);
#9006=EDGE_CURVE('',#6986,#6988,#241,.T.);
#9007=EDGE_CURVE('',#6978,#6989,#3952,.T.);
#9008=EDGE_CURVE('',#6990,#6989,#5943,.T.);
#9009=EDGE_CURVE('',#6991,#6990,#1005,.F.);
#9010=EDGE_CURVE('',#6989,#6991,#5944,.T.);
#9011=EDGE_CURVE('',#6992,#6992,#5945,.T.);
#9012=EDGE_CURVE('',#6992,#6961,#3953,.T.);
#9013=EDGE_CURVE('',#6975,#6969,#3954,.T.);
#9014=EDGE_CURVE('',#6972,#6985,#3955,.T.);
#9015=EDGE_CURVE('',#6991,#6986,#3956,.T.);
#9016=EDGE_CURVE('',#6971,#6990,#3957,.T.);
#9017=EDGE_CURVE('',#6966,#6981,#3958,.T.);
#9018=EDGE_CURVE('',#6963,#6983,#3959,.T.);
#9019=EDGE_CURVE('',#6993,#6994,#3960,.T.);
#9020=EDGE_CURVE('',#6993,#6995,#3961,.T.);
#9021=EDGE_CURVE('',#6995,#6996,#3962,.T.);
#9022=EDGE_CURVE('',#6994,#6996,#3963,.T.);
#9023=EDGE_CURVE('',#6997,#6998,#3964,.T.);
#9024=EDGE_CURVE('',#6998,#6999,#3965,.T.);
#9025=EDGE_CURVE('',#6999,#7000,#3966,.T.);
#9026=EDGE_CURVE('',#7000,#6997,#3967,.T.);
#9027=EDGE_CURVE('',#7001,#6987,#3968,.T.);
#9028=EDGE_CURVE('',#7001,#7002,#5946,.T.);
#9029=EDGE_CURVE('',#7003,#7002,#3969,.T.);
#9030=EDGE_CURVE('',#7004,#7003,#3970,.T.);
#9031=EDGE_CURVE('',#6996,#7004,#3971,.T.);
#9032=EDGE_CURVE('',#6995,#7005,#3972,.T.);
#9033=EDGE_CURVE('',#7005,#7006,#3973,.T.);
#9034=EDGE_CURVE('',#7006,#7007,#3974,.T.);
#9035=EDGE_CURVE('',#7008,#7007,#3975,.T.);
#9036=EDGE_CURVE('',#7009,#7008,#3976,.T.);
#9037=EDGE_CURVE('',#7010,#7009,#3977,.T.);
#9038=EDGE_CURVE('',#7011,#7010,#3978,.T.);
#9039=EDGE_CURVE('',#7011,#7012,#5947,.T.);
#9040=EDGE_CURVE('',#6988,#7012,#3979,.T.);
#9041=EDGE_CURVE('',#7007,#7013,#3980,.T.);
#9042=EDGE_CURVE('',#7014,#7013,#3981,.T.);
#9043=EDGE_CURVE('',#7014,#7008,#3982,.T.);
#9044=EDGE_CURVE('',#7015,#6974,#3983,.T.);
#9045=EDGE_CURVE('',#6973,#7016,#3984,.T.);
#9046=EDGE_CURVE('',#7016,#7017,#5948,.T.);
#9047=EDGE_CURVE('',#7017,#7018,#3985,.T.);
#9048=EDGE_CURVE('',#7018,#7019,#3986,.T.);
#9049=EDGE_CURVE('',#7019,#7014,#3987,.T.);
#9050=EDGE_CURVE('',#7013,#7020,#3988,.T.);
#9051=EDGE_CURVE('',#7020,#7021,#3989,.T.);
#9052=EDGE_CURVE('',#7021,#7022,#3990,.T.);
#9053=EDGE_CURVE('',#7022,#7023,#3991,.T.);
#9054=EDGE_CURVE('',#7023,#7024,#3992,.T.);
#9055=EDGE_CURVE('',#7024,#7025,#3993,.T.);
#9056=EDGE_CURVE('',#7025,#6993,#3994,.T.);
#9057=EDGE_CURVE('',#6994,#7026,#3995,.T.);
#9058=EDGE_CURVE('',#7026,#7027,#3996,.T.);
#9059=EDGE_CURVE('',#7027,#7028,#3997,.T.);
#9060=EDGE_CURVE('',#7028,#7015,#5949,.T.);
#9061=EDGE_CURVE('',#7029,#7030,#3998,.T.);
#9062=EDGE_CURVE('',#7030,#7031,#3999,.T.);
#9063=EDGE_CURVE('',#7031,#7032,#4000,.T.);
#9064=EDGE_CURVE('',#7029,#7032,#4001,.T.);
#9065=EDGE_CURVE('',#7033,#7034,#4002,.T.);
#9066=EDGE_CURVE('',#7034,#7035,#4003,.T.);
#9067=EDGE_CURVE('',#7035,#7036,#4004,.T.);
#9068=EDGE_CURVE('',#7036,#7037,#4005,.T.);
#9069=EDGE_CURVE('',#7038,#7037,#4006,.T.);
#9070=EDGE_CURVE('',#7029,#7038,#4007,.T.);
#9071=EDGE_CURVE('',#7032,#7033,#4008,.T.);
#9072=EDGE_CURVE('',#7039,#7040,#4009,.T.);
#9073=EDGE_CURVE('',#7040,#7041,#4010,.T.);
#9074=EDGE_CURVE('',#7041,#7042,#4011,.T.);
#9075=EDGE_CURVE('',#7042,#7043,#4012,.T.);
#9076=EDGE_CURVE('',#7043,#7044,#5950,.T.);
#9077=EDGE_CURVE('',#7044,#7045,#4013,.T.);
#9078=EDGE_CURVE('',#7045,#7039,#4014,.T.);
#9079=EDGE_CURVE('',#7046,#7047,#4015,.T.);
#9080=EDGE_CURVE('',#7047,#7048,#4016,.T.);
#9081=EDGE_CURVE('',#7048,#7049,#4017,.T.);
#9082=EDGE_CURVE('',#7049,#7050,#4018,.T.);
#9083=EDGE_CURVE('',#7050,#7051,#5951,.T.);
#9084=EDGE_CURVE('',#7051,#7052,#4019,.T.);
#9085=EDGE_CURVE('',#7052,#7053,#4020,.T.);
#9086=EDGE_CURVE('',#7053,#7054,#4021,.T.);
#9087=EDGE_CURVE('',#7054,#7046,#4022,.T.);
#9088=EDGE_CURVE('',#7055,#7056,#4023,.T.);
#9089=EDGE_CURVE('',#7056,#7057,#5952,.T.);
#9090=EDGE_CURVE('',#7058,#7057,#4024,.T.);
#9091=EDGE_CURVE('',#7058,#7055,#5953,.T.);
#9092=EDGE_CURVE('',#7012,#7056,#1006,.T.);
#9093=EDGE_CURVE('',#7055,#7016,#1007,.T.);
#9094=EDGE_CURVE('',#7059,#7060,#4025,.T.);
#9095=EDGE_CURVE('',#7060,#7001,#1008,.T.);
#9096=EDGE_CURVE('',#7015,#7059,#1009,.T.);
#9097=EDGE_CURVE('',#7061,#7062,#4026,.T.);
#9098=EDGE_CURVE('',#7062,#7060,#5954,.T.);
#9099=EDGE_CURVE('',#7059,#7061,#5955,.T.);
#9100=EDGE_CURVE('',#7002,#7062,#1010,.T.);
#9101=EDGE_CURVE('',#7061,#7028,#1011,.T.);
#9102=EDGE_CURVE('',#7027,#7003,#4027,.T.);
#9103=EDGE_CURVE('',#7026,#7004,#4028,.T.);
#9104=EDGE_CURVE('',#7019,#7009,#4029,.T.);
#9105=EDGE_CURVE('',#7018,#7010,#4030,.T.);
#9106=EDGE_CURVE('',#7057,#7011,#1012,.T.);
#9107=EDGE_CURVE('',#7017,#7058,#1013,.T.);
#9108=EDGE_CURVE('',#7031,#7063,#4031,.T.);
#9109=EDGE_CURVE('',#7063,#7064,#4032,.T.);
#9110=EDGE_CURVE('',#7064,#7065,#5956,.T.);
#9111=EDGE_CURVE('',#7065,#7066,#4033,.T.);
#9112=EDGE_CURVE('',#7066,#7033,#4034,.T.);
#9113=EDGE_CURVE('',#7066,#7067,#4035,.T.);
#9114=EDGE_CURVE('',#7067,#7034,#4036,.T.);
#9115=EDGE_CURVE('',#7063,#7068,#4037,.T.);
#9116=EDGE_CURVE('',#7068,#7069,#4038,.T.);
#9117=EDGE_CURVE('',#7064,#7069,#4039,.T.);
#9118=EDGE_CURVE('',#7065,#7070,#4040,.T.);
#9119=EDGE_CURVE('',#7070,#7067,#4041,.T.);
#9120=EDGE_CURVE('',#7069,#7070,#5957,.T.);
#9121=EDGE_CURVE('',#7071,#7072,#4042,.T.);
#9122=EDGE_CURVE('',#7072,#7030,#4043,.T.);
#9123=EDGE_CURVE('',#7038,#7071,#5958,.T.);
#9124=EDGE_CURVE('',#7073,#7074,#4044,.T.);
#9125=EDGE_CURVE('',#7074,#7072,#4045,.T.);
#9126=EDGE_CURVE('',#7071,#7073,#4046,.T.);
#9127=EDGE_CURVE('',#7037,#7073,#5959,.T.);
#9128=EDGE_CURVE('',#7025,#7042,#5960,.T.);
#9129=EDGE_CURVE('',#6993,#7041,#68,.T.);
#9130=EDGE_CURVE('',#6995,#7040,#69,.T.);
#9131=EDGE_CURVE('',#7042,#7074,#5961,.T.);
#9132=EDGE_CURVE('',#7043,#7073,#5962,.T.);
#9133=EDGE_CURVE('',#7005,#7039,#5963,.T.);
#9134=EDGE_CURVE('',#7052,#7020,#5964,.T.);
#9135=EDGE_CURVE('',#7053,#7013,#70,.T.);
#9136=EDGE_CURVE('',#7044,#7037,#5965,.T.);
#9137=EDGE_CURVE('',#7005,#6997,#5966,.T.);
#9138=EDGE_CURVE('',#6997,#7039,#5967,.T.);
#9139=EDGE_CURVE('',#7054,#7007,#71,.T.);
#9140=EDGE_CURVE('',#7068,#7052,#5968,.T.);
#9141=EDGE_CURVE('',#7069,#7051,#5969,.T.);
#9142=EDGE_CURVE('',#7045,#7036,#5970,.T.);
#9143=EDGE_CURVE('',#6998,#7045,#5971,.T.);
#9144=EDGE_CURVE('',#7006,#7000,#5972,.T.);
#9145=EDGE_CURVE('',#7046,#7006,#5973,.T.);
#9146=EDGE_CURVE('',#7070,#7050,#5974,.T.);
#9147=EDGE_CURVE('',#6998,#7036,#5975,.T.);
#9148=EDGE_CURVE('',#7046,#7000,#5976,.T.);
#9149=EDGE_CURVE('',#7067,#7049,#72,.T.);
#9150=EDGE_CURVE('',#6999,#7035,#5977,.T.);
#9151=EDGE_CURVE('',#7047,#6999,#5978,.T.);
#9152=EDGE_CURVE('',#7034,#7048,#73,.T.);
#9153=EDGE_CURVE('',#7047,#7035,#5979,.T.);
#9154=EDGE_CURVE('',#7074,#7025,#5980,.T.);
#9155=EDGE_CURVE('',#7072,#7024,#74,.T.);
#9156=EDGE_CURVE('',#7030,#7023,#75,.T.);
#9157=EDGE_CURVE('',#7031,#7022,#76,.T.);
#9158=EDGE_CURVE('',#7063,#7021,#77,.T.);
#9159=EDGE_CURVE('',#7068,#7020,#5981,.T.);
#9160=EDGE_CURVE('',#7075,#7075,#5982,.T.);
#9161=EDGE_CURVE('',#7075,#7076,#5983,.T.);
#9162=EDGE_CURVE('',#7077,#7076,#5984,.T.);
#9163=EDGE_CURVE('',#7076,#7077,#5985,.T.);
#9164=EDGE_CURVE('',#7078,#7079,#5986,.T.);
#9165=EDGE_CURVE('',#7079,#7078,#5987,.T.);
#9166=EDGE_CURVE('',#7079,#7080,#5988,.T.);
#9167=EDGE_CURVE('',#7080,#7080,#5989,.T.);
#9168=EDGE_CURVE('',#7078,#7077,#4047,.T.);
#9169=EDGE_CURVE('',#7081,#7081,#5990,.T.);
#9170=EDGE_CURVE('',#7081,#7082,#4048,.T.);
#9171=EDGE_CURVE('',#7082,#7082,#5991,.T.);
#9172=EDGE_CURVE('',#7083,#7084,#5992,.T.);
#9173=EDGE_CURVE('',#7084,#7085,#5993,.T.);
#9174=EDGE_CURVE('',#7085,#7086,#4049,.T.);
#9175=EDGE_CURVE('',#7086,#7086,#5994,.T.);
#9176=EDGE_CURVE('',#7085,#7083,#5995,.T.);
#9177=EDGE_CURVE('',#7087,#7087,#5996,.T.);
#9178=EDGE_CURVE('',#7087,#7088,#4050,.T.);
#9179=EDGE_CURVE('',#7088,#7088,#5997,.T.);
#9180=EDGE_CURVE('',#7089,#7089,#5998,.T.);
#9181=EDGE_CURVE('',#7089,#7090,#4051,.T.);
#9182=EDGE_CURVE('',#7090,#7090,#5999,.T.);
#9183=EDGE_CURVE('',#7091,#7091,#6000,.T.);
#9184=EDGE_CURVE('',#7091,#7092,#4052,.T.);
#9185=EDGE_CURVE('',#7092,#7092,#6001,.T.);
#9186=EDGE_CURVE('',#7093,#7093,#6002,.T.);
#9187=EDGE_CURVE('',#7093,#7094,#4053,.T.);
#9188=EDGE_CURVE('',#7094,#7094,#6003,.T.);
#9189=EDGE_CURVE('',#7095,#7083,#4054,.T.);
#9190=EDGE_CURVE('',#7096,#7095,#4055,.T.);
#9191=EDGE_CURVE('',#7096,#7084,#4056,.T.);
#9192=EDGE_CURVE('',#7097,#7098,#4057,.T.);
#9193=EDGE_CURVE('',#7098,#7099,#6004,.T.);
#9194=EDGE_CURVE('',#7100,#7099,#4058,.T.);
#9195=EDGE_CURVE('',#7097,#7100,#6005,.T.);
#9196=EDGE_CURVE('',#7099,#7101,#4059,.T.);
#9197=EDGE_CURVE('',#7102,#7101,#4060,.T.);
#9198=EDGE_CURVE('',#7100,#7102,#4061,.T.);
#9199=EDGE_CURVE('',#7095,#7097,#4062,.T.);
#9200=EDGE_CURVE('',#7102,#7096,#4063,.T.);
#9201=EDGE_CURVE('',#7103,#7104,#4064,.T.);
#9202=EDGE_CURVE('',#7105,#7103,#4065,.T.);
#9203=EDGE_CURVE('',#7106,#7105,#4066,.T.);
#9204=EDGE_CURVE('',#7107,#7106,#6006,.T.);
#9205=EDGE_CURVE('',#7104,#7107,#4067,.T.);
#9206=EDGE_CURVE('',#7084,#7103,#4068,.T.);
#9207=EDGE_CURVE('',#7083,#7104,#4069,.T.);
#9208=EDGE_CURVE('',#7108,#7109,#4070,.T.);
#9209=EDGE_CURVE('',#7098,#7108,#4071,.T.);
#9210=EDGE_CURVE('',#7110,#7107,#4072,.T.);
#9211=EDGE_CURVE('',#7109,#7110,#4073,.T.);
#9212=EDGE_CURVE('',#7111,#7106,#4074,.T.);
#9213=EDGE_CURVE('',#7111,#7110,#6007,.T.);
#9214=EDGE_CURVE('',#7112,#7105,#4075,.T.);
#9215=EDGE_CURVE('',#7112,#7111,#4076,.T.);
#9216=EDGE_CURVE('',#7101,#7113,#4077,.T.);
#9217=EDGE_CURVE('',#7113,#7114,#4078,.T.);
#9218=EDGE_CURVE('',#7114,#7112,#4079,.T.);
#9219=EDGE_CURVE('',#7113,#7108,#4080,.T.);
#9220=EDGE_CURVE('',#7114,#7109,#4081,.T.);
#9221=EDGE_CURVE('',#7115,#7115,#6008,.T.);
#9222=EDGE_CURVE('',#7115,#7116,#4082,.T.);
#9223=EDGE_CURVE('',#7116,#7116,#6009,.T.);
#9224=EDGE_CURVE('',#7117,#7118,#6010,.T.);
#9225=EDGE_CURVE('',#7119,#7119,#6011,.T.);
#9226=EDGE_CURVE('',#7119,#7120,#6012,.T.);
#9227=EDGE_CURVE('',#7120,#7120,#6013,.T.);
#9228=EDGE_CURVE('',#7121,#7122,#6014,.T.);
#9229=EDGE_CURVE('',#7122,#7121,#6015,.T.);
#9230=EDGE_CURVE('',#7122,#7123,#4083,.T.);
#9231=EDGE_CURVE('',#7123,#7123,#6016,.T.);
#9232=EDGE_CURVE('',#7124,#7125,#6017,.T.);
#9233=EDGE_CURVE('',#7125,#7124,#6018,.T.);
#9234=EDGE_CURVE('',#7125,#7126,#4084,.T.);
#9235=EDGE_CURVE('',#7126,#7127,#6019,.T.);
#9236=EDGE_CURVE('',#7127,#7126,#6020,.T.);
#9237=EDGE_CURVE('',#7121,#7127,#4085,.T.);
#9238=EDGE_CURVE('',#7128,#7129,#6021,.T.);
#9239=EDGE_CURVE('',#7129,#7128,#6022,.T.);
#9240=EDGE_CURVE('',#7129,#7124,#4086,.T.);
#9241=EDGE_CURVE('',#7130,#7131,#6023,.T.);
#9242=EDGE_CURVE('',#7131,#7130,#6024,.T.);
#9243=EDGE_CURVE('',#7131,#7132,#4087,.T.);
#9244=EDGE_CURVE('',#7132,#7133,#6025,.T.);
#9245=EDGE_CURVE('',#7133,#7132,#6026,.T.);
#9246=EDGE_CURVE('',#7128,#7133,#4088,.T.);
#9247=EDGE_CURVE('',#7134,#7135,#6027,.T.);
#9248=EDGE_CURVE('',#7135,#7134,#6028,.T.);
#9249=EDGE_CURVE('',#7135,#7130,#4089,.T.);
#9250=EDGE_CURVE('',#7136,#7137,#6029,.T.);
#9251=EDGE_CURVE('',#7137,#7136,#6030,.T.);
#9252=EDGE_CURVE('',#7137,#7138,#4090,.T.);
#9253=EDGE_CURVE('',#7138,#7139,#6031,.T.);
#9254=EDGE_CURVE('',#7139,#7138,#6032,.T.);
#9255=EDGE_CURVE('',#7134,#7139,#4091,.T.);
#9256=EDGE_CURVE('',#7140,#7141,#6033,.T.);
#9257=EDGE_CURVE('',#7141,#7140,#6034,.T.);
#9258=EDGE_CURVE('',#7141,#7136,#4092,.T.);
#9259=EDGE_CURVE('',#7142,#7143,#6035,.T.);
#9260=EDGE_CURVE('',#7143,#7142,#6036,.T.);
#9261=EDGE_CURVE('',#7143,#7144,#4093,.T.);
#9262=EDGE_CURVE('',#7144,#7145,#6037,.T.);
#9263=EDGE_CURVE('',#7145,#7144,#6038,.T.);
#9264=EDGE_CURVE('',#7140,#7145,#4094,.T.);
#9265=EDGE_CURVE('',#7146,#7147,#6039,.T.);
#9266=EDGE_CURVE('',#7147,#7146,#6040,.T.);
#9267=EDGE_CURVE('',#7147,#7142,#4095,.T.);
#9268=EDGE_CURVE('',#7148,#7149,#6041,.T.);
#9269=EDGE_CURVE('',#7149,#7148,#6042,.T.);
#9270=EDGE_CURVE('',#7149,#7150,#4096,.T.);
#9271=EDGE_CURVE('',#7150,#7151,#6043,.T.);
#9272=EDGE_CURVE('',#7151,#7150,#6044,.T.);
#9273=EDGE_CURVE('',#7146,#7151,#4097,.T.);
#9274=EDGE_CURVE('',#7152,#7153,#6045,.T.);
#9275=EDGE_CURVE('',#7153,#7152,#6046,.T.);
#9276=EDGE_CURVE('',#7153,#7148,#4098,.T.);
#9277=EDGE_CURVE('',#7154,#7155,#6047,.T.);
#9278=EDGE_CURVE('',#7155,#7154,#6048,.T.);
#9279=EDGE_CURVE('',#7155,#7156,#4099,.T.);
#9280=EDGE_CURVE('',#7156,#7157,#6049,.T.);
#9281=EDGE_CURVE('',#7157,#7156,#6050,.T.);
#9282=EDGE_CURVE('',#7152,#7157,#4100,.T.);
#9283=EDGE_CURVE('',#7158,#7159,#6051,.T.);
#9284=EDGE_CURVE('',#7159,#7158,#6052,.T.);
#9285=EDGE_CURVE('',#7159,#7154,#4101,.T.);
#9286=EDGE_CURVE('',#7160,#7161,#6053,.T.);
#9287=EDGE_CURVE('',#7161,#7160,#6054,.T.);
#9288=EDGE_CURVE('',#7161,#7162,#4102,.T.);
#9289=EDGE_CURVE('',#7162,#7163,#6055,.T.);
#9290=EDGE_CURVE('',#7163,#7162,#6056,.T.);
#9291=EDGE_CURVE('',#7158,#7163,#4103,.T.);
#9292=EDGE_CURVE('',#7164,#7165,#6057,.T.);
#9293=EDGE_CURVE('',#7165,#7164,#6058,.T.);
#9294=EDGE_CURVE('',#7165,#7160,#4104,.T.);
#9295=EDGE_CURVE('',#7166,#7167,#6059,.T.);
#9296=EDGE_CURVE('',#7167,#7166,#6060,.T.);
#9297=EDGE_CURVE('',#7167,#7168,#4105,.T.);
#9298=EDGE_CURVE('',#7168,#7169,#6061,.T.);
#9299=EDGE_CURVE('',#7169,#7168,#6062,.T.);
#9300=EDGE_CURVE('',#7164,#7169,#4106,.T.);
#9301=EDGE_CURVE('',#7170,#7171,#6063,.T.);
#9302=EDGE_CURVE('',#7171,#7170,#6064,.T.);
#9303=EDGE_CURVE('',#7171,#7166,#4107,.T.);
#9304=EDGE_CURVE('',#7172,#7173,#6065,.T.);
#9305=EDGE_CURVE('',#7173,#7172,#6066,.T.);
#9306=EDGE_CURVE('',#7173,#7174,#4108,.T.);
#9307=EDGE_CURVE('',#7174,#7175,#6067,.T.);
#9308=EDGE_CURVE('',#7175,#7174,#6068,.T.);
#9309=EDGE_CURVE('',#7170,#7175,#4109,.T.);
#9310=EDGE_CURVE('',#7176,#7177,#6069,.T.);
#9311=EDGE_CURVE('',#7177,#7176,#6070,.T.);
#9312=EDGE_CURVE('',#7177,#7172,#4110,.T.);
#9313=EDGE_CURVE('',#7178,#7179,#6071,.T.);
#9314=EDGE_CURVE('',#7179,#7178,#6072,.T.);
#9315=EDGE_CURVE('',#7179,#7180,#4111,.T.);
#9316=EDGE_CURVE('',#7180,#7181,#6073,.T.);
#9317=EDGE_CURVE('',#7181,#7180,#6074,.T.);
#9318=EDGE_CURVE('',#7176,#7181,#4112,.T.);
#9319=EDGE_CURVE('',#7182,#7183,#6075,.T.);
#9320=EDGE_CURVE('',#7183,#7182,#6076,.T.);
#9321=EDGE_CURVE('',#7183,#7178,#4113,.T.);
#9322=EDGE_CURVE('',#7184,#7185,#6077,.T.);
#9323=EDGE_CURVE('',#7185,#7184,#6078,.T.);
#9324=EDGE_CURVE('',#7185,#7186,#4114,.T.);
#9325=EDGE_CURVE('',#7186,#7187,#6079,.T.);
#9326=EDGE_CURVE('',#7187,#7186,#6080,.T.);
#9327=EDGE_CURVE('',#7182,#7187,#4115,.T.);
#9328=EDGE_CURVE('',#7188,#7189,#6081,.T.);
#9329=EDGE_CURVE('',#7189,#7188,#6082,.T.);
#9330=EDGE_CURVE('',#7189,#7184,#4116,.T.);
#9331=EDGE_CURVE('',#7190,#7191,#6083,.T.);
#9332=EDGE_CURVE('',#7191,#7190,#6084,.T.);
#9333=EDGE_CURVE('',#7191,#7192,#4117,.T.);
#9334=EDGE_CURVE('',#7192,#7193,#6085,.T.);
#9335=EDGE_CURVE('',#7193,#7192,#6086,.T.);
#9336=EDGE_CURVE('',#7188,#7193,#4118,.T.);
#9337=EDGE_CURVE('',#7194,#7195,#6087,.T.);
#9338=EDGE_CURVE('',#7195,#7194,#6088,.T.);
#9339=EDGE_CURVE('',#7195,#7190,#4119,.T.);
#9340=EDGE_CURVE('',#7196,#7197,#6089,.T.);
#9341=EDGE_CURVE('',#7197,#7196,#6090,.T.);
#9342=EDGE_CURVE('',#7197,#7198,#4120,.T.);
#9343=EDGE_CURVE('',#7198,#7199,#6091,.T.);
#9344=EDGE_CURVE('',#7199,#7198,#6092,.T.);
#9345=EDGE_CURVE('',#7194,#7199,#4121,.T.);
#9346=EDGE_CURVE('',#7200,#7201,#6093,.T.);
#9347=EDGE_CURVE('',#7201,#7200,#6094,.T.);
#9348=EDGE_CURVE('',#7201,#7196,#4122,.T.);
#9349=EDGE_CURVE('',#7202,#7203,#6095,.T.);
#9350=EDGE_CURVE('',#7203,#7202,#6096,.T.);
#9351=EDGE_CURVE('',#7203,#7204,#4123,.T.);
#9352=EDGE_CURVE('',#7204,#7205,#6097,.T.);
#9353=EDGE_CURVE('',#7205,#7204,#6098,.T.);
#9354=EDGE_CURVE('',#7200,#7205,#4124,.T.);
#9355=EDGE_CURVE('',#7206,#7207,#6099,.T.);
#9356=EDGE_CURVE('',#7207,#7206,#6100,.T.);
#9357=EDGE_CURVE('',#7207,#7202,#4125,.T.);
#9358=EDGE_CURVE('',#7208,#7209,#6101,.T.);
#9359=EDGE_CURVE('',#7209,#7208,#6102,.T.);
#9360=EDGE_CURVE('',#7209,#7210,#4126,.T.);
#9361=EDGE_CURVE('',#7210,#7211,#6103,.T.);
#9362=EDGE_CURVE('',#7211,#7210,#6104,.T.);
#9363=EDGE_CURVE('',#7206,#7211,#4127,.T.);
#9364=EDGE_CURVE('',#7212,#7213,#242,.T.);
#9365=EDGE_CURVE('',#7212,#7214,#6105,.T.);
#9366=EDGE_CURVE('',#7215,#7214,#243,.T.);
#9367=EDGE_CURVE('',#7216,#7215,#244,.T.);
#9368=EDGE_CURVE('',#7216,#7217,#6106,.T.);
#9369=EDGE_CURVE('',#7218,#7217,#245,.T.);
#9370=EDGE_CURVE('',#7219,#7218,#246,.T.);
#9371=EDGE_CURVE('',#7219,#7220,#6107,.T.);
#9372=EDGE_CURVE('',#7221,#7220,#247,.T.);
#9373=EDGE_CURVE('',#7222,#7221,#248,.T.);
#9374=EDGE_CURVE('',#7222,#7223,#6108,.T.);
#9375=EDGE_CURVE('',#7224,#7223,#249,.T.);
#9376=EDGE_CURVE('',#7225,#7224,#250,.T.);
#9377=EDGE_CURVE('',#7225,#7226,#6109,.T.);
#9378=EDGE_CURVE('',#7227,#7226,#251,.T.);
#9379=EDGE_CURVE('',#7228,#7227,#252,.T.);
#9380=EDGE_CURVE('',#7228,#7229,#6110,.T.);
#9381=EDGE_CURVE('',#7230,#7229,#253,.T.);
#9382=EDGE_CURVE('',#7231,#7230,#254,.T.);
#9383=EDGE_CURVE('',#7231,#7232,#6111,.T.);
#9384=EDGE_CURVE('',#7233,#7232,#255,.T.);
#9385=EDGE_CURVE('',#7234,#7233,#256,.T.);
#9386=EDGE_CURVE('',#7234,#7235,#6112,.T.);
#9387=EDGE_CURVE('',#7236,#7235,#257,.T.);
#9388=EDGE_CURVE('',#7237,#7236,#258,.T.);
#9389=EDGE_CURVE('',#7237,#7238,#6113,.T.);
#9390=EDGE_CURVE('',#7239,#7238,#259,.T.);
#9391=EDGE_CURVE('',#7240,#7239,#260,.T.);
#9392=EDGE_CURVE('',#7240,#7241,#6114,.T.);
#9393=EDGE_CURVE('',#7242,#7241,#261,.T.);
#9394=EDGE_CURVE('',#7243,#7242,#262,.T.);
#9395=EDGE_CURVE('',#7243,#7244,#6115,.T.);
#9396=EDGE_CURVE('',#7245,#7244,#263,.T.);
#9397=EDGE_CURVE('',#7246,#7245,#264,.T.);
#9398=EDGE_CURVE('',#7246,#7247,#6116,.T.);
#9399=EDGE_CURVE('',#7248,#7247,#265,.T.);
#9400=EDGE_CURVE('',#7249,#7248,#266,.T.);
#9401=EDGE_CURVE('',#7249,#7250,#6117,.T.);
#9402=EDGE_CURVE('',#7251,#7250,#267,.T.);
#9403=EDGE_CURVE('',#7252,#7251,#268,.T.);
#9404=EDGE_CURVE('',#7252,#7253,#6118,.T.);
#9405=EDGE_CURVE('',#7254,#7253,#269,.T.);
#9406=EDGE_CURVE('',#7255,#7254,#270,.T.);
#9407=EDGE_CURVE('',#7255,#7256,#6119,.T.);
#9408=EDGE_CURVE('',#7257,#7256,#271,.T.);
#9409=EDGE_CURVE('',#7258,#7257,#272,.T.);
#9410=EDGE_CURVE('',#7258,#7259,#6120,.T.);
#9411=EDGE_CURVE('',#7260,#7259,#273,.T.);
#9412=EDGE_CURVE('',#7261,#7260,#274,.T.);
#9413=EDGE_CURVE('',#7261,#7262,#6121,.T.);
#9414=EDGE_CURVE('',#7263,#7262,#275,.T.);
#9415=EDGE_CURVE('',#7264,#7263,#276,.T.);
#9416=EDGE_CURVE('',#7264,#7265,#6122,.T.);
#9417=EDGE_CURVE('',#7266,#7265,#277,.T.);
#9418=EDGE_CURVE('',#7267,#7266,#278,.T.);
#9419=EDGE_CURVE('',#7267,#7268,#6123,.T.);
#9420=EDGE_CURVE('',#7269,#7268,#279,.T.);
#9421=EDGE_CURVE('',#7270,#7269,#280,.T.);
#9422=EDGE_CURVE('',#7270,#7271,#6124,.T.);
#9423=EDGE_CURVE('',#7272,#7271,#281,.T.);
#9424=EDGE_CURVE('',#7273,#7272,#282,.T.);
#9425=EDGE_CURVE('',#7273,#7274,#6125,.T.);
#9426=EDGE_CURVE('',#7275,#7274,#283,.T.);
#9427=EDGE_CURVE('',#7276,#7275,#284,.T.);
#9428=EDGE_CURVE('',#7276,#7277,#6126,.T.);
#9429=EDGE_CURVE('',#7278,#7277,#285,.T.);
#9430=EDGE_CURVE('',#7279,#7278,#286,.T.);
#9431=EDGE_CURVE('',#7279,#7280,#6127,.T.);
#9432=EDGE_CURVE('',#7281,#7280,#287,.T.);
#9433=EDGE_CURVE('',#7282,#7281,#288,.T.);
#9434=EDGE_CURVE('',#7282,#7283,#6128,.T.);
#9435=EDGE_CURVE('',#7284,#7283,#289,.T.);
#9436=EDGE_CURVE('',#7285,#7284,#290,.T.);
#9437=EDGE_CURVE('',#7285,#7286,#6129,.T.);
#9438=EDGE_CURVE('',#7287,#7286,#291,.T.);
#9439=EDGE_CURVE('',#7288,#7287,#292,.T.);
#9440=EDGE_CURVE('',#7288,#7289,#6130,.T.);
#9441=EDGE_CURVE('',#7290,#7289,#293,.T.);
#9442=EDGE_CURVE('',#7291,#7290,#294,.T.);
#9443=EDGE_CURVE('',#7291,#7292,#6131,.T.);
#9444=EDGE_CURVE('',#7293,#7292,#295,.T.);
#9445=EDGE_CURVE('',#7294,#7293,#296,.T.);
#9446=EDGE_CURVE('',#7294,#7295,#6132,.T.);
#9447=EDGE_CURVE('',#7296,#7295,#297,.T.);
#9448=EDGE_CURVE('',#7297,#7296,#298,.T.);
#9449=EDGE_CURVE('',#7297,#7298,#6133,.T.);
#9450=EDGE_CURVE('',#7299,#7298,#299,.T.);
#9451=EDGE_CURVE('',#7300,#7299,#300,.T.);
#9452=EDGE_CURVE('',#7300,#7301,#6134,.T.);
#9453=EDGE_CURVE('',#7302,#7301,#301,.T.);
#9454=EDGE_CURVE('',#7303,#7302,#302,.T.);
#9455=EDGE_CURVE('',#7303,#7304,#6135,.T.);
#9456=EDGE_CURVE('',#7305,#7304,#303,.T.);
#9457=EDGE_CURVE('',#7306,#7305,#304,.T.);
#9458=EDGE_CURVE('',#7306,#7307,#6136,.T.);
#9459=EDGE_CURVE('',#7308,#7307,#305,.T.);
#9460=EDGE_CURVE('',#7309,#7308,#306,.T.);
#9461=EDGE_CURVE('',#7309,#7310,#6137,.T.);
#9462=EDGE_CURVE('',#7311,#7310,#307,.T.);
#9463=EDGE_CURVE('',#7312,#7311,#308,.T.);
#9464=EDGE_CURVE('',#7312,#7313,#6138,.T.);
#9465=EDGE_CURVE('',#7314,#7313,#309,.T.);
#9466=EDGE_CURVE('',#7315,#7314,#310,.T.);
#9467=EDGE_CURVE('',#7315,#7316,#6139,.T.);
#9468=EDGE_CURVE('',#7317,#7316,#311,.T.);
#9469=EDGE_CURVE('',#7318,#7317,#312,.T.);
#9470=EDGE_CURVE('',#7318,#7319,#6140,.T.);
#9471=EDGE_CURVE('',#7320,#7319,#313,.T.);
#9472=EDGE_CURVE('',#7321,#7320,#314,.T.);
#9473=EDGE_CURVE('',#7321,#7322,#6141,.T.);
#9474=EDGE_CURVE('',#7323,#7322,#315,.T.);
#9475=EDGE_CURVE('',#7324,#7323,#316,.T.);
#9476=EDGE_CURVE('',#7324,#7325,#6142,.T.);
#9477=EDGE_CURVE('',#7326,#7325,#317,.T.);
#9478=EDGE_CURVE('',#7327,#7326,#318,.T.);
#9479=EDGE_CURVE('',#7327,#7328,#6143,.T.);
#9480=EDGE_CURVE('',#7329,#7328,#319,.F.);
#9481=EDGE_CURVE('',#7329,#7330,#4128,.T.);
#9482=EDGE_CURVE('',#7330,#7330,#6144,.T.);
#9483=EDGE_CURVE('',#7331,#7329,#320,.F.);
#9484=EDGE_CURVE('',#7332,#7331,#321,.T.);
#9485=EDGE_CURVE('',#7332,#7333,#6145,.T.);
#9486=EDGE_CURVE('',#7334,#7333,#322,.T.);
#9487=EDGE_CURVE('',#7335,#7334,#323,.T.);
#9488=EDGE_CURVE('',#7335,#7336,#6146,.T.);
#9489=EDGE_CURVE('',#7337,#7336,#324,.T.);
#9490=EDGE_CURVE('',#7338,#7337,#325,.T.);
#9491=EDGE_CURVE('',#7338,#7339,#6147,.T.);
#9492=EDGE_CURVE('',#7340,#7339,#326,.T.);
#9493=EDGE_CURVE('',#7341,#7340,#327,.T.);
#9494=EDGE_CURVE('',#7341,#7342,#6148,.T.);
#9495=EDGE_CURVE('',#7343,#7342,#328,.T.);
#9496=EDGE_CURVE('',#7344,#7343,#329,.T.);
#9497=EDGE_CURVE('',#7344,#7345,#6149,.T.);
#9498=EDGE_CURVE('',#7346,#7345,#330,.T.);
#9499=EDGE_CURVE('',#7347,#7346,#331,.T.);
#9500=EDGE_CURVE('',#7347,#7348,#6150,.T.);
#9501=EDGE_CURVE('',#7349,#7348,#332,.T.);
#9502=EDGE_CURVE('',#7350,#7349,#333,.T.);
#9503=EDGE_CURVE('',#7350,#7351,#6151,.T.);
#9504=EDGE_CURVE('',#7352,#7351,#334,.T.);
#9505=EDGE_CURVE('',#7353,#7352,#335,.T.);
#9506=EDGE_CURVE('',#7353,#7354,#6152,.T.);
#9507=EDGE_CURVE('',#7355,#7354,#336,.T.);
#9508=EDGE_CURVE('',#7356,#7355,#337,.T.);
#9509=EDGE_CURVE('',#7356,#7357,#6153,.T.);
#9510=EDGE_CURVE('',#7358,#7357,#338,.T.);
#9511=EDGE_CURVE('',#7359,#7358,#339,.T.);
#9512=EDGE_CURVE('',#7359,#7360,#6154,.T.);
#9513=EDGE_CURVE('',#7361,#7360,#340,.T.);
#9514=EDGE_CURVE('',#7362,#7361,#341,.T.);
#9515=EDGE_CURVE('',#7362,#7363,#6155,.T.);
#9516=EDGE_CURVE('',#7364,#7363,#342,.T.);
#9517=EDGE_CURVE('',#7365,#7364,#343,.T.);
#9518=EDGE_CURVE('',#7365,#7366,#6156,.T.);
#9519=EDGE_CURVE('',#7367,#7366,#344,.T.);
#9520=EDGE_CURVE('',#7368,#7367,#345,.T.);
#9521=EDGE_CURVE('',#7368,#7369,#6157,.T.);
#9522=EDGE_CURVE('',#7370,#7369,#346,.T.);
#9523=EDGE_CURVE('',#7371,#7370,#347,.T.);
#9524=EDGE_CURVE('',#7371,#7372,#6158,.T.);
#9525=EDGE_CURVE('',#7373,#7372,#348,.T.);
#9526=EDGE_CURVE('',#7374,#7373,#349,.T.);
#9527=EDGE_CURVE('',#7374,#7375,#6159,.T.);
#9528=EDGE_CURVE('',#7376,#7375,#350,.T.);
#9529=EDGE_CURVE('',#7377,#7376,#351,.T.);
#9530=EDGE_CURVE('',#7377,#7378,#6160,.T.);
#9531=EDGE_CURVE('',#7379,#7378,#352,.T.);
#9532=EDGE_CURVE('',#7380,#7379,#353,.T.);
#9533=EDGE_CURVE('',#7380,#7381,#6161,.T.);
#9534=EDGE_CURVE('',#7382,#7381,#354,.T.);
#9535=EDGE_CURVE('',#7383,#7382,#355,.T.);
#9536=EDGE_CURVE('',#7383,#7384,#6162,.T.);
#9537=EDGE_CURVE('',#7385,#7384,#356,.T.);
#9538=EDGE_CURVE('',#7386,#7385,#357,.T.);
#9539=EDGE_CURVE('',#7386,#7387,#6163,.T.);
#9540=EDGE_CURVE('',#7388,#7387,#358,.T.);
#9541=EDGE_CURVE('',#7389,#7388,#359,.T.);
#9542=EDGE_CURVE('',#7389,#7390,#6164,.T.);
#9543=EDGE_CURVE('',#7391,#7390,#360,.T.);
#9544=EDGE_CURVE('',#7392,#7391,#361,.T.);
#9545=EDGE_CURVE('',#7392,#7393,#6165,.T.);
#9546=EDGE_CURVE('',#7394,#7393,#362,.T.);
#9547=EDGE_CURVE('',#7395,#7394,#363,.T.);
#9548=EDGE_CURVE('',#7395,#7396,#6166,.T.);
#9549=EDGE_CURVE('',#7397,#7396,#364,.T.);
#9550=EDGE_CURVE('',#7398,#7397,#365,.T.);
#9551=EDGE_CURVE('',#7398,#7399,#6167,.T.);
#9552=EDGE_CURVE('',#7400,#7399,#366,.T.);
#9553=EDGE_CURVE('',#7401,#7400,#367,.T.);
#9554=EDGE_CURVE('',#7401,#7402,#6168,.T.);
#9555=EDGE_CURVE('',#7403,#7402,#368,.T.);
#9556=EDGE_CURVE('',#7404,#7403,#369,.T.);
#9557=EDGE_CURVE('',#7404,#7405,#6169,.T.);
#9558=EDGE_CURVE('',#7406,#7405,#370,.T.);
#9559=EDGE_CURVE('',#7407,#7406,#371,.T.);
#9560=EDGE_CURVE('',#7407,#7408,#6170,.T.);
#9561=EDGE_CURVE('',#7409,#7408,#372,.T.);
#9562=EDGE_CURVE('',#7410,#7409,#373,.T.);
#9563=EDGE_CURVE('',#7410,#7411,#6171,.T.);
#9564=EDGE_CURVE('',#7412,#7411,#374,.T.);
#9565=EDGE_CURVE('',#7413,#7412,#375,.T.);
#9566=EDGE_CURVE('',#7413,#7414,#6172,.T.);
#9567=EDGE_CURVE('',#7415,#7414,#376,.T.);
#9568=EDGE_CURVE('',#7416,#7415,#377,.T.);
#9569=EDGE_CURVE('',#7416,#7417,#6173,.T.);
#9570=EDGE_CURVE('',#7418,#7417,#378,.T.);
#9571=EDGE_CURVE('',#7419,#7418,#379,.T.);
#9572=EDGE_CURVE('',#7419,#7420,#6174,.T.);
#9573=EDGE_CURVE('',#7421,#7420,#380,.T.);
#9574=EDGE_CURVE('',#7422,#7421,#381,.T.);
#9575=EDGE_CURVE('',#7422,#7423,#6175,.T.);
#9576=EDGE_CURVE('',#7424,#7423,#382,.T.);
#9577=EDGE_CURVE('',#7425,#7424,#383,.T.);
#9578=EDGE_CURVE('',#7425,#7426,#6176,.T.);
#9579=EDGE_CURVE('',#7427,#7426,#384,.T.);
#9580=EDGE_CURVE('',#7428,#7427,#385,.T.);
#9581=EDGE_CURVE('',#7428,#7429,#6177,.T.);
#9582=EDGE_CURVE('',#7430,#7429,#386,.T.);
#9583=EDGE_CURVE('',#7431,#7430,#387,.T.);
#9584=EDGE_CURVE('',#7431,#7432,#6178,.T.);
#9585=EDGE_CURVE('',#7433,#7432,#388,.T.);
#9586=EDGE_CURVE('',#7434,#7433,#389,.T.);
#9587=EDGE_CURVE('',#7434,#7435,#6179,.T.);
#9588=EDGE_CURVE('',#7436,#7435,#390,.T.);
#9589=EDGE_CURVE('',#7437,#7436,#391,.T.);
#9590=EDGE_CURVE('',#7437,#7438,#6180,.T.);
#9591=EDGE_CURVE('',#7439,#7438,#392,.T.);
#9592=EDGE_CURVE('',#7440,#7439,#393,.T.);
#9593=EDGE_CURVE('',#7440,#7441,#6181,.T.);
#9594=EDGE_CURVE('',#7442,#7441,#394,.T.);
#9595=EDGE_CURVE('',#7443,#7442,#395,.T.);
#9596=EDGE_CURVE('',#7443,#7444,#6182,.T.);
#9597=EDGE_CURVE('',#7213,#7444,#396,.T.);
#9598=EDGE_CURVE('',#7445,#7446,#397,.F.);
#9599=EDGE_CURVE('',#7447,#7446,#6183,.T.);
#9600=EDGE_CURVE('',#7447,#7448,#398,.T.);
#9601=EDGE_CURVE('',#7448,#7449,#399,.T.);
#9602=EDGE_CURVE('',#7450,#7449,#6184,.T.);
#9603=EDGE_CURVE('',#7450,#7451,#400,.T.);
#9604=EDGE_CURVE('',#7451,#7452,#401,.T.);
#9605=EDGE_CURVE('',#7453,#7452,#6185,.T.);
#9606=EDGE_CURVE('',#7453,#7454,#402,.T.);
#9607=EDGE_CURVE('',#7454,#7455,#403,.T.);
#9608=EDGE_CURVE('',#7456,#7455,#6186,.T.);
#9609=EDGE_CURVE('',#7456,#7457,#404,.T.);
#9610=EDGE_CURVE('',#7457,#7458,#405,.T.);
#9611=EDGE_CURVE('',#7459,#7458,#6187,.T.);
#9612=EDGE_CURVE('',#7459,#7460,#406,.T.);
#9613=EDGE_CURVE('',#7460,#7461,#407,.T.);
#9614=EDGE_CURVE('',#7462,#7461,#6188,.T.);
#9615=EDGE_CURVE('',#7462,#7463,#408,.T.);
#9616=EDGE_CURVE('',#7463,#7464,#409,.T.);
#9617=EDGE_CURVE('',#7465,#7464,#6189,.T.);
#9618=EDGE_CURVE('',#7465,#7466,#410,.T.);
#9619=EDGE_CURVE('',#7466,#7467,#411,.T.);
#9620=EDGE_CURVE('',#7468,#7467,#6190,.T.);
#9621=EDGE_CURVE('',#7468,#7469,#412,.T.);
#9622=EDGE_CURVE('',#7469,#7470,#413,.T.);
#9623=EDGE_CURVE('',#7471,#7470,#6191,.T.);
#9624=EDGE_CURVE('',#7471,#7472,#414,.T.);
#9625=EDGE_CURVE('',#7472,#7473,#415,.T.);
#9626=EDGE_CURVE('',#7474,#7473,#6192,.T.);
#9627=EDGE_CURVE('',#7474,#7475,#416,.T.);
#9628=EDGE_CURVE('',#7475,#7476,#417,.T.);
#9629=EDGE_CURVE('',#7477,#7476,#6193,.T.);
#9630=EDGE_CURVE('',#7477,#7478,#418,.T.);
#9631=EDGE_CURVE('',#7478,#7479,#419,.T.);
#9632=EDGE_CURVE('',#7480,#7479,#6194,.T.);
#9633=EDGE_CURVE('',#7480,#7481,#420,.T.);
#9634=EDGE_CURVE('',#7481,#7482,#421,.T.);
#9635=EDGE_CURVE('',#7483,#7482,#6195,.T.);
#9636=EDGE_CURVE('',#7483,#7484,#422,.T.);
#9637=EDGE_CURVE('',#7484,#7485,#423,.T.);
#9638=EDGE_CURVE('',#7486,#7485,#6196,.T.);
#9639=EDGE_CURVE('',#7486,#7487,#424,.T.);
#9640=EDGE_CURVE('',#7487,#7488,#425,.T.);
#9641=EDGE_CURVE('',#7489,#7488,#6197,.T.);
#9642=EDGE_CURVE('',#7489,#7490,#426,.T.);
#9643=EDGE_CURVE('',#7490,#7491,#427,.T.);
#9644=EDGE_CURVE('',#7492,#7491,#6198,.T.);
#9645=EDGE_CURVE('',#7492,#7493,#428,.T.);
#9646=EDGE_CURVE('',#7493,#7494,#429,.T.);
#9647=EDGE_CURVE('',#7495,#7494,#6199,.T.);
#9648=EDGE_CURVE('',#7495,#7496,#430,.T.);
#9649=EDGE_CURVE('',#7496,#7497,#431,.T.);
#9650=EDGE_CURVE('',#7498,#7497,#6200,.T.);
#9651=EDGE_CURVE('',#7498,#7499,#432,.T.);
#9652=EDGE_CURVE('',#7499,#7500,#433,.T.);
#9653=EDGE_CURVE('',#7501,#7500,#6201,.T.);
#9654=EDGE_CURVE('',#7501,#7502,#434,.T.);
#9655=EDGE_CURVE('',#7502,#7503,#435,.T.);
#9656=EDGE_CURVE('',#7504,#7503,#6202,.T.);
#9657=EDGE_CURVE('',#7504,#7505,#436,.T.);
#9658=EDGE_CURVE('',#7505,#7506,#437,.T.);
#9659=EDGE_CURVE('',#7507,#7506,#6203,.T.);
#9660=EDGE_CURVE('',#7507,#7508,#438,.T.);
#9661=EDGE_CURVE('',#7508,#7509,#439,.T.);
#9662=EDGE_CURVE('',#7510,#7509,#6204,.T.);
#9663=EDGE_CURVE('',#7510,#7511,#440,.T.);
#9664=EDGE_CURVE('',#7511,#7512,#441,.T.);
#9665=EDGE_CURVE('',#7513,#7512,#6205,.T.);
#9666=EDGE_CURVE('',#7513,#7514,#442,.T.);
#9667=EDGE_CURVE('',#7514,#7515,#443,.T.);
#9668=EDGE_CURVE('',#7516,#7515,#6206,.T.);
#9669=EDGE_CURVE('',#7516,#7517,#444,.T.);
#9670=EDGE_CURVE('',#7517,#7518,#445,.T.);
#9671=EDGE_CURVE('',#7519,#7518,#6207,.T.);
#9672=EDGE_CURVE('',#7519,#7520,#446,.T.);
#9673=EDGE_CURVE('',#7520,#7521,#447,.T.);
#9674=EDGE_CURVE('',#7522,#7521,#6208,.T.);
#9675=EDGE_CURVE('',#7522,#7523,#448,.T.);
#9676=EDGE_CURVE('',#7523,#7524,#449,.T.);
#9677=EDGE_CURVE('',#7525,#7524,#6209,.T.);
#9678=EDGE_CURVE('',#7525,#7526,#450,.T.);
#9679=EDGE_CURVE('',#7526,#7527,#451,.T.);
#9680=EDGE_CURVE('',#7528,#7527,#6210,.T.);
#9681=EDGE_CURVE('',#7528,#7529,#452,.T.);
#9682=EDGE_CURVE('',#7529,#7530,#453,.T.);
#9683=EDGE_CURVE('',#7531,#7530,#6211,.T.);
#9684=EDGE_CURVE('',#7531,#7532,#454,.T.);
#9685=EDGE_CURVE('',#7532,#7533,#455,.T.);
#9686=EDGE_CURVE('',#7534,#7533,#6212,.T.);
#9687=EDGE_CURVE('',#7534,#7535,#456,.T.);
#9688=EDGE_CURVE('',#7535,#7536,#457,.T.);
#9689=EDGE_CURVE('',#7537,#7536,#6213,.T.);
#9690=EDGE_CURVE('',#7537,#7538,#458,.T.);
#9691=EDGE_CURVE('',#7538,#7539,#459,.T.);
#9692=EDGE_CURVE('',#7540,#7539,#6214,.T.);
#9693=EDGE_CURVE('',#7540,#7541,#460,.T.);
#9694=EDGE_CURVE('',#7541,#7542,#461,.T.);
#9695=EDGE_CURVE('',#7543,#7542,#6215,.T.);
#9696=EDGE_CURVE('',#7543,#7544,#462,.T.);
#9697=EDGE_CURVE('',#7544,#7545,#463,.T.);
#9698=EDGE_CURVE('',#7546,#7545,#6216,.T.);
#9699=EDGE_CURVE('',#7546,#7547,#464,.T.);
#9700=EDGE_CURVE('',#7547,#7548,#465,.T.);
#9701=EDGE_CURVE('',#7549,#7548,#6217,.T.);
#9702=EDGE_CURVE('',#7549,#7550,#466,.T.);
#9703=EDGE_CURVE('',#7550,#7551,#467,.T.);
#9704=EDGE_CURVE('',#7552,#7551,#6218,.T.);
#9705=EDGE_CURVE('',#7552,#7553,#468,.T.);
#9706=EDGE_CURVE('',#7553,#7554,#469,.T.);
#9707=EDGE_CURVE('',#7555,#7554,#6219,.T.);
#9708=EDGE_CURVE('',#7555,#7556,#470,.T.);
#9709=EDGE_CURVE('',#7556,#7557,#471,.T.);
#9710=EDGE_CURVE('',#7558,#7557,#6220,.T.);
#9711=EDGE_CURVE('',#7558,#7559,#472,.T.);
#9712=EDGE_CURVE('',#7559,#7560,#473,.T.);
#9713=EDGE_CURVE('',#7561,#7560,#6221,.T.);
#9714=EDGE_CURVE('',#7561,#7562,#474,.T.);
#9715=EDGE_CURVE('',#7562,#7563,#4129,.T.);
#9716=EDGE_CURVE('',#7563,#7563,#6222,.T.);
#9717=EDGE_CURVE('',#7562,#7564,#475,.T.);
#9718=EDGE_CURVE('',#7564,#7565,#476,.T.);
#9719=EDGE_CURVE('',#7566,#7565,#6223,.T.);
#9720=EDGE_CURVE('',#7566,#7567,#477,.T.);
#9721=EDGE_CURVE('',#7567,#7568,#478,.T.);
#9722=EDGE_CURVE('',#7569,#7568,#6224,.T.);
#9723=EDGE_CURVE('',#7569,#7570,#479,.T.);
#9724=EDGE_CURVE('',#7570,#7571,#480,.T.);
#9725=EDGE_CURVE('',#7572,#7571,#6225,.T.);
#9726=EDGE_CURVE('',#7572,#7573,#481,.T.);
#9727=EDGE_CURVE('',#7573,#7574,#482,.T.);
#9728=EDGE_CURVE('',#7575,#7574,#6226,.T.);
#9729=EDGE_CURVE('',#7575,#7576,#483,.T.);
#9730=EDGE_CURVE('',#7576,#7577,#484,.T.);
#9731=EDGE_CURVE('',#7578,#7577,#6227,.T.);
#9732=EDGE_CURVE('',#7578,#7579,#485,.T.);
#9733=EDGE_CURVE('',#7579,#7580,#486,.T.);
#9734=EDGE_CURVE('',#7581,#7580,#6228,.T.);
#9735=EDGE_CURVE('',#7581,#7582,#487,.T.);
#9736=EDGE_CURVE('',#7582,#7583,#488,.T.);
#9737=EDGE_CURVE('',#7584,#7583,#6229,.T.);
#9738=EDGE_CURVE('',#7584,#7585,#489,.T.);
#9739=EDGE_CURVE('',#7585,#7586,#490,.T.);
#9740=EDGE_CURVE('',#7587,#7586,#6230,.T.);
#9741=EDGE_CURVE('',#7587,#7588,#491,.T.);
#9742=EDGE_CURVE('',#7588,#7589,#492,.T.);
#9743=EDGE_CURVE('',#7590,#7589,#6231,.T.);
#9744=EDGE_CURVE('',#7590,#7591,#493,.T.);
#9745=EDGE_CURVE('',#7591,#7592,#494,.T.);
#9746=EDGE_CURVE('',#7593,#7592,#6232,.T.);
#9747=EDGE_CURVE('',#7593,#7594,#495,.T.);
#9748=EDGE_CURVE('',#7594,#7595,#496,.T.);
#9749=EDGE_CURVE('',#7596,#7595,#6233,.T.);
#9750=EDGE_CURVE('',#7596,#7597,#497,.T.);
#9751=EDGE_CURVE('',#7597,#7598,#498,.T.);
#9752=EDGE_CURVE('',#7599,#7598,#6234,.T.);
#9753=EDGE_CURVE('',#7599,#7600,#499,.T.);
#9754=EDGE_CURVE('',#7600,#7601,#500,.T.);
#9755=EDGE_CURVE('',#7602,#7601,#6235,.T.);
#9756=EDGE_CURVE('',#7602,#7603,#501,.T.);
#9757=EDGE_CURVE('',#7603,#7604,#502,.T.);
#9758=EDGE_CURVE('',#7605,#7604,#6236,.T.);
#9759=EDGE_CURVE('',#7605,#7606,#503,.T.);
#9760=EDGE_CURVE('',#7606,#7607,#504,.T.);
#9761=EDGE_CURVE('',#7608,#7607,#6237,.T.);
#9762=EDGE_CURVE('',#7608,#7609,#505,.T.);
#9763=EDGE_CURVE('',#7609,#7610,#506,.T.);
#9764=EDGE_CURVE('',#7611,#7610,#6238,.T.);
#9765=EDGE_CURVE('',#7611,#7612,#507,.T.);
#9766=EDGE_CURVE('',#7612,#7613,#508,.T.);
#9767=EDGE_CURVE('',#7614,#7613,#6239,.T.);
#9768=EDGE_CURVE('',#7614,#7615,#509,.T.);
#9769=EDGE_CURVE('',#7615,#7616,#510,.T.);
#9770=EDGE_CURVE('',#7617,#7616,#6240,.T.);
#9771=EDGE_CURVE('',#7617,#7618,#511,.T.);
#9772=EDGE_CURVE('',#7618,#7619,#512,.T.);
#9773=EDGE_CURVE('',#7620,#7619,#6241,.T.);
#9774=EDGE_CURVE('',#7620,#7621,#513,.T.);
#9775=EDGE_CURVE('',#7621,#7622,#514,.T.);
#9776=EDGE_CURVE('',#7623,#7622,#6242,.T.);
#9777=EDGE_CURVE('',#7623,#7624,#515,.T.);
#9778=EDGE_CURVE('',#7624,#7625,#516,.T.);
#9779=EDGE_CURVE('',#7626,#7625,#6243,.T.);
#9780=EDGE_CURVE('',#7626,#7627,#517,.T.);
#9781=EDGE_CURVE('',#7627,#7628,#518,.T.);
#9782=EDGE_CURVE('',#7629,#7628,#6244,.T.);
#9783=EDGE_CURVE('',#7629,#7630,#519,.T.);
#9784=EDGE_CURVE('',#7630,#7631,#520,.T.);
#9785=EDGE_CURVE('',#7632,#7631,#6245,.T.);
#9786=EDGE_CURVE('',#7632,#7633,#521,.T.);
#9787=EDGE_CURVE('',#7633,#7634,#522,.T.);
#9788=EDGE_CURVE('',#7635,#7634,#6246,.T.);
#9789=EDGE_CURVE('',#7635,#7636,#523,.T.);
#9790=EDGE_CURVE('',#7636,#7637,#524,.T.);
#9791=EDGE_CURVE('',#7638,#7637,#6247,.T.);
#9792=EDGE_CURVE('',#7638,#7639,#525,.T.);
#9793=EDGE_CURVE('',#7639,#7640,#526,.T.);
#9794=EDGE_CURVE('',#7641,#7640,#6248,.T.);
#9795=EDGE_CURVE('',#7641,#7642,#527,.T.);
#9796=EDGE_CURVE('',#7642,#7643,#528,.T.);
#9797=EDGE_CURVE('',#7644,#7643,#6249,.T.);
#9798=EDGE_CURVE('',#7644,#7645,#529,.T.);
#9799=EDGE_CURVE('',#7645,#7646,#530,.T.);
#9800=EDGE_CURVE('',#7647,#7646,#6250,.T.);
#9801=EDGE_CURVE('',#7647,#7648,#531,.T.);
#9802=EDGE_CURVE('',#7648,#7649,#532,.T.);
#9803=EDGE_CURVE('',#7650,#7649,#6251,.T.);
#9804=EDGE_CURVE('',#7650,#7651,#533,.T.);
#9805=EDGE_CURVE('',#7651,#7652,#534,.T.);
#9806=EDGE_CURVE('',#7653,#7652,#6252,.T.);
#9807=EDGE_CURVE('',#7653,#7654,#535,.T.);
#9808=EDGE_CURVE('',#7654,#7655,#536,.T.);
#9809=EDGE_CURVE('',#7656,#7655,#6253,.T.);
#9810=EDGE_CURVE('',#7656,#7657,#537,.T.);
#9811=EDGE_CURVE('',#7657,#7658,#538,.T.);
#9812=EDGE_CURVE('',#7659,#7658,#6254,.T.);
#9813=EDGE_CURVE('',#7659,#7660,#539,.T.);
#9814=EDGE_CURVE('',#7660,#7661,#540,.T.);
#9815=EDGE_CURVE('',#7662,#7661,#6255,.T.);
#9816=EDGE_CURVE('',#7662,#7663,#541,.T.);
#9817=EDGE_CURVE('',#7663,#7664,#542,.T.);
#9818=EDGE_CURVE('',#7665,#7664,#6256,.T.);
#9819=EDGE_CURVE('',#7665,#7666,#543,.T.);
#9820=EDGE_CURVE('',#7666,#7667,#544,.T.);
#9821=EDGE_CURVE('',#7668,#7667,#6257,.T.);
#9822=EDGE_CURVE('',#7668,#7669,#545,.T.);
#9823=EDGE_CURVE('',#7669,#7670,#546,.T.);
#9824=EDGE_CURVE('',#7671,#7670,#6258,.T.);
#9825=EDGE_CURVE('',#7671,#7672,#547,.T.);
#9826=EDGE_CURVE('',#7672,#7673,#548,.T.);
#9827=EDGE_CURVE('',#7674,#7673,#6259,.T.);
#9828=EDGE_CURVE('',#7674,#7675,#549,.T.);
#9829=EDGE_CURVE('',#7675,#7676,#550,.T.);
#9830=EDGE_CURVE('',#7677,#7676,#6260,.T.);
#9831=EDGE_CURVE('',#7677,#7445,#551,.T.);
#9832=EDGE_CURVE('',#7120,#7208,#4130,.T.);
#9833=EDGE_CURVE('',#7626,#7383,#4131,.T.);
#9834=EDGE_CURVE('',#7625,#7384,#4132,.T.);
#9835=EDGE_CURVE('',#7628,#7381,#4133,.T.);
#9836=EDGE_CURVE('',#7629,#7380,#4134,.T.);
#9837=EDGE_CURVE('',#7631,#7378,#4135,.T.);
#9838=EDGE_CURVE('',#7632,#7377,#4136,.T.);
#9839=EDGE_CURVE('',#7634,#7375,#4137,.T.);
#9840=EDGE_CURVE('',#7635,#7374,#4138,.T.);
#9841=EDGE_CURVE('',#7637,#7372,#4139,.T.);
#9842=EDGE_CURVE('',#7638,#7371,#4140,.T.);
#9843=EDGE_CURVE('',#7640,#7369,#4141,.T.);
#9844=EDGE_CURVE('',#7641,#7368,#4142,.T.);
#9845=EDGE_CURVE('',#7643,#7366,#4143,.T.);
#9846=EDGE_CURVE('',#7644,#7365,#4144,.T.);
#9847=EDGE_CURVE('',#7646,#7363,#4145,.T.);
#9848=EDGE_CURVE('',#7647,#7362,#4146,.T.);
#9849=EDGE_CURVE('',#7649,#7360,#4147,.T.);
#9850=EDGE_CURVE('',#7650,#7359,#4148,.T.);
#9851=EDGE_CURVE('',#7652,#7357,#4149,.T.);
#9852=EDGE_CURVE('',#7653,#7356,#4150,.T.);
#9853=EDGE_CURVE('',#7655,#7354,#4151,.T.);
#9854=EDGE_CURVE('',#7656,#7353,#4152,.T.);
#9855=EDGE_CURVE('',#7658,#7351,#4153,.T.);
#9856=EDGE_CURVE('',#7659,#7350,#4154,.T.);
#9857=EDGE_CURVE('',#7661,#7348,#4155,.T.);
#9858=EDGE_CURVE('',#7662,#7347,#4156,.T.);
#9859=EDGE_CURVE('',#7664,#7345,#4157,.T.);
#9860=EDGE_CURVE('',#7665,#7344,#4158,.T.);
#9861=EDGE_CURVE('',#7667,#7342,#4159,.T.);
#9862=EDGE_CURVE('',#7668,#7341,#4160,.T.);
#9863=EDGE_CURVE('',#7670,#7339,#4161,.T.);
#9864=EDGE_CURVE('',#7671,#7338,#4162,.T.);
#9865=EDGE_CURVE('',#7673,#7336,#4163,.T.);
#9866=EDGE_CURVE('',#7674,#7335,#4164,.T.);
#9867=EDGE_CURVE('',#7676,#7333,#4165,.T.);
#9868=EDGE_CURVE('',#7677,#7332,#4166,.T.);
#9869=EDGE_CURVE('',#7446,#7328,#4167,.T.);
#9870=EDGE_CURVE('',#7447,#7327,#4168,.T.);
#9871=EDGE_CURVE('',#7449,#7325,#4169,.T.);
#9872=EDGE_CURVE('',#7450,#7324,#4170,.T.);
#9873=EDGE_CURVE('',#7452,#7322,#4171,.T.);
#9874=EDGE_CURVE('',#7453,#7321,#4172,.T.);
#9875=EDGE_CURVE('',#7455,#7319,#4173,.T.);
#9876=EDGE_CURVE('',#7456,#7318,#4174,.T.);
#9877=EDGE_CURVE('',#7458,#7316,#4175,.T.);
#9878=EDGE_CURVE('',#7459,#7315,#4176,.T.);
#9879=EDGE_CURVE('',#7461,#7313,#4177,.T.);
#9880=EDGE_CURVE('',#7462,#7312,#4178,.T.);
#9881=EDGE_CURVE('',#7464,#7310,#4179,.T.);
#9882=EDGE_CURVE('',#7465,#7309,#4180,.T.);
#9883=EDGE_CURVE('',#7467,#7307,#4181,.T.);
#9884=EDGE_CURVE('',#7468,#7306,#4182,.T.);
#9885=EDGE_CURVE('',#7470,#7304,#4183,.T.);
#9886=EDGE_CURVE('',#7471,#7303,#4184,.T.);
#9887=EDGE_CURVE('',#7473,#7301,#4185,.T.);
#9888=EDGE_CURVE('',#7474,#7300,#4186,.T.);
#9889=EDGE_CURVE('',#7476,#7298,#4187,.T.);
#9890=EDGE_CURVE('',#7477,#7297,#4188,.T.);
#9891=EDGE_CURVE('',#7479,#7295,#4189,.T.);
#9892=EDGE_CURVE('',#7480,#7294,#4190,.T.);
#9893=EDGE_CURVE('',#7482,#7292,#4191,.T.);
#9894=EDGE_CURVE('',#7483,#7291,#4192,.T.);
#9895=EDGE_CURVE('',#7485,#7289,#4193,.T.);
#9896=EDGE_CURVE('',#7486,#7288,#4194,.T.);
#9897=EDGE_CURVE('',#7488,#7286,#4195,.T.);
#9898=EDGE_CURVE('',#7489,#7285,#4196,.T.);
#9899=EDGE_CURVE('',#7491,#7283,#4197,.T.);
#9900=EDGE_CURVE('',#7492,#7282,#4198,.T.);
#9901=EDGE_CURVE('',#7494,#7280,#4199,.T.);
#9902=EDGE_CURVE('',#7495,#7279,#4200,.T.);
#9903=EDGE_CURVE('',#7497,#7277,#4201,.T.);
#9904=EDGE_CURVE('',#7498,#7276,#4202,.T.);
#9905=EDGE_CURVE('',#7500,#7274,#4203,.T.);
#9906=EDGE_CURVE('',#7501,#7273,#4204,.T.);
#9907=EDGE_CURVE('',#7503,#7271,#4205,.T.);
#9908=EDGE_CURVE('',#7504,#7270,#4206,.T.);
#9909=EDGE_CURVE('',#7506,#7268,#4207,.T.);
#9910=EDGE_CURVE('',#7507,#7267,#4208,.T.);
#9911=EDGE_CURVE('',#7509,#7265,#4209,.T.);
#9912=EDGE_CURVE('',#7510,#7264,#4210,.T.);
#9913=EDGE_CURVE('',#7512,#7262,#4211,.T.);
#9914=EDGE_CURVE('',#7513,#7261,#4212,.T.);
#9915=EDGE_CURVE('',#7515,#7259,#4213,.T.);
#9916=EDGE_CURVE('',#7516,#7258,#4214,.T.);
#9917=EDGE_CURVE('',#7518,#7256,#4215,.T.);
#9918=EDGE_CURVE('',#7519,#7255,#4216,.T.);
#9919=EDGE_CURVE('',#7521,#7253,#4217,.T.);
#9920=EDGE_CURVE('',#7522,#7252,#4218,.T.);
#9921=EDGE_CURVE('',#7524,#7250,#4219,.T.);
#9922=EDGE_CURVE('',#7525,#7249,#4220,.T.);
#9923=EDGE_CURVE('',#7527,#7247,#4221,.T.);
#9924=EDGE_CURVE('',#7528,#7246,#4222,.T.);
#9925=EDGE_CURVE('',#7530,#7244,#4223,.T.);
#9926=EDGE_CURVE('',#7531,#7243,#4224,.T.);
#9927=EDGE_CURVE('',#7533,#7241,#4225,.T.);
#9928=EDGE_CURVE('',#7534,#7240,#4226,.T.);
#9929=EDGE_CURVE('',#7536,#7238,#4227,.T.);
#9930=EDGE_CURVE('',#7537,#7237,#4228,.T.);
#9931=EDGE_CURVE('',#7539,#7235,#4229,.T.);
#9932=EDGE_CURVE('',#7540,#7234,#4230,.T.);
#9933=EDGE_CURVE('',#7542,#7232,#4231,.T.);
#9934=EDGE_CURVE('',#7543,#7231,#4232,.T.);
#9935=EDGE_CURVE('',#7545,#7229,#4233,.T.);
#9936=EDGE_CURVE('',#7546,#7228,#4234,.T.);
#9937=EDGE_CURVE('',#7548,#7226,#4235,.T.);
#9938=EDGE_CURVE('',#7549,#7225,#4236,.T.);
#9939=EDGE_CURVE('',#7551,#7223,#4237,.T.);
#9940=EDGE_CURVE('',#7552,#7222,#4238,.T.);
#9941=EDGE_CURVE('',#7554,#7220,#4239,.T.);
#9942=EDGE_CURVE('',#7555,#7219,#4240,.T.);
#9943=EDGE_CURVE('',#7557,#7217,#4241,.T.);
#9944=EDGE_CURVE('',#7558,#7216,#4242,.T.);
#9945=EDGE_CURVE('',#7560,#7214,#4243,.T.);
#9946=EDGE_CURVE('',#7561,#7212,#4244,.T.);
#9947=EDGE_CURVE('',#7565,#7444,#4245,.T.);
#9948=EDGE_CURVE('',#7566,#7443,#4246,.T.);
#9949=EDGE_CURVE('',#7568,#7441,#4247,.T.);
#9950=EDGE_CURVE('',#7569,#7440,#4248,.T.);
#9951=EDGE_CURVE('',#7571,#7438,#4249,.T.);
#9952=EDGE_CURVE('',#7572,#7437,#4250,.T.);
#9953=EDGE_CURVE('',#7574,#7435,#4251,.T.);
#9954=EDGE_CURVE('',#7575,#7434,#4252,.T.);
#9955=EDGE_CURVE('',#7577,#7432,#4253,.T.);
#9956=EDGE_CURVE('',#7578,#7431,#4254,.T.);
#9957=EDGE_CURVE('',#7580,#7429,#4255,.T.);
#9958=EDGE_CURVE('',#7581,#7428,#4256,.T.);
#9959=EDGE_CURVE('',#7583,#7426,#4257,.T.);
#9960=EDGE_CURVE('',#7584,#7425,#4258,.T.);
#9961=EDGE_CURVE('',#7586,#7423,#4259,.T.);
#9962=EDGE_CURVE('',#7587,#7422,#4260,.T.);
#9963=EDGE_CURVE('',#7589,#7420,#4261,.T.);
#9964=EDGE_CURVE('',#7590,#7419,#4262,.T.);
#9965=EDGE_CURVE('',#7592,#7417,#4263,.T.);
#9966=EDGE_CURVE('',#7593,#7416,#4264,.T.);
#9967=EDGE_CURVE('',#7595,#7414,#4265,.T.);
#9968=EDGE_CURVE('',#7596,#7413,#4266,.T.);
#9969=EDGE_CURVE('',#7598,#7411,#4267,.T.);
#9970=EDGE_CURVE('',#7599,#7410,#4268,.T.);
#9971=EDGE_CURVE('',#7601,#7408,#4269,.T.);
#9972=EDGE_CURVE('',#7602,#7407,#4270,.T.);
#9973=EDGE_CURVE('',#7604,#7405,#4271,.T.);
#9974=EDGE_CURVE('',#7605,#7404,#4272,.T.);
#9975=EDGE_CURVE('',#7607,#7402,#4273,.T.);
#9976=EDGE_CURVE('',#7608,#7401,#4274,.T.);
#9977=EDGE_CURVE('',#7610,#7399,#4275,.T.);
#9978=EDGE_CURVE('',#7611,#7398,#4276,.T.);
#9979=EDGE_CURVE('',#7613,#7396,#4277,.T.);
#9980=EDGE_CURVE('',#7614,#7395,#4278,.T.);
#9981=EDGE_CURVE('',#7616,#7393,#4279,.T.);
#9982=EDGE_CURVE('',#7617,#7392,#4280,.T.);
#9983=EDGE_CURVE('',#7623,#7386,#4281,.T.);
#9984=EDGE_CURVE('',#7622,#7387,#4282,.T.);
#9985=EDGE_CURVE('',#7619,#7390,#4283,.T.);
#9986=EDGE_CURVE('',#7620,#7389,#4284,.T.);
#9987=EDGE_CURVE('',#7621,#7388,#4285,.T.);
#9988=EDGE_CURVE('',#7624,#7385,#4286,.T.);
#9989=EDGE_CURVE('',#7618,#7391,#4287,.T.);
#9990=EDGE_CURVE('',#7615,#7394,#4288,.T.);
#9991=EDGE_CURVE('',#7612,#7397,#4289,.T.);
#9992=EDGE_CURVE('',#7609,#7400,#4290,.T.);
#9993=EDGE_CURVE('',#7606,#7403,#4291,.T.);
#9994=EDGE_CURVE('',#7603,#7406,#4292,.T.);
#9995=EDGE_CURVE('',#7600,#7409,#4293,.T.);
#9996=EDGE_CURVE('',#7597,#7412,#4294,.T.);
#9997=EDGE_CURVE('',#7594,#7415,#4295,.T.);
#9998=EDGE_CURVE('',#7591,#7418,#4296,.T.);
#9999=EDGE_CURVE('',#7588,#7421,#4297,.T.);
#10000=EDGE_CURVE('',#7585,#7424,#4298,.T.);
#10001=EDGE_CURVE('',#7582,#7427,#4299,.T.);
#10002=EDGE_CURVE('',#7579,#7430,#4300,.T.);
#10003=EDGE_CURVE('',#7576,#7433,#4301,.T.);
#10004=EDGE_CURVE('',#7573,#7436,#4302,.T.);
#10005=EDGE_CURVE('',#7570,#7439,#4303,.T.);
#10006=EDGE_CURVE('',#7567,#7442,#4304,.T.);
#10007=EDGE_CURVE('',#7564,#7213,#4305,.T.);
#10008=EDGE_CURVE('',#7559,#7215,#4306,.T.);
#10009=EDGE_CURVE('',#7556,#7218,#4307,.T.);
#10010=EDGE_CURVE('',#7553,#7221,#4308,.T.);
#10011=EDGE_CURVE('',#7550,#7224,#4309,.T.);
#10012=EDGE_CURVE('',#7547,#7227,#4310,.T.);
#10013=EDGE_CURVE('',#7544,#7230,#4311,.T.);
#10014=EDGE_CURVE('',#7541,#7233,#4312,.T.);
#10015=EDGE_CURVE('',#7538,#7236,#4313,.T.);
#10016=EDGE_CURVE('',#7535,#7239,#4314,.T.);
#10017=EDGE_CURVE('',#7532,#7242,#4315,.T.);
#10018=EDGE_CURVE('',#7529,#7245,#4316,.T.);
#10019=EDGE_CURVE('',#7526,#7248,#4317,.T.);
#10020=EDGE_CURVE('',#7523,#7251,#4318,.T.);
#10021=EDGE_CURVE('',#7520,#7254,#4319,.T.);
#10022=EDGE_CURVE('',#7517,#7257,#4320,.T.);
#10023=EDGE_CURVE('',#7514,#7260,#4321,.T.);
#10024=EDGE_CURVE('',#7511,#7263,#4322,.T.);
#10025=EDGE_CURVE('',#7508,#7266,#4323,.T.);
#10026=EDGE_CURVE('',#7505,#7269,#4324,.T.);
#10027=EDGE_CURVE('',#7502,#7272,#4325,.T.);
#10028=EDGE_CURVE('',#7499,#7275,#4326,.T.);
#10029=EDGE_CURVE('',#7496,#7278,#4327,.T.);
#10030=EDGE_CURVE('',#7493,#7281,#4328,.T.);
#10031=EDGE_CURVE('',#7490,#7284,#4329,.T.);
#10032=EDGE_CURVE('',#7487,#7287,#4330,.T.);
#10033=EDGE_CURVE('',#7484,#7290,#4331,.T.);
#10034=EDGE_CURVE('',#7481,#7293,#4332,.T.);
#10035=EDGE_CURVE('',#7478,#7296,#4333,.T.);
#10036=EDGE_CURVE('',#7475,#7299,#4334,.T.);
#10037=EDGE_CURVE('',#7472,#7302,#4335,.T.);
#10038=EDGE_CURVE('',#7469,#7305,#4336,.T.);
#10039=EDGE_CURVE('',#7466,#7308,#4337,.T.);
#10040=EDGE_CURVE('',#7463,#7311,#4338,.T.);
#10041=EDGE_CURVE('',#7460,#7314,#4339,.T.);
#10042=EDGE_CURVE('',#7457,#7317,#4340,.T.);
#10043=EDGE_CURVE('',#7454,#7320,#4341,.T.);
#10044=EDGE_CURVE('',#7451,#7323,#4342,.T.);
#10045=EDGE_CURVE('',#7448,#7326,#4343,.T.);
#10046=EDGE_CURVE('',#7445,#7331,#4344,.T.);
#10047=EDGE_CURVE('',#7675,#7334,#4345,.T.);
#10048=EDGE_CURVE('',#7672,#7337,#4346,.T.);
#10049=EDGE_CURVE('',#7669,#7340,#4347,.T.);
#10050=EDGE_CURVE('',#7666,#7343,#4348,.T.);
#10051=EDGE_CURVE('',#7663,#7346,#4349,.T.);
#10052=EDGE_CURVE('',#7660,#7349,#4350,.T.);
#10053=EDGE_CURVE('',#7657,#7352,#4351,.T.);
#10054=EDGE_CURVE('',#7654,#7355,#4352,.T.);
#10055=EDGE_CURVE('',#7651,#7358,#4353,.T.);
#10056=EDGE_CURVE('',#7648,#7361,#4354,.T.);
#10057=EDGE_CURVE('',#7645,#7364,#4355,.T.);
#10058=EDGE_CURVE('',#7642,#7367,#4356,.T.);
#10059=EDGE_CURVE('',#7639,#7370,#4357,.T.);
#10060=EDGE_CURVE('',#7636,#7373,#4358,.T.);
#10061=EDGE_CURVE('',#7633,#7376,#4359,.T.);
#10062=EDGE_CURVE('',#7630,#7379,#4360,.T.);
#10063=EDGE_CURVE('',#7627,#7382,#4361,.T.);
#10064=EDGE_CURVE('',#7678,#7679,#6261,.T.);
#10065=EDGE_CURVE('',#7680,#7679,#1014,.T.);
#10066=EDGE_CURVE('',#7681,#7680,#6262,.T.);
#10067=EDGE_CURVE('',#7682,#7681,#1015,.T.);
#10068=EDGE_CURVE('',#7682,#7683,#6263,.T.);
#10069=EDGE_CURVE('',#7683,#7684,#6264,.T.);
#10070=EDGE_CURVE('',#7685,#7684,#6265,.T.);
#10071=EDGE_CURVE('',#7684,#7685,#6266,.T.);
#10072=EDGE_CURVE('',#7683,#7686,#6267,.T.);
#10073=EDGE_CURVE('',#7687,#7686,#1016,.T.);
#10074=EDGE_CURVE('',#7688,#7687,#6268,.T.);
#10075=EDGE_CURVE('',#7678,#7688,#1017,.T.);
#10076=EDGE_CURVE('',#7689,#7689,#6269,.T.);
#10077=EDGE_CURVE('',#7689,#7685,#4362,.T.);
#10078=EDGE_CURVE('',#7690,#7690,#6270,.T.);
#10079=EDGE_CURVE('',#7690,#7691,#4363,.T.);
#10080=EDGE_CURVE('',#7691,#7691,#6271,.T.);
#10081=EDGE_CURVE('',#7688,#7687,#4364,.T.);
#10082=EDGE_CURVE('',#7681,#7680,#4365,.T.);
#10083=EDGE_CURVE('',#7678,#7686,#4366,.T.);
#10084=EDGE_CURVE('',#7682,#7679,#4367,.T.);
#10085=EDGE_CURVE('',#7692,#7692,#6272,.T.);
#10086=EDGE_CURVE('',#7692,#7693,#6273,.T.);
#10087=EDGE_CURVE('',#7693,#7693,#6274,.T.);
#10088=EDGE_CURVE('',#7694,#7695,#6275,.T.);
#10089=EDGE_CURVE('',#7695,#7694,#6276,.T.);
#10090=EDGE_CURVE('',#7695,#7696,#4368,.T.);
#10091=EDGE_CURVE('',#7696,#7696,#6277,.T.);
#10092=EDGE_CURVE('',#7697,#7698,#6278,.T.);
#10093=EDGE_CURVE('',#7698,#7697,#6279,.T.);
#10094=EDGE_CURVE('',#7698,#7699,#4369,.T.);
#10095=EDGE_CURVE('',#7699,#7700,#6280,.T.);
#10096=EDGE_CURVE('',#7700,#7699,#6281,.T.);
#10097=EDGE_CURVE('',#7694,#7700,#4370,.T.);
#10098=EDGE_CURVE('',#7701,#7702,#6282,.T.);
#10099=EDGE_CURVE('',#7702,#7701,#6283,.T.);
#10100=EDGE_CURVE('',#7702,#7697,#4371,.T.);
#10101=EDGE_CURVE('',#7703,#7704,#6284,.T.);
#10102=EDGE_CURVE('',#7704,#7703,#6285,.T.);
#10103=EDGE_CURVE('',#7704,#7705,#4372,.T.);
#10104=EDGE_CURVE('',#7705,#7706,#6286,.T.);
#10105=EDGE_CURVE('',#7706,#7705,#6287,.T.);
#10106=EDGE_CURVE('',#7701,#7706,#4373,.T.);
#10107=EDGE_CURVE('',#7707,#7708,#6288,.T.);
#10108=EDGE_CURVE('',#7708,#7707,#6289,.T.);
#10109=EDGE_CURVE('',#7708,#7703,#4374,.T.);
#10110=EDGE_CURVE('',#7709,#7710,#6290,.T.);
#10111=EDGE_CURVE('',#7710,#7709,#6291,.T.);
#10112=EDGE_CURVE('',#7710,#7711,#4375,.T.);
#10113=EDGE_CURVE('',#7711,#7712,#6292,.T.);
#10114=EDGE_CURVE('',#7712,#7711,#6293,.T.);
#10115=EDGE_CURVE('',#7707,#7712,#4376,.T.);
#10116=EDGE_CURVE('',#7713,#7714,#6294,.T.);
#10117=EDGE_CURVE('',#7714,#7713,#6295,.T.);
#10118=EDGE_CURVE('',#7714,#7709,#4377,.T.);
#10119=EDGE_CURVE('',#7715,#7716,#6296,.T.);
#10120=EDGE_CURVE('',#7716,#7715,#6297,.T.);
#10121=EDGE_CURVE('',#7716,#7717,#4378,.T.);
#10122=EDGE_CURVE('',#7717,#7718,#6298,.T.);
#10123=EDGE_CURVE('',#7718,#7717,#6299,.T.);
#10124=EDGE_CURVE('',#7713,#7718,#4379,.T.);
#10125=EDGE_CURVE('',#7719,#7720,#6300,.T.);
#10126=EDGE_CURVE('',#7720,#7719,#6301,.T.);
#10127=EDGE_CURVE('',#7720,#7715,#4380,.T.);
#10128=EDGE_CURVE('',#7721,#7722,#6302,.T.);
#10129=EDGE_CURVE('',#7722,#7721,#6303,.T.);
#10130=EDGE_CURVE('',#7722,#7723,#4381,.T.);
#10131=EDGE_CURVE('',#7723,#7724,#6304,.T.);
#10132=EDGE_CURVE('',#7724,#7723,#6305,.T.);
#10133=EDGE_CURVE('',#7719,#7724,#4382,.T.);
#10134=EDGE_CURVE('',#7725,#7726,#6306,.T.);
#10135=EDGE_CURVE('',#7726,#7725,#6307,.T.);
#10136=EDGE_CURVE('',#7726,#7721,#4383,.T.);
#10137=EDGE_CURVE('',#7727,#7728,#6308,.T.);
#10138=EDGE_CURVE('',#7728,#7727,#6309,.T.);
#10139=EDGE_CURVE('',#7728,#7729,#4384,.T.);
#10140=EDGE_CURVE('',#7729,#7730,#6310,.T.);
#10141=EDGE_CURVE('',#7730,#7729,#6311,.T.);
#10142=EDGE_CURVE('',#7725,#7730,#4385,.T.);
#10143=EDGE_CURVE('',#7731,#7732,#6312,.T.);
#10144=EDGE_CURVE('',#7732,#7731,#6313,.T.);
#10145=EDGE_CURVE('',#7732,#7727,#4386,.T.);
#10146=EDGE_CURVE('',#7733,#7734,#6314,.T.);
#10147=EDGE_CURVE('',#7734,#7733,#6315,.T.);
#10148=EDGE_CURVE('',#7734,#7735,#4387,.T.);
#10149=EDGE_CURVE('',#7735,#7736,#6316,.T.);
#10150=EDGE_CURVE('',#7736,#7735,#6317,.T.);
#10151=EDGE_CURVE('',#7731,#7736,#4388,.T.);
#10152=EDGE_CURVE('',#7737,#7738,#6318,.T.);
#10153=EDGE_CURVE('',#7738,#7737,#6319,.T.);
#10154=EDGE_CURVE('',#7738,#7733,#4389,.T.);
#10155=EDGE_CURVE('',#7739,#7740,#6320,.T.);
#10156=EDGE_CURVE('',#7740,#7739,#6321,.T.);
#10157=EDGE_CURVE('',#7740,#7741,#4390,.T.);
#10158=EDGE_CURVE('',#7741,#7742,#6322,.T.);
#10159=EDGE_CURVE('',#7742,#7741,#6323,.T.);
#10160=EDGE_CURVE('',#7737,#7742,#4391,.T.);
#10161=EDGE_CURVE('',#7743,#7744,#6324,.T.);
#10162=EDGE_CURVE('',#7744,#7743,#6325,.T.);
#10163=EDGE_CURVE('',#7744,#7739,#4392,.T.);
#10164=EDGE_CURVE('',#7745,#7746,#6326,.T.);
#10165=EDGE_CURVE('',#7746,#7745,#6327,.T.);
#10166=EDGE_CURVE('',#7746,#7747,#4393,.T.);
#10167=EDGE_CURVE('',#7747,#7748,#6328,.T.);
#10168=EDGE_CURVE('',#7748,#7747,#6329,.T.);
#10169=EDGE_CURVE('',#7743,#7748,#4394,.T.);
#10170=EDGE_CURVE('',#7749,#7750,#6330,.T.);
#10171=EDGE_CURVE('',#7750,#7749,#6331,.T.);
#10172=EDGE_CURVE('',#7750,#7745,#4395,.T.);
#10173=EDGE_CURVE('',#7751,#7752,#6332,.T.);
#10174=EDGE_CURVE('',#7752,#7751,#6333,.T.);
#10175=EDGE_CURVE('',#7752,#7753,#4396,.T.);
#10176=EDGE_CURVE('',#7753,#7754,#6334,.T.);
#10177=EDGE_CURVE('',#7754,#7753,#6335,.T.);
#10178=EDGE_CURVE('',#7749,#7754,#4397,.T.);
#10179=EDGE_CURVE('',#7755,#7756,#6336,.T.);
#10180=EDGE_CURVE('',#7756,#7755,#6337,.T.);
#10181=EDGE_CURVE('',#7756,#7751,#4398,.T.);
#10182=EDGE_CURVE('',#7757,#7758,#6338,.T.);
#10183=EDGE_CURVE('',#7758,#7757,#6339,.T.);
#10184=EDGE_CURVE('',#7758,#7759,#4399,.T.);
#10185=EDGE_CURVE('',#7759,#7760,#6340,.T.);
#10186=EDGE_CURVE('',#7760,#7759,#6341,.T.);
#10187=EDGE_CURVE('',#7755,#7760,#4400,.T.);
#10188=EDGE_CURVE('',#7761,#7762,#6342,.T.);
#10189=EDGE_CURVE('',#7762,#7761,#6343,.T.);
#10190=EDGE_CURVE('',#7762,#7757,#4401,.T.);
#10191=EDGE_CURVE('',#7763,#7764,#6344,.T.);
#10192=EDGE_CURVE('',#7764,#7763,#6345,.T.);
#10193=EDGE_CURVE('',#7764,#7765,#4402,.T.);
#10194=EDGE_CURVE('',#7765,#7766,#6346,.T.);
#10195=EDGE_CURVE('',#7766,#7765,#6347,.T.);
#10196=EDGE_CURVE('',#7761,#7766,#4403,.T.);
#10197=EDGE_CURVE('',#7767,#7768,#6348,.T.);
#10198=EDGE_CURVE('',#7768,#7767,#6349,.T.);
#10199=EDGE_CURVE('',#7768,#7763,#4404,.T.);
#10200=EDGE_CURVE('',#7769,#7770,#6350,.T.);
#10201=EDGE_CURVE('',#7770,#7769,#6351,.T.);
#10202=EDGE_CURVE('',#7770,#7771,#4405,.T.);
#10203=EDGE_CURVE('',#7771,#7772,#6352,.T.);
#10204=EDGE_CURVE('',#7772,#7771,#6353,.T.);
#10205=EDGE_CURVE('',#7767,#7772,#4406,.T.);
#10206=EDGE_CURVE('',#7693,#7773,#4407,.T.);
#10207=EDGE_CURVE('',#7773,#7773,#6354,.T.);
#10208=EDGE_CURVE('',#7774,#7775,#552,.F.);
#10209=EDGE_CURVE('',#7776,#7775,#6355,.T.);
#10210=EDGE_CURVE('',#7776,#7777,#553,.T.);
#10211=EDGE_CURVE('',#7777,#7778,#554,.T.);
#10212=EDGE_CURVE('',#7779,#7778,#6356,.T.);
#10213=EDGE_CURVE('',#7779,#7780,#555,.T.);
#10214=EDGE_CURVE('',#7780,#7781,#556,.T.);
#10215=EDGE_CURVE('',#7782,#7781,#6357,.T.);
#10216=EDGE_CURVE('',#7782,#7783,#557,.T.);
#10217=EDGE_CURVE('',#7783,#7784,#558,.T.);
#10218=EDGE_CURVE('',#7785,#7784,#6358,.T.);
#10219=EDGE_CURVE('',#7785,#7786,#559,.T.);
#10220=EDGE_CURVE('',#7786,#7787,#560,.T.);
#10221=EDGE_CURVE('',#7788,#7787,#6359,.T.);
#10222=EDGE_CURVE('',#7788,#7789,#561,.T.);
#10223=EDGE_CURVE('',#7789,#7790,#562,.T.);
#10224=EDGE_CURVE('',#7791,#7790,#6360,.T.);
#10225=EDGE_CURVE('',#7791,#7792,#563,.T.);
#10226=EDGE_CURVE('',#7792,#7793,#564,.T.);
#10227=EDGE_CURVE('',#7794,#7793,#6361,.T.);
#10228=EDGE_CURVE('',#7794,#7795,#565,.T.);
#10229=EDGE_CURVE('',#7795,#7796,#566,.T.);
#10230=EDGE_CURVE('',#7797,#7796,#6362,.T.);
#10231=EDGE_CURVE('',#7797,#7798,#567,.T.);
#10232=EDGE_CURVE('',#7798,#7799,#568,.T.);
#10233=EDGE_CURVE('',#7800,#7799,#6363,.T.);
#10234=EDGE_CURVE('',#7800,#7801,#569,.T.);
#10235=EDGE_CURVE('',#7801,#7802,#570,.T.);
#10236=EDGE_CURVE('',#7803,#7802,#6364,.T.);
#10237=EDGE_CURVE('',#7803,#7804,#571,.T.);
#10238=EDGE_CURVE('',#7804,#7805,#572,.T.);
#10239=EDGE_CURVE('',#7806,#7805,#6365,.T.);
#10240=EDGE_CURVE('',#7806,#7807,#573,.T.);
#10241=EDGE_CURVE('',#7807,#7808,#574,.T.);
#10242=EDGE_CURVE('',#7809,#7808,#6366,.T.);
#10243=EDGE_CURVE('',#7809,#7810,#575,.T.);
#10244=EDGE_CURVE('',#7810,#7811,#576,.T.);
#10245=EDGE_CURVE('',#7812,#7811,#6367,.T.);
#10246=EDGE_CURVE('',#7812,#7813,#577,.T.);
#10247=EDGE_CURVE('',#7813,#7814,#578,.T.);
#10248=EDGE_CURVE('',#7815,#7814,#6368,.T.);
#10249=EDGE_CURVE('',#7815,#7816,#579,.T.);
#10250=EDGE_CURVE('',#7816,#7817,#580,.T.);
#10251=EDGE_CURVE('',#7818,#7817,#6369,.T.);
#10252=EDGE_CURVE('',#7818,#7819,#581,.T.);
#10253=EDGE_CURVE('',#7819,#7820,#582,.T.);
#10254=EDGE_CURVE('',#7821,#7820,#6370,.T.);
#10255=EDGE_CURVE('',#7821,#7822,#583,.T.);
#10256=EDGE_CURVE('',#7822,#7823,#584,.T.);
#10257=EDGE_CURVE('',#7824,#7823,#6371,.T.);
#10258=EDGE_CURVE('',#7824,#7825,#585,.T.);
#10259=EDGE_CURVE('',#7825,#7826,#586,.T.);
#10260=EDGE_CURVE('',#7827,#7826,#6372,.T.);
#10261=EDGE_CURVE('',#7827,#7828,#587,.T.);
#10262=EDGE_CURVE('',#7828,#7829,#588,.T.);
#10263=EDGE_CURVE('',#7830,#7829,#6373,.T.);
#10264=EDGE_CURVE('',#7830,#7831,#589,.T.);
#10265=EDGE_CURVE('',#7831,#7832,#590,.T.);
#10266=EDGE_CURVE('',#7833,#7832,#6374,.T.);
#10267=EDGE_CURVE('',#7833,#7834,#591,.T.);
#10268=EDGE_CURVE('',#7834,#7835,#592,.T.);
#10269=EDGE_CURVE('',#7836,#7835,#6375,.T.);
#10270=EDGE_CURVE('',#7836,#7837,#593,.T.);
#10271=EDGE_CURVE('',#7837,#7838,#594,.T.);
#10272=EDGE_CURVE('',#7839,#7838,#6376,.T.);
#10273=EDGE_CURVE('',#7839,#7840,#595,.T.);
#10274=EDGE_CURVE('',#7840,#7841,#596,.T.);
#10275=EDGE_CURVE('',#7842,#7841,#6377,.T.);
#10276=EDGE_CURVE('',#7842,#7843,#597,.T.);
#10277=EDGE_CURVE('',#7843,#7844,#598,.T.);
#10278=EDGE_CURVE('',#7845,#7844,#6378,.T.);
#10279=EDGE_CURVE('',#7845,#7846,#599,.T.);
#10280=EDGE_CURVE('',#7846,#7847,#600,.T.);
#10281=EDGE_CURVE('',#7848,#7847,#6379,.T.);
#10282=EDGE_CURVE('',#7848,#7849,#601,.T.);
#10283=EDGE_CURVE('',#7849,#7850,#602,.T.);
#10284=EDGE_CURVE('',#7851,#7850,#6380,.T.);
#10285=EDGE_CURVE('',#7851,#7852,#603,.T.);
#10286=EDGE_CURVE('',#7852,#7853,#604,.T.);
#10287=EDGE_CURVE('',#7854,#7853,#6381,.T.);
#10288=EDGE_CURVE('',#7854,#7855,#605,.T.);
#10289=EDGE_CURVE('',#7855,#7856,#606,.T.);
#10290=EDGE_CURVE('',#7857,#7856,#6382,.T.);
#10291=EDGE_CURVE('',#7857,#7858,#607,.T.);
#10292=EDGE_CURVE('',#7858,#7859,#608,.T.);
#10293=EDGE_CURVE('',#7860,#7859,#6383,.T.);
#10294=EDGE_CURVE('',#7860,#7861,#609,.T.);
#10295=EDGE_CURVE('',#7861,#7862,#610,.T.);
#10296=EDGE_CURVE('',#7863,#7862,#6384,.T.);
#10297=EDGE_CURVE('',#7863,#7864,#611,.T.);
#10298=EDGE_CURVE('',#7864,#7865,#612,.T.);
#10299=EDGE_CURVE('',#7866,#7865,#6385,.T.);
#10300=EDGE_CURVE('',#7866,#7867,#613,.T.);
#10301=EDGE_CURVE('',#7867,#7868,#614,.T.);
#10302=EDGE_CURVE('',#7869,#7868,#6386,.T.);
#10303=EDGE_CURVE('',#7869,#7870,#615,.T.);
#10304=EDGE_CURVE('',#7870,#7871,#616,.T.);
#10305=EDGE_CURVE('',#7872,#7871,#6387,.T.);
#10306=EDGE_CURVE('',#7872,#7873,#617,.T.);
#10307=EDGE_CURVE('',#7873,#7874,#618,.T.);
#10308=EDGE_CURVE('',#7875,#7874,#6388,.T.);
#10309=EDGE_CURVE('',#7875,#7876,#619,.T.);
#10310=EDGE_CURVE('',#7876,#7877,#620,.T.);
#10311=EDGE_CURVE('',#7878,#7877,#6389,.T.);
#10312=EDGE_CURVE('',#7878,#7879,#621,.T.);
#10313=EDGE_CURVE('',#7879,#7880,#622,.T.);
#10314=EDGE_CURVE('',#7881,#7880,#6390,.T.);
#10315=EDGE_CURVE('',#7881,#7882,#623,.T.);
#10316=EDGE_CURVE('',#7882,#7883,#624,.T.);
#10317=EDGE_CURVE('',#7884,#7883,#6391,.T.);
#10318=EDGE_CURVE('',#7884,#7885,#625,.T.);
#10319=EDGE_CURVE('',#7885,#7886,#626,.T.);
#10320=EDGE_CURVE('',#7887,#7886,#6392,.T.);
#10321=EDGE_CURVE('',#7887,#7888,#627,.T.);
#10322=EDGE_CURVE('',#7888,#7889,#628,.T.);
#10323=EDGE_CURVE('',#7890,#7889,#6393,.T.);
#10324=EDGE_CURVE('',#7890,#7891,#629,.T.);
#10325=EDGE_CURVE('',#7891,#7892,#4408,.T.);
#10326=EDGE_CURVE('',#7892,#7892,#6394,.T.);
#10327=EDGE_CURVE('',#7891,#7893,#630,.T.);
#10328=EDGE_CURVE('',#7893,#7894,#631,.T.);
#10329=EDGE_CURVE('',#7895,#7894,#6395,.T.);
#10330=EDGE_CURVE('',#7895,#7896,#632,.T.);
#10331=EDGE_CURVE('',#7896,#7897,#633,.T.);
#10332=EDGE_CURVE('',#7898,#7897,#6396,.T.);
#10333=EDGE_CURVE('',#7898,#7899,#634,.T.);
#10334=EDGE_CURVE('',#7899,#7900,#635,.T.);
#10335=EDGE_CURVE('',#7901,#7900,#6397,.T.);
#10336=EDGE_CURVE('',#7901,#7902,#636,.T.);
#10337=EDGE_CURVE('',#7902,#7903,#637,.T.);
#10338=EDGE_CURVE('',#7904,#7903,#6398,.T.);
#10339=EDGE_CURVE('',#7904,#7905,#638,.T.);
#10340=EDGE_CURVE('',#7905,#7906,#639,.T.);
#10341=EDGE_CURVE('',#7907,#7906,#6399,.T.);
#10342=EDGE_CURVE('',#7907,#7908,#640,.T.);
#10343=EDGE_CURVE('',#7908,#7909,#641,.T.);
#10344=EDGE_CURVE('',#7910,#7909,#6400,.T.);
#10345=EDGE_CURVE('',#7910,#7911,#642,.T.);
#10346=EDGE_CURVE('',#7911,#7912,#643,.T.);
#10347=EDGE_CURVE('',#7913,#7912,#6401,.T.);
#10348=EDGE_CURVE('',#7913,#7914,#644,.T.);
#10349=EDGE_CURVE('',#7914,#7915,#645,.T.);
#10350=EDGE_CURVE('',#7916,#7915,#6402,.T.);
#10351=EDGE_CURVE('',#7916,#7917,#646,.T.);
#10352=EDGE_CURVE('',#7917,#7918,#647,.T.);
#10353=EDGE_CURVE('',#7919,#7918,#6403,.T.);
#10354=EDGE_CURVE('',#7919,#7920,#648,.T.);
#10355=EDGE_CURVE('',#7920,#7921,#649,.T.);
#10356=EDGE_CURVE('',#7922,#7921,#6404,.T.);
#10357=EDGE_CURVE('',#7922,#7923,#650,.T.);
#10358=EDGE_CURVE('',#7923,#7924,#651,.T.);
#10359=EDGE_CURVE('',#7925,#7924,#6405,.T.);
#10360=EDGE_CURVE('',#7925,#7926,#652,.T.);
#10361=EDGE_CURVE('',#7926,#7927,#653,.T.);
#10362=EDGE_CURVE('',#7928,#7927,#6406,.T.);
#10363=EDGE_CURVE('',#7928,#7929,#654,.T.);
#10364=EDGE_CURVE('',#7929,#7930,#655,.T.);
#10365=EDGE_CURVE('',#7931,#7930,#6407,.T.);
#10366=EDGE_CURVE('',#7931,#7932,#656,.T.);
#10367=EDGE_CURVE('',#7932,#7933,#657,.T.);
#10368=EDGE_CURVE('',#7934,#7933,#6408,.T.);
#10369=EDGE_CURVE('',#7934,#7935,#658,.T.);
#10370=EDGE_CURVE('',#7935,#7936,#659,.T.);
#10371=EDGE_CURVE('',#7937,#7936,#6409,.T.);
#10372=EDGE_CURVE('',#7937,#7938,#660,.T.);
#10373=EDGE_CURVE('',#7938,#7939,#661,.T.);
#10374=EDGE_CURVE('',#7940,#7939,#6410,.T.);
#10375=EDGE_CURVE('',#7940,#7941,#662,.T.);
#10376=EDGE_CURVE('',#7941,#7942,#663,.T.);
#10377=EDGE_CURVE('',#7943,#7942,#6411,.T.);
#10378=EDGE_CURVE('',#7943,#7944,#664,.T.);
#10379=EDGE_CURVE('',#7944,#7945,#665,.T.);
#10380=EDGE_CURVE('',#7946,#7945,#6412,.T.);
#10381=EDGE_CURVE('',#7946,#7947,#666,.T.);
#10382=EDGE_CURVE('',#7947,#7948,#667,.T.);
#10383=EDGE_CURVE('',#7949,#7948,#6413,.T.);
#10384=EDGE_CURVE('',#7949,#7950,#668,.T.);
#10385=EDGE_CURVE('',#7950,#7951,#669,.T.);
#10386=EDGE_CURVE('',#7952,#7951,#6414,.T.);
#10387=EDGE_CURVE('',#7952,#7953,#670,.T.);
#10388=EDGE_CURVE('',#7953,#7954,#671,.T.);
#10389=EDGE_CURVE('',#7955,#7954,#6415,.T.);
#10390=EDGE_CURVE('',#7955,#7956,#672,.T.);
#10391=EDGE_CURVE('',#7956,#7957,#673,.T.);
#10392=EDGE_CURVE('',#7958,#7957,#6416,.T.);
#10393=EDGE_CURVE('',#7958,#7959,#674,.T.);
#10394=EDGE_CURVE('',#7959,#7960,#675,.T.);
#10395=EDGE_CURVE('',#7961,#7960,#6417,.T.);
#10396=EDGE_CURVE('',#7961,#7962,#676,.T.);
#10397=EDGE_CURVE('',#7962,#7963,#677,.T.);
#10398=EDGE_CURVE('',#7964,#7963,#6418,.T.);
#10399=EDGE_CURVE('',#7964,#7965,#678,.T.);
#10400=EDGE_CURVE('',#7965,#7966,#679,.T.);
#10401=EDGE_CURVE('',#7967,#7966,#6419,.T.);
#10402=EDGE_CURVE('',#7967,#7968,#680,.T.);
#10403=EDGE_CURVE('',#7968,#7969,#681,.T.);
#10404=EDGE_CURVE('',#7970,#7969,#6420,.T.);
#10405=EDGE_CURVE('',#7970,#7971,#682,.T.);
#10406=EDGE_CURVE('',#7971,#7972,#683,.T.);
#10407=EDGE_CURVE('',#7973,#7972,#6421,.T.);
#10408=EDGE_CURVE('',#7973,#7974,#684,.T.);
#10409=EDGE_CURVE('',#7974,#7975,#685,.T.);
#10410=EDGE_CURVE('',#7976,#7975,#6422,.T.);
#10411=EDGE_CURVE('',#7976,#7977,#686,.T.);
#10412=EDGE_CURVE('',#7977,#7978,#687,.T.);
#10413=EDGE_CURVE('',#7979,#7978,#6423,.T.);
#10414=EDGE_CURVE('',#7979,#7980,#688,.T.);
#10415=EDGE_CURVE('',#7980,#7981,#689,.T.);
#10416=EDGE_CURVE('',#7982,#7981,#6424,.T.);
#10417=EDGE_CURVE('',#7982,#7983,#690,.T.);
#10418=EDGE_CURVE('',#7983,#7984,#691,.T.);
#10419=EDGE_CURVE('',#7985,#7984,#6425,.T.);
#10420=EDGE_CURVE('',#7985,#7986,#692,.T.);
#10421=EDGE_CURVE('',#7986,#7987,#693,.T.);
#10422=EDGE_CURVE('',#7988,#7987,#6426,.T.);
#10423=EDGE_CURVE('',#7988,#7989,#694,.T.);
#10424=EDGE_CURVE('',#7989,#7990,#695,.T.);
#10425=EDGE_CURVE('',#7991,#7990,#6427,.T.);
#10426=EDGE_CURVE('',#7991,#7992,#696,.T.);
#10427=EDGE_CURVE('',#7992,#7993,#697,.T.);
#10428=EDGE_CURVE('',#7994,#7993,#6428,.T.);
#10429=EDGE_CURVE('',#7994,#7995,#698,.T.);
#10430=EDGE_CURVE('',#7995,#7996,#699,.T.);
#10431=EDGE_CURVE('',#7997,#7996,#6429,.T.);
#10432=EDGE_CURVE('',#7997,#7998,#700,.T.);
#10433=EDGE_CURVE('',#7998,#7999,#701,.T.);
#10434=EDGE_CURVE('',#8000,#7999,#6430,.T.);
#10435=EDGE_CURVE('',#8000,#8001,#702,.T.);
#10436=EDGE_CURVE('',#8001,#8002,#703,.T.);
#10437=EDGE_CURVE('',#8003,#8002,#6431,.T.);
#10438=EDGE_CURVE('',#8003,#8004,#704,.T.);
#10439=EDGE_CURVE('',#8004,#8005,#705,.T.);
#10440=EDGE_CURVE('',#8006,#8005,#6432,.T.);
#10441=EDGE_CURVE('',#8006,#7774,#706,.T.);
#10442=EDGE_CURVE('',#8007,#8008,#707,.T.);
#10443=EDGE_CURVE('',#8007,#8009,#6433,.T.);
#10444=EDGE_CURVE('',#8010,#8009,#708,.T.);
#10445=EDGE_CURVE('',#8011,#8010,#709,.T.);
#10446=EDGE_CURVE('',#8011,#8012,#6434,.T.);
#10447=EDGE_CURVE('',#8013,#8012,#710,.T.);
#10448=EDGE_CURVE('',#8014,#8013,#711,.T.);
#10449=EDGE_CURVE('',#8014,#8015,#6435,.T.);
#10450=EDGE_CURVE('',#8016,#8015,#712,.T.);
#10451=EDGE_CURVE('',#8017,#8016,#713,.T.);
#10452=EDGE_CURVE('',#8017,#8018,#6436,.T.);
#10453=EDGE_CURVE('',#8019,#8018,#714,.T.);
#10454=EDGE_CURVE('',#8020,#8019,#715,.T.);
#10455=EDGE_CURVE('',#8020,#8021,#6437,.T.);
#10456=EDGE_CURVE('',#8022,#8021,#716,.T.);
#10457=EDGE_CURVE('',#8023,#8022,#717,.T.);
#10458=EDGE_CURVE('',#8023,#8024,#6438,.T.);
#10459=EDGE_CURVE('',#8025,#8024,#718,.T.);
#10460=EDGE_CURVE('',#8026,#8025,#719,.T.);
#10461=EDGE_CURVE('',#8026,#8027,#6439,.T.);
#10462=EDGE_CURVE('',#8028,#8027,#720,.T.);
#10463=EDGE_CURVE('',#8029,#8028,#721,.T.);
#10464=EDGE_CURVE('',#8029,#8030,#6440,.T.);
#10465=EDGE_CURVE('',#8031,#8030,#722,.T.);
#10466=EDGE_CURVE('',#8032,#8031,#723,.T.);
#10467=EDGE_CURVE('',#8032,#8033,#6441,.T.);
#10468=EDGE_CURVE('',#8034,#8033,#724,.T.);
#10469=EDGE_CURVE('',#8035,#8034,#725,.T.);
#10470=EDGE_CURVE('',#8035,#8036,#6442,.T.);
#10471=EDGE_CURVE('',#8037,#8036,#726,.T.);
#10472=EDGE_CURVE('',#8038,#8037,#727,.T.);
#10473=EDGE_CURVE('',#8038,#8039,#6443,.T.);
#10474=EDGE_CURVE('',#8040,#8039,#728,.T.);
#10475=EDGE_CURVE('',#8041,#8040,#729,.T.);
#10476=EDGE_CURVE('',#8041,#8042,#6444,.T.);
#10477=EDGE_CURVE('',#8043,#8042,#730,.T.);
#10478=EDGE_CURVE('',#8044,#8043,#731,.T.);
#10479=EDGE_CURVE('',#8044,#8045,#6445,.T.);
#10480=EDGE_CURVE('',#8046,#8045,#732,.T.);
#10481=EDGE_CURVE('',#8047,#8046,#733,.T.);
#10482=EDGE_CURVE('',#8047,#8048,#6446,.T.);
#10483=EDGE_CURVE('',#8049,#8048,#734,.T.);
#10484=EDGE_CURVE('',#8050,#8049,#735,.T.);
#10485=EDGE_CURVE('',#8050,#8051,#6447,.T.);
#10486=EDGE_CURVE('',#8052,#8051,#736,.T.);
#10487=EDGE_CURVE('',#8053,#8052,#737,.T.);
#10488=EDGE_CURVE('',#8053,#8054,#6448,.T.);
#10489=EDGE_CURVE('',#8055,#8054,#738,.T.);
#10490=EDGE_CURVE('',#8056,#8055,#739,.T.);
#10491=EDGE_CURVE('',#8056,#8057,#6449,.T.);
#10492=EDGE_CURVE('',#8058,#8057,#740,.T.);
#10493=EDGE_CURVE('',#8059,#8058,#741,.T.);
#10494=EDGE_CURVE('',#8059,#8060,#6450,.T.);
#10495=EDGE_CURVE('',#8061,#8060,#742,.T.);
#10496=EDGE_CURVE('',#8062,#8061,#743,.T.);
#10497=EDGE_CURVE('',#8062,#8063,#6451,.T.);
#10498=EDGE_CURVE('',#8064,#8063,#744,.T.);
#10499=EDGE_CURVE('',#8065,#8064,#745,.T.);
#10500=EDGE_CURVE('',#8065,#8066,#6452,.T.);
#10501=EDGE_CURVE('',#8067,#8066,#746,.T.);
#10502=EDGE_CURVE('',#8068,#8067,#747,.T.);
#10503=EDGE_CURVE('',#8068,#8069,#6453,.T.);
#10504=EDGE_CURVE('',#8070,#8069,#748,.T.);
#10505=EDGE_CURVE('',#8071,#8070,#749,.T.);
#10506=EDGE_CURVE('',#8071,#8072,#6454,.T.);
#10507=EDGE_CURVE('',#8073,#8072,#750,.T.);
#10508=EDGE_CURVE('',#8074,#8073,#751,.T.);
#10509=EDGE_CURVE('',#8074,#8075,#6455,.T.);
#10510=EDGE_CURVE('',#8076,#8075,#752,.T.);
#10511=EDGE_CURVE('',#8077,#8076,#753,.T.);
#10512=EDGE_CURVE('',#8077,#8078,#6456,.T.);
#10513=EDGE_CURVE('',#8079,#8078,#754,.T.);
#10514=EDGE_CURVE('',#8080,#8079,#755,.T.);
#10515=EDGE_CURVE('',#8080,#8081,#6457,.T.);
#10516=EDGE_CURVE('',#8082,#8081,#756,.T.);
#10517=EDGE_CURVE('',#8083,#8082,#757,.T.);
#10518=EDGE_CURVE('',#8083,#8084,#6458,.T.);
#10519=EDGE_CURVE('',#8085,#8084,#758,.T.);
#10520=EDGE_CURVE('',#8086,#8085,#759,.T.);
#10521=EDGE_CURVE('',#8086,#8087,#6459,.T.);
#10522=EDGE_CURVE('',#8088,#8087,#760,.T.);
#10523=EDGE_CURVE('',#8089,#8088,#761,.T.);
#10524=EDGE_CURVE('',#8089,#8090,#6460,.T.);
#10525=EDGE_CURVE('',#8091,#8090,#762,.T.);
#10526=EDGE_CURVE('',#8092,#8091,#763,.T.);
#10527=EDGE_CURVE('',#8092,#8093,#6461,.T.);
#10528=EDGE_CURVE('',#8094,#8093,#764,.T.);
#10529=EDGE_CURVE('',#8095,#8094,#765,.T.);
#10530=EDGE_CURVE('',#8095,#8096,#6462,.T.);
#10531=EDGE_CURVE('',#8097,#8096,#766,.T.);
#10532=EDGE_CURVE('',#8098,#8097,#767,.T.);
#10533=EDGE_CURVE('',#8098,#8099,#6463,.T.);
#10534=EDGE_CURVE('',#8100,#8099,#768,.T.);
#10535=EDGE_CURVE('',#8101,#8100,#769,.T.);
#10536=EDGE_CURVE('',#8101,#8102,#6464,.T.);
#10537=EDGE_CURVE('',#8103,#8102,#770,.T.);
#10538=EDGE_CURVE('',#8104,#8103,#771,.T.);
#10539=EDGE_CURVE('',#8104,#8105,#6465,.T.);
#10540=EDGE_CURVE('',#8106,#8105,#772,.T.);
#10541=EDGE_CURVE('',#8107,#8106,#773,.T.);
#10542=EDGE_CURVE('',#8107,#8108,#6466,.T.);
#10543=EDGE_CURVE('',#8109,#8108,#774,.T.);
#10544=EDGE_CURVE('',#8110,#8109,#775,.T.);
#10545=EDGE_CURVE('',#8110,#8111,#6467,.T.);
#10546=EDGE_CURVE('',#8112,#8111,#776,.T.);
#10547=EDGE_CURVE('',#8113,#8112,#777,.T.);
#10548=EDGE_CURVE('',#8113,#8114,#6468,.T.);
#10549=EDGE_CURVE('',#8115,#8114,#778,.T.);
#10550=EDGE_CURVE('',#8116,#8115,#779,.T.);
#10551=EDGE_CURVE('',#8116,#8117,#6469,.T.);
#10552=EDGE_CURVE('',#8118,#8117,#780,.T.);
#10553=EDGE_CURVE('',#8119,#8118,#781,.T.);
#10554=EDGE_CURVE('',#8119,#8120,#6470,.T.);
#10555=EDGE_CURVE('',#8121,#8120,#782,.T.);
#10556=EDGE_CURVE('',#8122,#8121,#783,.T.);
#10557=EDGE_CURVE('',#8122,#8123,#6471,.T.);
#10558=EDGE_CURVE('',#8124,#8123,#784,.F.);
#10559=EDGE_CURVE('',#8124,#8125,#4409,.T.);
#10560=EDGE_CURVE('',#8125,#8125,#6472,.T.);
#10561=EDGE_CURVE('',#8126,#8124,#785,.F.);
#10562=EDGE_CURVE('',#8127,#8126,#786,.T.);
#10563=EDGE_CURVE('',#8127,#8128,#6473,.T.);
#10564=EDGE_CURVE('',#8129,#8128,#787,.T.);
#10565=EDGE_CURVE('',#8130,#8129,#788,.T.);
#10566=EDGE_CURVE('',#8130,#8131,#6474,.T.);
#10567=EDGE_CURVE('',#8132,#8131,#789,.T.);
#10568=EDGE_CURVE('',#8133,#8132,#790,.T.);
#10569=EDGE_CURVE('',#8133,#8134,#6475,.T.);
#10570=EDGE_CURVE('',#8135,#8134,#791,.T.);
#10571=EDGE_CURVE('',#8136,#8135,#792,.T.);
#10572=EDGE_CURVE('',#8136,#8137,#6476,.T.);
#10573=EDGE_CURVE('',#8138,#8137,#793,.T.);
#10574=EDGE_CURVE('',#8139,#8138,#794,.T.);
#10575=EDGE_CURVE('',#8139,#8140,#6477,.T.);
#10576=EDGE_CURVE('',#8141,#8140,#795,.T.);
#10577=EDGE_CURVE('',#8142,#8141,#796,.T.);
#10578=EDGE_CURVE('',#8142,#8143,#6478,.T.);
#10579=EDGE_CURVE('',#8144,#8143,#797,.T.);
#10580=EDGE_CURVE('',#8145,#8144,#798,.T.);
#10581=EDGE_CURVE('',#8145,#8146,#6479,.T.);
#10582=EDGE_CURVE('',#8147,#8146,#799,.T.);
#10583=EDGE_CURVE('',#8148,#8147,#800,.T.);
#10584=EDGE_CURVE('',#8148,#8149,#6480,.T.);
#10585=EDGE_CURVE('',#8150,#8149,#801,.T.);
#10586=EDGE_CURVE('',#8151,#8150,#802,.T.);
#10587=EDGE_CURVE('',#8151,#8152,#6481,.T.);
#10588=EDGE_CURVE('',#8153,#8152,#803,.T.);
#10589=EDGE_CURVE('',#8154,#8153,#804,.T.);
#10590=EDGE_CURVE('',#8154,#8155,#6482,.T.);
#10591=EDGE_CURVE('',#8156,#8155,#805,.T.);
#10592=EDGE_CURVE('',#8157,#8156,#806,.T.);
#10593=EDGE_CURVE('',#8157,#8158,#6483,.T.);
#10594=EDGE_CURVE('',#8159,#8158,#807,.T.);
#10595=EDGE_CURVE('',#8160,#8159,#808,.T.);
#10596=EDGE_CURVE('',#8160,#8161,#6484,.T.);
#10597=EDGE_CURVE('',#8162,#8161,#809,.T.);
#10598=EDGE_CURVE('',#8163,#8162,#810,.T.);
#10599=EDGE_CURVE('',#8163,#8164,#6485,.T.);
#10600=EDGE_CURVE('',#8165,#8164,#811,.T.);
#10601=EDGE_CURVE('',#8166,#8165,#812,.T.);
#10602=EDGE_CURVE('',#8166,#8167,#6486,.T.);
#10603=EDGE_CURVE('',#8168,#8167,#813,.T.);
#10604=EDGE_CURVE('',#8169,#8168,#814,.T.);
#10605=EDGE_CURVE('',#8169,#8170,#6487,.T.);
#10606=EDGE_CURVE('',#8171,#8170,#815,.T.);
#10607=EDGE_CURVE('',#8172,#8171,#816,.T.);
#10608=EDGE_CURVE('',#8172,#8173,#6488,.T.);
#10609=EDGE_CURVE('',#8174,#8173,#817,.T.);
#10610=EDGE_CURVE('',#8175,#8174,#818,.T.);
#10611=EDGE_CURVE('',#8175,#8176,#6489,.T.);
#10612=EDGE_CURVE('',#8177,#8176,#819,.T.);
#10613=EDGE_CURVE('',#8178,#8177,#820,.T.);
#10614=EDGE_CURVE('',#8178,#8179,#6490,.T.);
#10615=EDGE_CURVE('',#8180,#8179,#821,.T.);
#10616=EDGE_CURVE('',#8181,#8180,#822,.T.);
#10617=EDGE_CURVE('',#8181,#8182,#6491,.T.);
#10618=EDGE_CURVE('',#8183,#8182,#823,.T.);
#10619=EDGE_CURVE('',#8184,#8183,#824,.T.);
#10620=EDGE_CURVE('',#8184,#8185,#6492,.T.);
#10621=EDGE_CURVE('',#8186,#8185,#825,.T.);
#10622=EDGE_CURVE('',#8187,#8186,#826,.T.);
#10623=EDGE_CURVE('',#8187,#8188,#6493,.T.);
#10624=EDGE_CURVE('',#8189,#8188,#827,.T.);
#10625=EDGE_CURVE('',#8190,#8189,#828,.T.);
#10626=EDGE_CURVE('',#8190,#8191,#6494,.T.);
#10627=EDGE_CURVE('',#8192,#8191,#829,.T.);
#10628=EDGE_CURVE('',#8193,#8192,#830,.T.);
#10629=EDGE_CURVE('',#8193,#8194,#6495,.T.);
#10630=EDGE_CURVE('',#8195,#8194,#831,.T.);
#10631=EDGE_CURVE('',#8196,#8195,#832,.T.);
#10632=EDGE_CURVE('',#8196,#8197,#6496,.T.);
#10633=EDGE_CURVE('',#8198,#8197,#833,.T.);
#10634=EDGE_CURVE('',#8199,#8198,#834,.T.);
#10635=EDGE_CURVE('',#8199,#8200,#6497,.T.);
#10636=EDGE_CURVE('',#8201,#8200,#835,.T.);
#10637=EDGE_CURVE('',#8202,#8201,#836,.T.);
#10638=EDGE_CURVE('',#8202,#8203,#6498,.T.);
#10639=EDGE_CURVE('',#8204,#8203,#837,.T.);
#10640=EDGE_CURVE('',#8205,#8204,#838,.T.);
#10641=EDGE_CURVE('',#8205,#8206,#6499,.T.);
#10642=EDGE_CURVE('',#8207,#8206,#839,.T.);
#10643=EDGE_CURVE('',#8208,#8207,#840,.T.);
#10644=EDGE_CURVE('',#8208,#8209,#6500,.T.);
#10645=EDGE_CURVE('',#8210,#8209,#841,.T.);
#10646=EDGE_CURVE('',#8211,#8210,#842,.T.);
#10647=EDGE_CURVE('',#8211,#8212,#6501,.T.);
#10648=EDGE_CURVE('',#8213,#8212,#843,.T.);
#10649=EDGE_CURVE('',#8214,#8213,#844,.T.);
#10650=EDGE_CURVE('',#8214,#8215,#6502,.T.);
#10651=EDGE_CURVE('',#8216,#8215,#845,.T.);
#10652=EDGE_CURVE('',#8217,#8216,#846,.T.);
#10653=EDGE_CURVE('',#8217,#8218,#6503,.T.);
#10654=EDGE_CURVE('',#8219,#8218,#847,.T.);
#10655=EDGE_CURVE('',#8220,#8219,#848,.T.);
#10656=EDGE_CURVE('',#8220,#8221,#6504,.T.);
#10657=EDGE_CURVE('',#8222,#8221,#849,.T.);
#10658=EDGE_CURVE('',#8223,#8222,#850,.T.);
#10659=EDGE_CURVE('',#8223,#8224,#6505,.T.);
#10660=EDGE_CURVE('',#8225,#8224,#851,.T.);
#10661=EDGE_CURVE('',#8226,#8225,#852,.T.);
#10662=EDGE_CURVE('',#8226,#8227,#6506,.T.);
#10663=EDGE_CURVE('',#8228,#8227,#853,.T.);
#10664=EDGE_CURVE('',#8229,#8228,#854,.T.);
#10665=EDGE_CURVE('',#8229,#8230,#6507,.T.);
#10666=EDGE_CURVE('',#8231,#8230,#855,.T.);
#10667=EDGE_CURVE('',#8232,#8231,#856,.T.);
#10668=EDGE_CURVE('',#8232,#8233,#6508,.T.);
#10669=EDGE_CURVE('',#8234,#8233,#857,.T.);
#10670=EDGE_CURVE('',#8235,#8234,#858,.T.);
#10671=EDGE_CURVE('',#8235,#8236,#6509,.T.);
#10672=EDGE_CURVE('',#8237,#8236,#859,.T.);
#10673=EDGE_CURVE('',#8238,#8237,#860,.T.);
#10674=EDGE_CURVE('',#8238,#8239,#6510,.T.);
#10675=EDGE_CURVE('',#8008,#8239,#861,.T.);
#10676=EDGE_CURVE('',#8240,#8240,#6511,.T.);
#10677=EDGE_CURVE('',#8240,#7769,#4410,.T.);
#10678=EDGE_CURVE('',#7955,#8178,#4411,.T.);
#10679=EDGE_CURVE('',#7954,#8179,#4412,.T.);
#10680=EDGE_CURVE('',#7957,#8176,#4413,.T.);
#10681=EDGE_CURVE('',#7958,#8175,#4414,.T.);
#10682=EDGE_CURVE('',#7960,#8173,#4415,.T.);
#10683=EDGE_CURVE('',#7961,#8172,#4416,.T.);
#10684=EDGE_CURVE('',#7963,#8170,#4417,.T.);
#10685=EDGE_CURVE('',#7964,#8169,#4418,.T.);
#10686=EDGE_CURVE('',#7966,#8167,#4419,.T.);
#10687=EDGE_CURVE('',#7967,#8166,#4420,.T.);
#10688=EDGE_CURVE('',#7969,#8164,#4421,.T.);
#10689=EDGE_CURVE('',#7970,#8163,#4422,.T.);
#10690=EDGE_CURVE('',#7972,#8161,#4423,.T.);
#10691=EDGE_CURVE('',#7973,#8160,#4424,.T.);
#10692=EDGE_CURVE('',#7975,#8158,#4425,.T.);
#10693=EDGE_CURVE('',#7976,#8157,#4426,.T.);
#10694=EDGE_CURVE('',#7978,#8155,#4427,.T.);
#10695=EDGE_CURVE('',#7979,#8154,#4428,.T.);
#10696=EDGE_CURVE('',#7981,#8152,#4429,.T.);
#10697=EDGE_CURVE('',#7982,#8151,#4430,.T.);
#10698=EDGE_CURVE('',#7984,#8149,#4431,.T.);
#10699=EDGE_CURVE('',#7985,#8148,#4432,.T.);
#10700=EDGE_CURVE('',#7987,#8146,#4433,.T.);
#10701=EDGE_CURVE('',#7988,#8145,#4434,.T.);
#10702=EDGE_CURVE('',#7990,#8143,#4435,.T.);
#10703=EDGE_CURVE('',#7991,#8142,#4436,.T.);
#10704=EDGE_CURVE('',#7993,#8140,#4437,.T.);
#10705=EDGE_CURVE('',#7994,#8139,#4438,.T.);
#10706=EDGE_CURVE('',#7996,#8137,#4439,.T.);
#10707=EDGE_CURVE('',#7997,#8136,#4440,.T.);
#10708=EDGE_CURVE('',#7999,#8134,#4441,.T.);
#10709=EDGE_CURVE('',#8000,#8133,#4442,.T.);
#10710=EDGE_CURVE('',#8002,#8131,#4443,.T.);
#10711=EDGE_CURVE('',#8003,#8130,#4444,.T.);
#10712=EDGE_CURVE('',#8005,#8128,#4445,.T.);
#10713=EDGE_CURVE('',#8006,#8127,#4446,.T.);
#10714=EDGE_CURVE('',#7775,#8123,#4447,.T.);
#10715=EDGE_CURVE('',#7776,#8122,#4448,.T.);
#10716=EDGE_CURVE('',#7778,#8120,#4449,.T.);
#10717=EDGE_CURVE('',#7779,#8119,#4450,.T.);
#10718=EDGE_CURVE('',#7781,#8117,#4451,.T.);
#10719=EDGE_CURVE('',#7782,#8116,#4452,.T.);
#10720=EDGE_CURVE('',#7784,#8114,#4453,.T.);
#10721=EDGE_CURVE('',#7785,#8113,#4454,.T.);
#10722=EDGE_CURVE('',#7787,#8111,#4455,.T.);
#10723=EDGE_CURVE('',#7788,#8110,#4456,.T.);
#10724=EDGE_CURVE('',#7790,#8108,#4457,.T.);
#10725=EDGE_CURVE('',#7791,#8107,#4458,.T.);
#10726=EDGE_CURVE('',#7793,#8105,#4459,.T.);
#10727=EDGE_CURVE('',#7794,#8104,#4460,.T.);
#10728=EDGE_CURVE('',#7796,#8102,#4461,.T.);
#10729=EDGE_CURVE('',#7797,#8101,#4462,.T.);
#10730=EDGE_CURVE('',#7799,#8099,#4463,.T.);
#10731=EDGE_CURVE('',#7800,#8098,#4464,.T.);
#10732=EDGE_CURVE('',#7802,#8096,#4465,.T.);
#10733=EDGE_CURVE('',#7803,#8095,#4466,.T.);
#10734=EDGE_CURVE('',#7805,#8093,#4467,.T.);
#10735=EDGE_CURVE('',#7806,#8092,#4468,.T.);
#10736=EDGE_CURVE('',#7808,#8090,#4469,.T.);
#10737=EDGE_CURVE('',#7809,#8089,#4470,.T.);
#10738=EDGE_CURVE('',#7811,#8087,#4471,.T.);
#10739=EDGE_CURVE('',#7812,#8086,#4472,.T.);
#10740=EDGE_CURVE('',#7814,#8084,#4473,.T.);
#10741=EDGE_CURVE('',#7815,#8083,#4474,.T.);
#10742=EDGE_CURVE('',#7817,#8081,#4475,.T.);
#10743=EDGE_CURVE('',#7818,#8080,#4476,.T.);
#10744=EDGE_CURVE('',#7820,#8078,#4477,.T.);
#10745=EDGE_CURVE('',#7821,#8077,#4478,.T.);
#10746=EDGE_CURVE('',#7823,#8075,#4479,.T.);
#10747=EDGE_CURVE('',#7824,#8074,#4480,.T.);
#10748=EDGE_CURVE('',#7826,#8072,#4481,.T.);
#10749=EDGE_CURVE('',#7827,#8071,#4482,.T.);
#10750=EDGE_CURVE('',#7829,#8069,#4483,.T.);
#10751=EDGE_CURVE('',#7830,#8068,#4484,.T.);
#10752=EDGE_CURVE('',#7832,#8066,#4485,.T.);
#10753=EDGE_CURVE('',#7833,#8065,#4486,.T.);
#10754=EDGE_CURVE('',#7835,#8063,#4487,.T.);
#10755=EDGE_CURVE('',#7836,#8062,#4488,.T.);
#10756=EDGE_CURVE('',#7838,#8060,#4489,.T.);
#10757=EDGE_CURVE('',#7839,#8059,#4490,.T.);
#10758=EDGE_CURVE('',#7841,#8057,#4491,.T.);
#10759=EDGE_CURVE('',#7842,#8056,#4492,.T.);
#10760=EDGE_CURVE('',#7844,#8054,#4493,.T.);
#10761=EDGE_CURVE('',#7845,#8053,#4494,.T.);
#10762=EDGE_CURVE('',#7847,#8051,#4495,.T.);
#10763=EDGE_CURVE('',#7848,#8050,#4496,.T.);
#10764=EDGE_CURVE('',#7850,#8048,#4497,.T.);
#10765=EDGE_CURVE('',#7851,#8047,#4498,.T.);
#10766=EDGE_CURVE('',#7853,#8045,#4499,.T.);
#10767=EDGE_CURVE('',#7854,#8044,#4500,.T.);
#10768=EDGE_CURVE('',#7856,#8042,#4501,.T.);
#10769=EDGE_CURVE('',#7857,#8041,#4502,.T.);
#10770=EDGE_CURVE('',#7859,#8039,#4503,.T.);
#10771=EDGE_CURVE('',#7860,#8038,#4504,.T.);
#10772=EDGE_CURVE('',#7862,#8036,#4505,.T.);
#10773=EDGE_CURVE('',#7863,#8035,#4506,.T.);
#10774=EDGE_CURVE('',#7865,#8033,#4507,.T.);
#10775=EDGE_CURVE('',#7866,#8032,#4508,.T.);
#10776=EDGE_CURVE('',#7868,#8030,#4509,.T.);
#10777=EDGE_CURVE('',#7869,#8029,#4510,.T.);
#10778=EDGE_CURVE('',#7871,#8027,#4511,.T.);
#10779=EDGE_CURVE('',#7872,#8026,#4512,.T.);
#10780=EDGE_CURVE('',#7874,#8024,#4513,.T.);
#10781=EDGE_CURVE('',#7875,#8023,#4514,.T.);
#10782=EDGE_CURVE('',#7877,#8021,#4515,.T.);
#10783=EDGE_CURVE('',#7878,#8020,#4516,.T.);
#10784=EDGE_CURVE('',#7880,#8018,#4517,.T.);
#10785=EDGE_CURVE('',#7881,#8017,#4518,.T.);
#10786=EDGE_CURVE('',#7883,#8015,#4519,.T.);
#10787=EDGE_CURVE('',#7884,#8014,#4520,.T.);
#10788=EDGE_CURVE('',#7886,#8012,#4521,.T.);
#10789=EDGE_CURVE('',#7887,#8011,#4522,.T.);
#10790=EDGE_CURVE('',#7889,#8009,#4523,.T.);
#10791=EDGE_CURVE('',#7890,#8007,#4524,.T.);
#10792=EDGE_CURVE('',#7894,#8239,#4525,.T.);
#10793=EDGE_CURVE('',#7895,#8238,#4526,.T.);
#10794=EDGE_CURVE('',#7897,#8236,#4527,.T.);
#10795=EDGE_CURVE('',#7898,#8235,#4528,.T.);
#10796=EDGE_CURVE('',#7900,#8233,#4529,.T.);
#10797=EDGE_CURVE('',#7901,#8232,#4530,.T.);
#10798=EDGE_CURVE('',#7903,#8230,#4531,.T.);
#10799=EDGE_CURVE('',#7904,#8229,#4532,.T.);
#10800=EDGE_CURVE('',#7906,#8227,#4533,.T.);
#10801=EDGE_CURVE('',#7907,#8226,#4534,.T.);
#10802=EDGE_CURVE('',#7909,#8224,#4535,.T.);
#10803=EDGE_CURVE('',#7910,#8223,#4536,.T.);
#10804=EDGE_CURVE('',#7912,#8221,#4537,.T.);
#10805=EDGE_CURVE('',#7913,#8220,#4538,.T.);
#10806=EDGE_CURVE('',#7915,#8218,#4539,.T.);
#10807=EDGE_CURVE('',#7916,#8217,#4540,.T.);
#10808=EDGE_CURVE('',#7918,#8215,#4541,.T.);
#10809=EDGE_CURVE('',#7919,#8214,#4542,.T.);
#10810=EDGE_CURVE('',#7921,#8212,#4543,.T.);
#10811=EDGE_CURVE('',#7922,#8211,#4544,.T.);
#10812=EDGE_CURVE('',#7924,#8209,#4545,.T.);
#10813=EDGE_CURVE('',#7925,#8208,#4546,.T.);
#10814=EDGE_CURVE('',#7927,#8206,#4547,.T.);
#10815=EDGE_CURVE('',#7928,#8205,#4548,.T.);
#10816=EDGE_CURVE('',#7930,#8203,#4549,.T.);
#10817=EDGE_CURVE('',#7931,#8202,#4550,.T.);
#10818=EDGE_CURVE('',#7933,#8200,#4551,.T.);
#10819=EDGE_CURVE('',#7934,#8199,#4552,.T.);
#10820=EDGE_CURVE('',#7936,#8197,#4553,.T.);
#10821=EDGE_CURVE('',#7937,#8196,#4554,.T.);
#10822=EDGE_CURVE('',#7939,#8194,#4555,.T.);
#10823=EDGE_CURVE('',#7940,#8193,#4556,.T.);
#10824=EDGE_CURVE('',#7942,#8191,#4557,.T.);
#10825=EDGE_CURVE('',#7943,#8190,#4558,.T.);
#10826=EDGE_CURVE('',#7945,#8188,#4559,.T.);
#10827=EDGE_CURVE('',#7946,#8187,#4560,.T.);
#10828=EDGE_CURVE('',#7952,#8181,#4561,.T.);
#10829=EDGE_CURVE('',#7951,#8182,#4562,.T.);
#10830=EDGE_CURVE('',#7948,#8185,#4563,.T.);
#10831=EDGE_CURVE('',#7949,#8184,#4564,.T.);
#10832=EDGE_CURVE('',#7950,#8183,#4565,.T.);
#10833=EDGE_CURVE('',#7953,#8180,#4566,.T.);
#10834=EDGE_CURVE('',#7947,#8186,#4567,.T.);
#10835=EDGE_CURVE('',#7944,#8189,#4568,.T.);
#10836=EDGE_CURVE('',#7941,#8192,#4569,.T.);
#10837=EDGE_CURVE('',#7938,#8195,#4570,.T.);
#10838=EDGE_CURVE('',#7935,#8198,#4571,.T.);
#10839=EDGE_CURVE('',#7932,#8201,#4572,.T.);
#10840=EDGE_CURVE('',#7929,#8204,#4573,.T.);
#10841=EDGE_CURVE('',#7926,#8207,#4574,.T.);
#10842=EDGE_CURVE('',#7923,#8210,#4575,.T.);
#10843=EDGE_CURVE('',#7920,#8213,#4576,.T.);
#10844=EDGE_CURVE('',#7917,#8216,#4577,.T.);
#10845=EDGE_CURVE('',#7914,#8219,#4578,.T.);
#10846=EDGE_CURVE('',#7911,#8222,#4579,.T.);
#10847=EDGE_CURVE('',#7908,#8225,#4580,.T.);
#10848=EDGE_CURVE('',#7905,#8228,#4581,.T.);
#10849=EDGE_CURVE('',#7902,#8231,#4582,.T.);
#10850=EDGE_CURVE('',#7899,#8234,#4583,.T.);
#10851=EDGE_CURVE('',#7896,#8237,#4584,.T.);
#10852=EDGE_CURVE('',#7893,#8008,#4585,.T.);
#10853=EDGE_CURVE('',#7888,#8010,#4586,.T.);
#10854=EDGE_CURVE('',#7885,#8013,#4587,.T.);
#10855=EDGE_CURVE('',#7882,#8016,#4588,.T.);
#10856=EDGE_CURVE('',#7879,#8019,#4589,.T.);
#10857=EDGE_CURVE('',#7876,#8022,#4590,.T.);
#10858=EDGE_CURVE('',#7873,#8025,#4591,.T.);
#10859=EDGE_CURVE('',#7870,#8028,#4592,.T.);
#10860=EDGE_CURVE('',#7867,#8031,#4593,.T.);
#10861=EDGE_CURVE('',#7864,#8034,#4594,.T.);
#10862=EDGE_CURVE('',#7861,#8037,#4595,.T.);
#10863=EDGE_CURVE('',#7858,#8040,#4596,.T.);
#10864=EDGE_CURVE('',#7855,#8043,#4597,.T.);
#10865=EDGE_CURVE('',#7852,#8046,#4598,.T.);
#10866=EDGE_CURVE('',#7849,#8049,#4599,.T.);
#10867=EDGE_CURVE('',#7846,#8052,#4600,.T.);
#10868=EDGE_CURVE('',#7843,#8055,#4601,.T.);
#10869=EDGE_CURVE('',#7840,#8058,#4602,.T.);
#10870=EDGE_CURVE('',#7837,#8061,#4603,.T.);
#10871=EDGE_CURVE('',#7834,#8064,#4604,.T.);
#10872=EDGE_CURVE('',#7831,#8067,#4605,.T.);
#10873=EDGE_CURVE('',#7828,#8070,#4606,.T.);
#10874=EDGE_CURVE('',#7825,#8073,#4607,.T.);
#10875=EDGE_CURVE('',#7822,#8076,#4608,.T.);
#10876=EDGE_CURVE('',#7819,#8079,#4609,.T.);
#10877=EDGE_CURVE('',#7816,#8082,#4610,.T.);
#10878=EDGE_CURVE('',#7813,#8085,#4611,.T.);
#10879=EDGE_CURVE('',#7810,#8088,#4612,.T.);
#10880=EDGE_CURVE('',#7807,#8091,#4613,.T.);
#10881=EDGE_CURVE('',#7804,#8094,#4614,.T.);
#10882=EDGE_CURVE('',#7801,#8097,#4615,.T.);
#10883=EDGE_CURVE('',#7798,#8100,#4616,.T.);
#10884=EDGE_CURVE('',#7795,#8103,#4617,.T.);
#10885=EDGE_CURVE('',#7792,#8106,#4618,.T.);
#10886=EDGE_CURVE('',#7789,#8109,#4619,.T.);
#10887=EDGE_CURVE('',#7786,#8112,#4620,.T.);
#10888=EDGE_CURVE('',#7783,#8115,#4621,.T.);
#10889=EDGE_CURVE('',#7780,#8118,#4622,.T.);
#10890=EDGE_CURVE('',#7777,#8121,#4623,.T.);
#10891=EDGE_CURVE('',#7774,#8126,#4624,.T.);
#10892=EDGE_CURVE('',#8004,#8129,#4625,.T.);
#10893=EDGE_CURVE('',#8001,#8132,#4626,.T.);
#10894=EDGE_CURVE('',#7998,#8135,#4627,.T.);
#10895=EDGE_CURVE('',#7995,#8138,#4628,.T.);
#10896=EDGE_CURVE('',#7992,#8141,#4629,.T.);
#10897=EDGE_CURVE('',#7989,#8144,#4630,.T.);
#10898=EDGE_CURVE('',#7986,#8147,#4631,.T.);
#10899=EDGE_CURVE('',#7983,#8150,#4632,.T.);
#10900=EDGE_CURVE('',#7980,#8153,#4633,.T.);
#10901=EDGE_CURVE('',#7977,#8156,#4634,.T.);
#10902=EDGE_CURVE('',#7974,#8159,#4635,.T.);
#10903=EDGE_CURVE('',#7971,#8162,#4636,.T.);
#10904=EDGE_CURVE('',#7968,#8165,#4637,.T.);
#10905=EDGE_CURVE('',#7965,#8168,#4638,.T.);
#10906=EDGE_CURVE('',#7962,#8171,#4639,.T.);
#10907=EDGE_CURVE('',#7959,#8174,#4640,.T.);
#10908=EDGE_CURVE('',#7956,#8177,#4641,.T.);
#12369=ORIENTED_EDGE('',*,*,#8971,.F.);
#12370=ORIENTED_EDGE('',*,*,#8972,.T.);
#12371=ORIENTED_EDGE('',*,*,#8973,.F.);
#12372=ORIENTED_EDGE('',*,*,#8972,.F.);
#12373=ORIENTED_EDGE('',*,*,#8974,.F.);
#12374=ORIENTED_EDGE('',*,*,#8975,.F.);
#12375=ORIENTED_EDGE('',*,*,#8976,.T.);
#12376=ORIENTED_EDGE('',*,*,#8977,.F.);
#12377=ORIENTED_EDGE('',*,*,#8976,.F.);
#12378=ORIENTED_EDGE('',*,*,#8978,.F.);
#12379=ORIENTED_EDGE('',*,*,#8979,.F.);
#12380=ORIENTED_EDGE('',*,*,#8980,.T.);
#12381=ORIENTED_EDGE('',*,*,#8981,.F.);
#12382=ORIENTED_EDGE('',*,*,#8980,.F.);
#12383=ORIENTED_EDGE('',*,*,#8982,.F.);
#12384=ORIENTED_EDGE('',*,*,#8983,.T.);
#12385=ORIENTED_EDGE('',*,*,#8984,.F.);
#12386=ORIENTED_EDGE('',*,*,#8983,.F.);
#12387=ORIENTED_EDGE('',*,*,#8985,.F.);
#12388=ORIENTED_EDGE('',*,*,#8986,.F.);
#12389=ORIENTED_EDGE('',*,*,#8987,.F.);
#12390=ORIENTED_EDGE('',*,*,#8988,.F.);
#12391=ORIENTED_EDGE('',*,*,#8989,.F.);
#12392=ORIENTED_EDGE('',*,*,#8990,.F.);
#12393=ORIENTED_EDGE('',*,*,#8991,.T.);
#12394=ORIENTED_EDGE('',*,*,#8992,.F.);
#12395=ORIENTED_EDGE('',*,*,#8991,.F.);
#12396=ORIENTED_EDGE('',*,*,#8993,.F.);
#12397=ORIENTED_EDGE('',*,*,#8994,.F.);
#12398=ORIENTED_EDGE('',*,*,#8995,.T.);
#12399=ORIENTED_EDGE('',*,*,#8996,.F.);
#12400=ORIENTED_EDGE('',*,*,#8995,.F.);
#12401=ORIENTED_EDGE('',*,*,#8997,.F.);
#12402=ORIENTED_EDGE('',*,*,#8998,.T.);
#12403=ORIENTED_EDGE('',*,*,#8999,.F.);
#12404=ORIENTED_EDGE('',*,*,#8998,.F.);
#12405=ORIENTED_EDGE('',*,*,#9000,.F.);
#12406=ORIENTED_EDGE('',*,*,#9001,.T.);
#12407=ORIENTED_EDGE('',*,*,#9002,.F.);
#12408=ORIENTED_EDGE('',*,*,#9001,.F.);
#12409=ORIENTED_EDGE('',*,*,#9003,.F.);
#12410=ORIENTED_EDGE('',*,*,#9004,.F.);
#12411=ORIENTED_EDGE('',*,*,#9005,.F.);
#12412=ORIENTED_EDGE('',*,*,#9006,.F.);
#12413=ORIENTED_EDGE('',*,*,#8993,.T.);
#12414=ORIENTED_EDGE('',*,*,#8994,.T.);
#12415=ORIENTED_EDGE('',*,*,#9007,.T.);
#12416=ORIENTED_EDGE('',*,*,#9008,.F.);
#12417=ORIENTED_EDGE('',*,*,#9009,.F.);
#12418=ORIENTED_EDGE('',*,*,#9010,.F.);
#12419=ORIENTED_EDGE('',*,*,#9007,.F.);
#12420=ORIENTED_EDGE('',*,*,#9011,.F.);
#12421=ORIENTED_EDGE('',*,*,#9012,.T.);
#12422=ORIENTED_EDGE('',*,*,#8971,.T.);
#12423=ORIENTED_EDGE('',*,*,#9012,.F.);
#12424=ORIENTED_EDGE('',*,*,#8989,.T.);
#12425=ORIENTED_EDGE('',*,*,#8990,.T.);
#12426=ORIENTED_EDGE('',*,*,#9013,.T.);
#12427=ORIENTED_EDGE('',*,*,#8982,.T.);
#12428=ORIENTED_EDGE('',*,*,#9013,.F.);
#12429=ORIENTED_EDGE('',*,*,#8985,.T.);
#12430=ORIENTED_EDGE('',*,*,#9014,.T.);
#12431=ORIENTED_EDGE('',*,*,#9003,.T.);
#12432=ORIENTED_EDGE('',*,*,#9015,.F.);
#12433=ORIENTED_EDGE('',*,*,#9009,.T.);
#12434=ORIENTED_EDGE('',*,*,#9016,.F.);
#12435=ORIENTED_EDGE('',*,*,#8978,.T.);
#12436=ORIENTED_EDGE('',*,*,#8979,.T.);
#12437=ORIENTED_EDGE('',*,*,#9017,.T.);
#12438=ORIENTED_EDGE('',*,*,#8997,.T.);
#12439=ORIENTED_EDGE('',*,*,#9017,.F.);
#12440=ORIENTED_EDGE('',*,*,#8974,.T.);
#12441=ORIENTED_EDGE('',*,*,#8975,.T.);
#12442=ORIENTED_EDGE('',*,*,#9018,.T.);
#12443=ORIENTED_EDGE('',*,*,#9000,.T.);
#12444=ORIENTED_EDGE('',*,*,#9018,.F.);
#12445=ORIENTED_EDGE('',*,*,#9019,.F.);
#12446=ORIENTED_EDGE('',*,*,#9020,.T.);
#12447=ORIENTED_EDGE('',*,*,#9021,.T.);
#12448=ORIENTED_EDGE('',*,*,#9022,.F.);
#12449=ORIENTED_EDGE('',*,*,#9023,.T.);
#12450=ORIENTED_EDGE('',*,*,#9024,.T.);
#12451=ORIENTED_EDGE('',*,*,#9025,.T.);
#12452=ORIENTED_EDGE('',*,*,#9026,.T.);
#12453=ORIENTED_EDGE('',*,*,#9027,.F.);
#12454=ORIENTED_EDGE('',*,*,#9028,.T.);
#12455=ORIENTED_EDGE('',*,*,#9029,.F.);
#12456=ORIENTED_EDGE('',*,*,#9030,.F.);
#12457=ORIENTED_EDGE('',*,*,#9031,.F.);
#12458=ORIENTED_EDGE('',*,*,#9021,.F.);
#12459=ORIENTED_EDGE('',*,*,#9032,.T.);
#12460=ORIENTED_EDGE('',*,*,#9033,.T.);
#12461=ORIENTED_EDGE('',*,*,#9034,.T.);
#12462=ORIENTED_EDGE('',*,*,#9035,.F.);
#12463=ORIENTED_EDGE('',*,*,#9036,.F.);
#12464=ORIENTED_EDGE('',*,*,#9037,.F.);
#12465=ORIENTED_EDGE('',*,*,#9038,.F.);
#12466=ORIENTED_EDGE('',*,*,#9039,.T.);
#12467=ORIENTED_EDGE('',*,*,#9040,.F.);
#12468=ORIENTED_EDGE('',*,*,#9005,.T.);
#12469=ORIENTED_EDGE('',*,*,#9002,.T.);
#12470=ORIENTED_EDGE('',*,*,#8999,.T.);
#12471=ORIENTED_EDGE('',*,*,#9035,.T.);
#12472=ORIENTED_EDGE('',*,*,#9041,.T.);
#12473=ORIENTED_EDGE('',*,*,#9042,.F.);
#12474=ORIENTED_EDGE('',*,*,#9043,.T.);
#12475=ORIENTED_EDGE('',*,*,#9044,.T.);
#12476=ORIENTED_EDGE('',*,*,#8987,.T.);
#12477=ORIENTED_EDGE('',*,*,#9045,.T.);
#12478=ORIENTED_EDGE('',*,*,#9046,.T.);
#12479=ORIENTED_EDGE('',*,*,#9047,.T.);
#12480=ORIENTED_EDGE('',*,*,#9048,.T.);
#12481=ORIENTED_EDGE('',*,*,#9049,.T.);
#12482=ORIENTED_EDGE('',*,*,#9042,.T.);
#12483=ORIENTED_EDGE('',*,*,#9050,.T.);
#12484=ORIENTED_EDGE('',*,*,#9051,.T.);
#12485=ORIENTED_EDGE('',*,*,#9052,.T.);
#12486=ORIENTED_EDGE('',*,*,#9053,.T.);
#12487=ORIENTED_EDGE('',*,*,#9054,.T.);
#12488=ORIENTED_EDGE('',*,*,#9055,.T.);
#12489=ORIENTED_EDGE('',*,*,#9056,.T.);
#12490=ORIENTED_EDGE('',*,*,#9019,.T.);
#12491=ORIENTED_EDGE('',*,*,#9057,.T.);
#12492=ORIENTED_EDGE('',*,*,#9058,.T.);
#12493=ORIENTED_EDGE('',*,*,#9059,.T.);
#12494=ORIENTED_EDGE('',*,*,#9060,.T.);
#12495=ORIENTED_EDGE('',*,*,#9061,.T.);
#12496=ORIENTED_EDGE('',*,*,#9062,.T.);
#12497=ORIENTED_EDGE('',*,*,#9063,.T.);
#12498=ORIENTED_EDGE('',*,*,#9064,.F.);
#12499=ORIENTED_EDGE('',*,*,#9065,.T.);
#12500=ORIENTED_EDGE('',*,*,#9066,.T.);
#12501=ORIENTED_EDGE('',*,*,#9067,.T.);
#12502=ORIENTED_EDGE('',*,*,#9068,.T.);
#12503=ORIENTED_EDGE('',*,*,#9069,.F.);
#12504=ORIENTED_EDGE('',*,*,#9070,.F.);
#12505=ORIENTED_EDGE('',*,*,#9064,.T.);
#12506=ORIENTED_EDGE('',*,*,#9071,.T.);
#12507=ORIENTED_EDGE('',*,*,#8981,.T.);
#12508=ORIENTED_EDGE('',*,*,#8977,.T.);
#12509=ORIENTED_EDGE('',*,*,#9072,.T.);
#12510=ORIENTED_EDGE('',*,*,#9073,.T.);
#12511=ORIENTED_EDGE('',*,*,#9074,.T.);
#12512=ORIENTED_EDGE('',*,*,#9075,.T.);
#12513=ORIENTED_EDGE('',*,*,#9076,.T.);
#12514=ORIENTED_EDGE('',*,*,#9077,.T.);
#12515=ORIENTED_EDGE('',*,*,#9078,.T.);
#12516=ORIENTED_EDGE('',*,*,#8973,.T.);
#12517=ORIENTED_EDGE('',*,*,#9079,.T.);
#12518=ORIENTED_EDGE('',*,*,#9080,.T.);
#12519=ORIENTED_EDGE('',*,*,#9081,.T.);
#12520=ORIENTED_EDGE('',*,*,#9082,.T.);
#12521=ORIENTED_EDGE('',*,*,#9083,.T.);
#12522=ORIENTED_EDGE('',*,*,#9084,.T.);
#12523=ORIENTED_EDGE('',*,*,#9085,.T.);
#12524=ORIENTED_EDGE('',*,*,#9086,.T.);
#12525=ORIENTED_EDGE('',*,*,#9087,.T.);
#12526=ORIENTED_EDGE('',*,*,#8996,.T.);
#12527=ORIENTED_EDGE('',*,*,#9088,.T.);
#12528=ORIENTED_EDGE('',*,*,#9089,.T.);
#12529=ORIENTED_EDGE('',*,*,#9090,.F.);
#12530=ORIENTED_EDGE('',*,*,#9091,.T.);
#12531=ORIENTED_EDGE('',*,*,#9040,.T.);
#12532=ORIENTED_EDGE('',*,*,#9092,.T.);
#12533=ORIENTED_EDGE('',*,*,#9088,.F.);
#12534=ORIENTED_EDGE('',*,*,#9093,.T.);
#12535=ORIENTED_EDGE('',*,*,#9045,.F.);
#12536=ORIENTED_EDGE('',*,*,#8986,.T.);
#12537=ORIENTED_EDGE('',*,*,#9016,.T.);
#12538=ORIENTED_EDGE('',*,*,#9008,.T.);
#12539=ORIENTED_EDGE('',*,*,#9010,.T.);
#12540=ORIENTED_EDGE('',*,*,#9015,.T.);
#12541=ORIENTED_EDGE('',*,*,#9006,.T.);
#12542=ORIENTED_EDGE('',*,*,#9094,.T.);
#12543=ORIENTED_EDGE('',*,*,#9095,.T.);
#12544=ORIENTED_EDGE('',*,*,#9027,.T.);
#12545=ORIENTED_EDGE('',*,*,#9004,.T.);
#12546=ORIENTED_EDGE('',*,*,#9014,.F.);
#12547=ORIENTED_EDGE('',*,*,#8988,.T.);
#12548=ORIENTED_EDGE('',*,*,#9044,.F.);
#12549=ORIENTED_EDGE('',*,*,#9096,.T.);
#12550=ORIENTED_EDGE('',*,*,#9011,.T.);
#12551=ORIENTED_EDGE('',*,*,#9097,.T.);
#12552=ORIENTED_EDGE('',*,*,#9098,.T.);
#12553=ORIENTED_EDGE('',*,*,#9094,.F.);
#12554=ORIENTED_EDGE('',*,*,#9099,.T.);
#12555=ORIENTED_EDGE('',*,*,#9029,.T.);
#12556=ORIENTED_EDGE('',*,*,#9100,.T.);
#12557=ORIENTED_EDGE('',*,*,#9097,.F.);
#12558=ORIENTED_EDGE('',*,*,#9101,.T.);
#12559=ORIENTED_EDGE('',*,*,#9059,.F.);
#12560=ORIENTED_EDGE('',*,*,#9102,.T.);
#12561=ORIENTED_EDGE('',*,*,#9030,.T.);
#12562=ORIENTED_EDGE('',*,*,#9102,.F.);
#12563=ORIENTED_EDGE('',*,*,#9058,.F.);
#12564=ORIENTED_EDGE('',*,*,#9103,.T.);
#12565=ORIENTED_EDGE('',*,*,#9031,.T.);
#12566=ORIENTED_EDGE('',*,*,#9103,.F.);
#12567=ORIENTED_EDGE('',*,*,#9057,.F.);
#12568=ORIENTED_EDGE('',*,*,#9022,.T.);
#12569=ORIENTED_EDGE('',*,*,#9036,.T.);
#12570=ORIENTED_EDGE('',*,*,#9043,.F.);
#12571=ORIENTED_EDGE('',*,*,#9049,.F.);
#12572=ORIENTED_EDGE('',*,*,#9104,.T.);
#12573=ORIENTED_EDGE('',*,*,#9037,.T.);
#12574=ORIENTED_EDGE('',*,*,#9104,.F.);
#12575=ORIENTED_EDGE('',*,*,#9048,.F.);
#12576=ORIENTED_EDGE('',*,*,#9105,.T.);
#12577=ORIENTED_EDGE('',*,*,#9090,.T.);
#12578=ORIENTED_EDGE('',*,*,#9106,.T.);
#12579=ORIENTED_EDGE('',*,*,#9038,.T.);
#12580=ORIENTED_EDGE('',*,*,#9105,.F.);
#12581=ORIENTED_EDGE('',*,*,#9047,.F.);
#12582=ORIENTED_EDGE('',*,*,#9107,.T.);
#12583=ORIENTED_EDGE('',*,*,#9063,.F.);
#12584=ORIENTED_EDGE('',*,*,#9108,.T.);
#12585=ORIENTED_EDGE('',*,*,#9109,.T.);
#12586=ORIENTED_EDGE('',*,*,#9110,.T.);
#12587=ORIENTED_EDGE('',*,*,#9111,.T.);
#12588=ORIENTED_EDGE('',*,*,#9112,.T.);
#12589=ORIENTED_EDGE('',*,*,#9071,.F.);
#12590=ORIENTED_EDGE('',*,*,#8992,.T.);
#12591=ORIENTED_EDGE('',*,*,#9113,.T.);
#12592=ORIENTED_EDGE('',*,*,#9114,.T.);
#12593=ORIENTED_EDGE('',*,*,#9065,.F.);
#12594=ORIENTED_EDGE('',*,*,#9112,.F.);
#12595=ORIENTED_EDGE('',*,*,#9109,.F.);
#12596=ORIENTED_EDGE('',*,*,#9115,.T.);
#12597=ORIENTED_EDGE('',*,*,#9116,.T.);
#12598=ORIENTED_EDGE('',*,*,#9117,.F.);
#12599=ORIENTED_EDGE('',*,*,#9118,.T.);
#12600=ORIENTED_EDGE('',*,*,#9119,.T.);
#12601=ORIENTED_EDGE('',*,*,#9113,.F.);
#12602=ORIENTED_EDGE('',*,*,#9111,.F.);
#12603=ORIENTED_EDGE('',*,*,#9117,.T.);
#12604=ORIENTED_EDGE('',*,*,#9120,.T.);
#12605=ORIENTED_EDGE('',*,*,#9118,.F.);
#12606=ORIENTED_EDGE('',*,*,#9110,.F.);
#12607=ORIENTED_EDGE('',*,*,#9121,.T.);
#12608=ORIENTED_EDGE('',*,*,#9122,.T.);
#12609=ORIENTED_EDGE('',*,*,#9061,.F.);
#12610=ORIENTED_EDGE('',*,*,#9070,.T.);
#12611=ORIENTED_EDGE('',*,*,#9123,.T.);
#12612=ORIENTED_EDGE('',*,*,#8984,.T.);
#12613=ORIENTED_EDGE('',*,*,#9124,.T.);
#12614=ORIENTED_EDGE('',*,*,#9125,.T.);
#12615=ORIENTED_EDGE('',*,*,#9121,.F.);
#12616=ORIENTED_EDGE('',*,*,#9126,.T.);
#12617=ORIENTED_EDGE('',*,*,#9069,.T.);
#12618=ORIENTED_EDGE('',*,*,#9127,.T.);
#12619=ORIENTED_EDGE('',*,*,#9126,.F.);
#12620=ORIENTED_EDGE('',*,*,#9123,.F.);
#12621=ORIENTED_EDGE('',*,*,#9056,.F.);
#12622=ORIENTED_EDGE('',*,*,#9128,.T.);
#12623=ORIENTED_EDGE('',*,*,#9074,.F.);
#12624=ORIENTED_EDGE('',*,*,#9129,.F.);
#12625=ORIENTED_EDGE('',*,*,#9129,.T.);
#12626=ORIENTED_EDGE('',*,*,#9073,.F.);
#12627=ORIENTED_EDGE('',*,*,#9130,.F.);
#12628=ORIENTED_EDGE('',*,*,#9020,.F.);
#12629=ORIENTED_EDGE('',*,*,#9075,.F.);
#12630=ORIENTED_EDGE('',*,*,#9131,.T.);
#12631=ORIENTED_EDGE('',*,*,#9124,.F.);
#12632=ORIENTED_EDGE('',*,*,#9132,.F.);
#12633=ORIENTED_EDGE('',*,*,#9130,.T.);
#12634=ORIENTED_EDGE('',*,*,#9072,.F.);
#12635=ORIENTED_EDGE('',*,*,#9133,.F.);
#12636=ORIENTED_EDGE('',*,*,#9032,.F.);
#12637=ORIENTED_EDGE('',*,*,#9085,.F.);
#12638=ORIENTED_EDGE('',*,*,#9134,.T.);
#12639=ORIENTED_EDGE('',*,*,#9050,.F.);
#12640=ORIENTED_EDGE('',*,*,#9135,.F.);
#12641=ORIENTED_EDGE('',*,*,#9132,.T.);
#12642=ORIENTED_EDGE('',*,*,#9127,.F.);
#12643=ORIENTED_EDGE('',*,*,#9136,.F.);
#12644=ORIENTED_EDGE('',*,*,#9076,.F.);
#12645=ORIENTED_EDGE('',*,*,#9137,.F.);
#12646=ORIENTED_EDGE('',*,*,#9133,.T.);
#12647=ORIENTED_EDGE('',*,*,#9138,.F.);
#12648=ORIENTED_EDGE('',*,*,#9135,.T.);
#12649=ORIENTED_EDGE('',*,*,#9041,.F.);
#12650=ORIENTED_EDGE('',*,*,#9139,.F.);
#12651=ORIENTED_EDGE('',*,*,#9086,.F.);
#12652=ORIENTED_EDGE('',*,*,#9116,.F.);
#12653=ORIENTED_EDGE('',*,*,#9140,.T.);
#12654=ORIENTED_EDGE('',*,*,#9084,.F.);
#12655=ORIENTED_EDGE('',*,*,#9141,.F.);
#12656=ORIENTED_EDGE('',*,*,#9136,.T.);
#12657=ORIENTED_EDGE('',*,*,#9068,.F.);
#12658=ORIENTED_EDGE('',*,*,#9142,.F.);
#12659=ORIENTED_EDGE('',*,*,#9077,.F.);
#12660=ORIENTED_EDGE('',*,*,#9138,.T.);
#12661=ORIENTED_EDGE('',*,*,#9078,.F.);
#12662=ORIENTED_EDGE('',*,*,#9143,.F.);
#12663=ORIENTED_EDGE('',*,*,#9023,.F.);
#12664=ORIENTED_EDGE('',*,*,#9137,.T.);
#12665=ORIENTED_EDGE('',*,*,#9026,.F.);
#12666=ORIENTED_EDGE('',*,*,#9144,.F.);
#12667=ORIENTED_EDGE('',*,*,#9033,.F.);
#12668=ORIENTED_EDGE('',*,*,#9139,.T.);
#12669=ORIENTED_EDGE('',*,*,#9034,.F.);
#12670=ORIENTED_EDGE('',*,*,#9145,.F.);
#12671=ORIENTED_EDGE('',*,*,#9087,.F.);
#12672=ORIENTED_EDGE('',*,*,#9141,.T.);
#12673=ORIENTED_EDGE('',*,*,#9083,.F.);
#12674=ORIENTED_EDGE('',*,*,#9146,.F.);
#12675=ORIENTED_EDGE('',*,*,#9120,.F.);
#12676=ORIENTED_EDGE('',*,*,#9143,.T.);
#12677=ORIENTED_EDGE('',*,*,#9142,.T.);
#12678=ORIENTED_EDGE('',*,*,#9147,.F.);
#12679=ORIENTED_EDGE('',*,*,#9145,.T.);
#12680=ORIENTED_EDGE('',*,*,#9144,.T.);
#12681=ORIENTED_EDGE('',*,*,#9148,.F.);
#12682=ORIENTED_EDGE('',*,*,#9146,.T.);
#12683=ORIENTED_EDGE('',*,*,#9082,.F.);
#12684=ORIENTED_EDGE('',*,*,#9149,.F.);
#12685=ORIENTED_EDGE('',*,*,#9119,.F.);
#12686=ORIENTED_EDGE('',*,*,#9147,.T.);
#12687=ORIENTED_EDGE('',*,*,#9067,.F.);
#12688=ORIENTED_EDGE('',*,*,#9150,.F.);
#12689=ORIENTED_EDGE('',*,*,#9024,.F.);
#12690=ORIENTED_EDGE('',*,*,#9148,.T.);
#12691=ORIENTED_EDGE('',*,*,#9025,.F.);
#12692=ORIENTED_EDGE('',*,*,#9151,.F.);
#12693=ORIENTED_EDGE('',*,*,#9079,.F.);
#12694=ORIENTED_EDGE('',*,*,#9149,.T.);
#12695=ORIENTED_EDGE('',*,*,#9081,.F.);
#12696=ORIENTED_EDGE('',*,*,#9152,.F.);
#12697=ORIENTED_EDGE('',*,*,#9114,.F.);
#12698=ORIENTED_EDGE('',*,*,#9151,.T.);
#12699=ORIENTED_EDGE('',*,*,#9150,.T.);
#12700=ORIENTED_EDGE('',*,*,#9153,.F.);
#12701=ORIENTED_EDGE('',*,*,#9152,.T.);
#12702=ORIENTED_EDGE('',*,*,#9080,.F.);
#12703=ORIENTED_EDGE('',*,*,#9153,.T.);
#12704=ORIENTED_EDGE('',*,*,#9066,.F.);
#12705=ORIENTED_EDGE('',*,*,#9131,.F.);
#12706=ORIENTED_EDGE('',*,*,#9128,.F.);
#12707=ORIENTED_EDGE('',*,*,#9154,.F.);
#12708=ORIENTED_EDGE('',*,*,#9154,.T.);
#12709=ORIENTED_EDGE('',*,*,#9055,.F.);
#12710=ORIENTED_EDGE('',*,*,#9155,.F.);
#12711=ORIENTED_EDGE('',*,*,#9125,.F.);
#12712=ORIENTED_EDGE('',*,*,#9155,.T.);
#12713=ORIENTED_EDGE('',*,*,#9054,.F.);
#12714=ORIENTED_EDGE('',*,*,#9156,.F.);
#12715=ORIENTED_EDGE('',*,*,#9122,.F.);
#12716=ORIENTED_EDGE('',*,*,#9156,.T.);
#12717=ORIENTED_EDGE('',*,*,#9053,.F.);
#12718=ORIENTED_EDGE('',*,*,#9157,.F.);
#12719=ORIENTED_EDGE('',*,*,#9062,.F.);
#12720=ORIENTED_EDGE('',*,*,#9157,.T.);
#12721=ORIENTED_EDGE('',*,*,#9052,.F.);
#12722=ORIENTED_EDGE('',*,*,#9158,.F.);
#12723=ORIENTED_EDGE('',*,*,#9108,.F.);
#12724=ORIENTED_EDGE('',*,*,#9158,.T.);
#12725=ORIENTED_EDGE('',*,*,#9051,.F.);
#12726=ORIENTED_EDGE('',*,*,#9159,.F.);
#12727=ORIENTED_EDGE('',*,*,#9115,.F.);
#12728=ORIENTED_EDGE('',*,*,#9159,.T.);
#12729=ORIENTED_EDGE('',*,*,#9134,.F.);
#12730=ORIENTED_EDGE('',*,*,#9140,.F.);
#12731=ORIENTED_EDGE('',*,*,#9100,.F.);
#12732=ORIENTED_EDGE('',*,*,#9028,.F.);
#12733=ORIENTED_EDGE('',*,*,#9095,.F.);
#12734=ORIENTED_EDGE('',*,*,#9098,.F.);
#12735=ORIENTED_EDGE('',*,*,#9092,.F.);
#12736=ORIENTED_EDGE('',*,*,#9039,.F.);
#12737=ORIENTED_EDGE('',*,*,#9106,.F.);
#12738=ORIENTED_EDGE('',*,*,#9089,.F.);
#12739=ORIENTED_EDGE('',*,*,#9101,.F.);
#12740=ORIENTED_EDGE('',*,*,#9099,.F.);
#12741=ORIENTED_EDGE('',*,*,#9096,.F.);
#12742=ORIENTED_EDGE('',*,*,#9060,.F.);
#12743=ORIENTED_EDGE('',*,*,#9093,.F.);
#12744=ORIENTED_EDGE('',*,*,#9091,.F.);
#12745=ORIENTED_EDGE('',*,*,#9107,.F.);
#12746=ORIENTED_EDGE('',*,*,#9046,.F.);
#12747=ORIENTED_EDGE('',*,*,#9160,.F.);
#12748=ORIENTED_EDGE('',*,*,#9161,.T.);
#12749=ORIENTED_EDGE('',*,*,#9162,.F.);
#12750=ORIENTED_EDGE('',*,*,#9163,.F.);
#12751=ORIENTED_EDGE('',*,*,#9161,.F.);
#12752=ORIENTED_EDGE('',*,*,#9164,.F.);
#12753=ORIENTED_EDGE('',*,*,#9165,.F.);
#12754=ORIENTED_EDGE('',*,*,#9166,.T.);
#12755=ORIENTED_EDGE('',*,*,#9167,.F.);
#12756=ORIENTED_EDGE('',*,*,#9166,.F.);
#12757=ORIENTED_EDGE('',*,*,#9164,.T.);
#12758=ORIENTED_EDGE('',*,*,#9165,.T.);
#12759=ORIENTED_EDGE('',*,*,#9168,.T.);
#12760=ORIENTED_EDGE('',*,*,#9162,.T.);
#12761=ORIENTED_EDGE('',*,*,#9163,.T.);
#12762=ORIENTED_EDGE('',*,*,#9168,.F.);
#12763=ORIENTED_EDGE('',*,*,#9160,.T.);
#12764=ORIENTED_EDGE('',*,*,#9167,.T.);
#12765=ORIENTED_EDGE('',*,*,#9169,.T.);
#12766=ORIENTED_EDGE('',*,*,#9170,.T.);
#12767=ORIENTED_EDGE('',*,*,#9171,.F.);
#12768=ORIENTED_EDGE('',*,*,#9170,.F.);
#12769=ORIENTED_EDGE('',*,*,#9172,.T.);
#12770=ORIENTED_EDGE('',*,*,#9173,.T.);
#12771=ORIENTED_EDGE('',*,*,#9174,.T.);
#12772=ORIENTED_EDGE('',*,*,#9175,.F.);
#12773=ORIENTED_EDGE('',*,*,#9174,.F.);
#12774=ORIENTED_EDGE('',*,*,#9176,.T.);
#12775=ORIENTED_EDGE('',*,*,#9177,.F.);
#12776=ORIENTED_EDGE('',*,*,#9178,.T.);
#12777=ORIENTED_EDGE('',*,*,#9179,.T.);
#12778=ORIENTED_EDGE('',*,*,#9178,.F.);
#12779=ORIENTED_EDGE('',*,*,#9180,.F.);
#12780=ORIENTED_EDGE('',*,*,#9181,.T.);
#12781=ORIENTED_EDGE('',*,*,#9182,.F.);
#12782=ORIENTED_EDGE('',*,*,#9181,.F.);
#12783=ORIENTED_EDGE('',*,*,#9183,.T.);
#12784=ORIENTED_EDGE('',*,*,#9184,.T.);
#12785=ORIENTED_EDGE('',*,*,#9185,.F.);
#12786=ORIENTED_EDGE('',*,*,#9184,.F.);
#12787=ORIENTED_EDGE('',*,*,#9186,.F.);
#12788=ORIENTED_EDGE('',*,*,#9187,.T.);
#12789=ORIENTED_EDGE('',*,*,#9188,.F.);
#12790=ORIENTED_EDGE('',*,*,#9187,.F.);
#12791=ORIENTED_EDGE('',*,*,#9172,.F.);
#12792=ORIENTED_EDGE('',*,*,#9189,.F.);
#12793=ORIENTED_EDGE('',*,*,#9190,.F.);
#12794=ORIENTED_EDGE('',*,*,#9191,.T.);
#12795=ORIENTED_EDGE('',*,*,#9192,.T.);
#12796=ORIENTED_EDGE('',*,*,#9193,.T.);
#12797=ORIENTED_EDGE('',*,*,#9194,.F.);
#12798=ORIENTED_EDGE('',*,*,#9195,.F.);
#12799=ORIENTED_EDGE('',*,*,#9194,.T.);
#12800=ORIENTED_EDGE('',*,*,#9196,.T.);
#12801=ORIENTED_EDGE('',*,*,#9197,.F.);
#12802=ORIENTED_EDGE('',*,*,#9198,.F.);
#12803=ORIENTED_EDGE('',*,*,#9190,.T.);
#12804=ORIENTED_EDGE('',*,*,#9199,.T.);
#12805=ORIENTED_EDGE('',*,*,#9195,.T.);
#12806=ORIENTED_EDGE('',*,*,#9198,.T.);
#12807=ORIENTED_EDGE('',*,*,#9200,.T.);
#12808=ORIENTED_EDGE('',*,*,#9183,.F.);
#12809=ORIENTED_EDGE('',*,*,#9201,.F.);
#12810=ORIENTED_EDGE('',*,*,#9202,.F.);
#12811=ORIENTED_EDGE('',*,*,#9203,.F.);
#12812=ORIENTED_EDGE('',*,*,#9204,.F.);
#12813=ORIENTED_EDGE('',*,*,#9205,.F.);
#12814=ORIENTED_EDGE('',*,*,#9182,.T.);
#12815=ORIENTED_EDGE('',*,*,#9173,.F.);
#12816=ORIENTED_EDGE('',*,*,#9206,.T.);
#12817=ORIENTED_EDGE('',*,*,#9201,.T.);
#12818=ORIENTED_EDGE('',*,*,#9207,.F.);
#12819=ORIENTED_EDGE('',*,*,#9176,.F.);
#12820=ORIENTED_EDGE('',*,*,#9208,.F.);
#12821=ORIENTED_EDGE('',*,*,#9209,.F.);
#12822=ORIENTED_EDGE('',*,*,#9192,.F.);
#12823=ORIENTED_EDGE('',*,*,#9199,.F.);
#12824=ORIENTED_EDGE('',*,*,#9189,.T.);
#12825=ORIENTED_EDGE('',*,*,#9207,.T.);
#12826=ORIENTED_EDGE('',*,*,#9205,.T.);
#12827=ORIENTED_EDGE('',*,*,#9210,.F.);
#12828=ORIENTED_EDGE('',*,*,#9211,.F.);
#12829=ORIENTED_EDGE('',*,*,#9186,.T.);
#12830=ORIENTED_EDGE('',*,*,#9212,.F.);
#12831=ORIENTED_EDGE('',*,*,#9213,.T.);
#12832=ORIENTED_EDGE('',*,*,#9210,.T.);
#12833=ORIENTED_EDGE('',*,*,#9204,.T.);
#12834=ORIENTED_EDGE('',*,*,#9214,.F.);
#12835=ORIENTED_EDGE('',*,*,#9215,.T.);
#12836=ORIENTED_EDGE('',*,*,#9212,.T.);
#12837=ORIENTED_EDGE('',*,*,#9203,.T.);
#12838=ORIENTED_EDGE('',*,*,#9197,.T.);
#12839=ORIENTED_EDGE('',*,*,#9216,.T.);
#12840=ORIENTED_EDGE('',*,*,#9217,.T.);
#12841=ORIENTED_EDGE('',*,*,#9218,.T.);
#12842=ORIENTED_EDGE('',*,*,#9214,.T.);
#12843=ORIENTED_EDGE('',*,*,#9202,.T.);
#12844=ORIENTED_EDGE('',*,*,#9206,.F.);
#12845=ORIENTED_EDGE('',*,*,#9191,.F.);
#12846=ORIENTED_EDGE('',*,*,#9200,.F.);
#12847=ORIENTED_EDGE('',*,*,#9179,.F.);
#12848=ORIENTED_EDGE('',*,*,#9209,.T.);
#12849=ORIENTED_EDGE('',*,*,#9219,.F.);
#12850=ORIENTED_EDGE('',*,*,#9216,.F.);
#12851=ORIENTED_EDGE('',*,*,#9196,.F.);
#12852=ORIENTED_EDGE('',*,*,#9193,.F.);
#12853=ORIENTED_EDGE('',*,*,#9185,.T.);
#12854=ORIENTED_EDGE('',*,*,#9215,.F.);
#12855=ORIENTED_EDGE('',*,*,#9218,.F.);
#12856=ORIENTED_EDGE('',*,*,#9220,.T.);
#12857=ORIENTED_EDGE('',*,*,#9211,.T.);
#12858=ORIENTED_EDGE('',*,*,#9213,.F.);
#12859=ORIENTED_EDGE('',*,*,#9180,.T.);
#12860=ORIENTED_EDGE('',*,*,#9208,.T.);
#12861=ORIENTED_EDGE('',*,*,#9220,.F.);
#12862=ORIENTED_EDGE('',*,*,#9217,.F.);
#12863=ORIENTED_EDGE('',*,*,#9219,.T.);
#12864=ORIENTED_EDGE('',*,*,#9177,.T.);
#12865=ORIENTED_EDGE('',*,*,#9188,.T.);
#12866=ORIENTED_EDGE('',*,*,#9175,.T.);
#12867=ORIENTED_EDGE('',*,*,#9169,.F.);
#12868=ORIENTED_EDGE('',*,*,#9171,.T.);
#12869=ORIENTED_EDGE('',*,*,#9221,.F.);
#12870=ORIENTED_EDGE('',*,*,#9222,.T.);
#12871=ORIENTED_EDGE('',*,*,#9223,.T.);
#12872=ORIENTED_EDGE('',*,*,#9222,.F.);
#12873=ORIENTED_EDGE('',*,*,#9224,.T.);
#12874=ORIENTED_EDGE('',*,*,#9224,.F.);
#12875=ORIENTED_EDGE('',*,*,#9221,.T.);
#12876=ORIENTED_EDGE('',*,*,#9223,.F.);
#12877=ORIENTED_EDGE('',*,*,#9225,.F.);
#12878=ORIENTED_EDGE('',*,*,#9226,.T.);
#12879=ORIENTED_EDGE('',*,*,#9227,.F.);
#12880=ORIENTED_EDGE('',*,*,#9226,.F.);
#12881=ORIENTED_EDGE('',*,*,#9228,.F.);
#12882=ORIENTED_EDGE('',*,*,#9229,.F.);
#12883=ORIENTED_EDGE('',*,*,#9230,.T.);
#12884=ORIENTED_EDGE('',*,*,#9231,.T.);
#12885=ORIENTED_EDGE('',*,*,#9230,.F.);
#12886=ORIENTED_EDGE('',*,*,#9232,.F.);
#12887=ORIENTED_EDGE('',*,*,#9233,.F.);
#12888=ORIENTED_EDGE('',*,*,#9234,.T.);
#12889=ORIENTED_EDGE('',*,*,#9235,.T.);
#12890=ORIENTED_EDGE('',*,*,#9236,.T.);
#12891=ORIENTED_EDGE('',*,*,#9234,.F.);
#12892=ORIENTED_EDGE('',*,*,#9228,.T.);
#12893=ORIENTED_EDGE('',*,*,#9229,.T.);
#12894=ORIENTED_EDGE('',*,*,#9237,.T.);
#12895=ORIENTED_EDGE('',*,*,#9235,.F.);
#12896=ORIENTED_EDGE('',*,*,#9236,.F.);
#12897=ORIENTED_EDGE('',*,*,#9237,.F.);
#12898=ORIENTED_EDGE('',*,*,#9238,.F.);
#12899=ORIENTED_EDGE('',*,*,#9239,.F.);
#12900=ORIENTED_EDGE('',*,*,#9240,.T.);
#12901=ORIENTED_EDGE('',*,*,#9232,.T.);
#12902=ORIENTED_EDGE('',*,*,#9233,.T.);
#12903=ORIENTED_EDGE('',*,*,#9240,.F.);
#12904=ORIENTED_EDGE('',*,*,#9241,.F.);
#12905=ORIENTED_EDGE('',*,*,#9242,.F.);
#12906=ORIENTED_EDGE('',*,*,#9243,.T.);
#12907=ORIENTED_EDGE('',*,*,#9244,.T.);
#12908=ORIENTED_EDGE('',*,*,#9245,.T.);
#12909=ORIENTED_EDGE('',*,*,#9243,.F.);
#12910=ORIENTED_EDGE('',*,*,#9238,.T.);
#12911=ORIENTED_EDGE('',*,*,#9239,.T.);
#12912=ORIENTED_EDGE('',*,*,#9246,.T.);
#12913=ORIENTED_EDGE('',*,*,#9244,.F.);
#12914=ORIENTED_EDGE('',*,*,#9245,.F.);
#12915=ORIENTED_EDGE('',*,*,#9246,.F.);
#12916=ORIENTED_EDGE('',*,*,#9247,.F.);
#12917=ORIENTED_EDGE('',*,*,#9248,.F.);
#12918=ORIENTED_EDGE('',*,*,#9249,.T.);
#12919=ORIENTED_EDGE('',*,*,#9241,.T.);
#12920=ORIENTED_EDGE('',*,*,#9242,.T.);
#12921=ORIENTED_EDGE('',*,*,#9249,.F.);
#12922=ORIENTED_EDGE('',*,*,#9250,.F.);
#12923=ORIENTED_EDGE('',*,*,#9251,.F.);
#12924=ORIENTED_EDGE('',*,*,#9252,.T.);
#12925=ORIENTED_EDGE('',*,*,#9253,.T.);
#12926=ORIENTED_EDGE('',*,*,#9254,.T.);
#12927=ORIENTED_EDGE('',*,*,#9252,.F.);
#12928=ORIENTED_EDGE('',*,*,#9247,.T.);
#12929=ORIENTED_EDGE('',*,*,#9248,.T.);
#12930=ORIENTED_EDGE('',*,*,#9255,.T.);
#12931=ORIENTED_EDGE('',*,*,#9253,.F.);
#12932=ORIENTED_EDGE('',*,*,#9254,.F.);
#12933=ORIENTED_EDGE('',*,*,#9255,.F.);
#12934=ORIENTED_EDGE('',*,*,#9256,.F.);
#12935=ORIENTED_EDGE('',*,*,#9257,.F.);
#12936=ORIENTED_EDGE('',*,*,#9258,.T.);
#12937=ORIENTED_EDGE('',*,*,#9250,.T.);
#12938=ORIENTED_EDGE('',*,*,#9251,.T.);
#12939=ORIENTED_EDGE('',*,*,#9258,.F.);
#12940=ORIENTED_EDGE('',*,*,#9259,.F.);
#12941=ORIENTED_EDGE('',*,*,#9260,.F.);
#12942=ORIENTED_EDGE('',*,*,#9261,.T.);
#12943=ORIENTED_EDGE('',*,*,#9262,.T.);
#12944=ORIENTED_EDGE('',*,*,#9263,.T.);
#12945=ORIENTED_EDGE('',*,*,#9261,.F.);
#12946=ORIENTED_EDGE('',*,*,#9256,.T.);
#12947=ORIENTED_EDGE('',*,*,#9257,.T.);
#12948=ORIENTED_EDGE('',*,*,#9264,.T.);
#12949=ORIENTED_EDGE('',*,*,#9262,.F.);
#12950=ORIENTED_EDGE('',*,*,#9263,.F.);
#12951=ORIENTED_EDGE('',*,*,#9264,.F.);
#12952=ORIENTED_EDGE('',*,*,#9265,.F.);
#12953=ORIENTED_EDGE('',*,*,#9266,.F.);
#12954=ORIENTED_EDGE('',*,*,#9267,.T.);
#12955=ORIENTED_EDGE('',*,*,#9259,.T.);
#12956=ORIENTED_EDGE('',*,*,#9260,.T.);
#12957=ORIENTED_EDGE('',*,*,#9267,.F.);
#12958=ORIENTED_EDGE('',*,*,#9268,.F.);
#12959=ORIENTED_EDGE('',*,*,#9269,.F.);
#12960=ORIENTED_EDGE('',*,*,#9270,.T.);
#12961=ORIENTED_EDGE('',*,*,#9271,.T.);
#12962=ORIENTED_EDGE('',*,*,#9272,.T.);
#12963=ORIENTED_EDGE('',*,*,#9270,.F.);
#12964=ORIENTED_EDGE('',*,*,#9265,.T.);
#12965=ORIENTED_EDGE('',*,*,#9266,.T.);
#12966=ORIENTED_EDGE('',*,*,#9273,.T.);
#12967=ORIENTED_EDGE('',*,*,#9271,.F.);
#12968=ORIENTED_EDGE('',*,*,#9272,.F.);
#12969=ORIENTED_EDGE('',*,*,#9273,.F.);
#12970=ORIENTED_EDGE('',*,*,#9274,.F.);
#12971=ORIENTED_EDGE('',*,*,#9275,.F.);
#12972=ORIENTED_EDGE('',*,*,#9276,.T.);
#12973=ORIENTED_EDGE('',*,*,#9268,.T.);
#12974=ORIENTED_EDGE('',*,*,#9269,.T.);
#12975=ORIENTED_EDGE('',*,*,#9276,.F.);
#12976=ORIENTED_EDGE('',*,*,#9277,.F.);
#12977=ORIENTED_EDGE('',*,*,#9278,.F.);
#12978=ORIENTED_EDGE('',*,*,#9279,.T.);
#12979=ORIENTED_EDGE('',*,*,#9280,.T.);
#12980=ORIENTED_EDGE('',*,*,#9281,.T.);
#12981=ORIENTED_EDGE('',*,*,#9279,.F.);
#12982=ORIENTED_EDGE('',*,*,#9274,.T.);
#12983=ORIENTED_EDGE('',*,*,#9275,.T.);
#12984=ORIENTED_EDGE('',*,*,#9282,.T.);
#12985=ORIENTED_EDGE('',*,*,#9280,.F.);
#12986=ORIENTED_EDGE('',*,*,#9281,.F.);
#12987=ORIENTED_EDGE('',*,*,#9282,.F.);
#12988=ORIENTED_EDGE('',*,*,#9283,.F.);
#12989=ORIENTED_EDGE('',*,*,#9284,.F.);
#12990=ORIENTED_EDGE('',*,*,#9285,.T.);
#12991=ORIENTED_EDGE('',*,*,#9277,.T.);
#12992=ORIENTED_EDGE('',*,*,#9278,.T.);
#12993=ORIENTED_EDGE('',*,*,#9285,.F.);
#12994=ORIENTED_EDGE('',*,*,#9286,.F.);
#12995=ORIENTED_EDGE('',*,*,#9287,.F.);
#12996=ORIENTED_EDGE('',*,*,#9288,.T.);
#12997=ORIENTED_EDGE('',*,*,#9289,.T.);
#12998=ORIENTED_EDGE('',*,*,#9290,.T.);
#12999=ORIENTED_EDGE('',*,*,#9288,.F.);
#13000=ORIENTED_EDGE('',*,*,#9283,.T.);
#13001=ORIENTED_EDGE('',*,*,#9284,.T.);
#13002=ORIENTED_EDGE('',*,*,#9291,.T.);
#13003=ORIENTED_EDGE('',*,*,#9289,.F.);
#13004=ORIENTED_EDGE('',*,*,#9290,.F.);
#13005=ORIENTED_EDGE('',*,*,#9291,.F.);
#13006=ORIENTED_EDGE('',*,*,#9292,.F.);
#13007=ORIENTED_EDGE('',*,*,#9293,.F.);
#13008=ORIENTED_EDGE('',*,*,#9294,.T.);
#13009=ORIENTED_EDGE('',*,*,#9286,.T.);
#13010=ORIENTED_EDGE('',*,*,#9287,.T.);
#13011=ORIENTED_EDGE('',*,*,#9294,.F.);
#13012=ORIENTED_EDGE('',*,*,#9295,.F.);
#13013=ORIENTED_EDGE('',*,*,#9296,.F.);
#13014=ORIENTED_EDGE('',*,*,#9297,.T.);
#13015=ORIENTED_EDGE('',*,*,#9298,.T.);
#13016=ORIENTED_EDGE('',*,*,#9299,.T.);
#13017=ORIENTED_EDGE('',*,*,#9297,.F.);
#13018=ORIENTED_EDGE('',*,*,#9292,.T.);
#13019=ORIENTED_EDGE('',*,*,#9293,.T.);
#13020=ORIENTED_EDGE('',*,*,#9300,.T.);
#13021=ORIENTED_EDGE('',*,*,#9298,.F.);
#13022=ORIENTED_EDGE('',*,*,#9299,.F.);
#13023=ORIENTED_EDGE('',*,*,#9300,.F.);
#13024=ORIENTED_EDGE('',*,*,#9301,.F.);
#13025=ORIENTED_EDGE('',*,*,#9302,.F.);
#13026=ORIENTED_EDGE('',*,*,#9303,.T.);
#13027=ORIENTED_EDGE('',*,*,#9295,.T.);
#13028=ORIENTED_EDGE('',*,*,#9296,.T.);
#13029=ORIENTED_EDGE('',*,*,#9303,.F.);
#13030=ORIENTED_EDGE('',*,*,#9304,.F.);
#13031=ORIENTED_EDGE('',*,*,#9305,.F.);
#13032=ORIENTED_EDGE('',*,*,#9306,.T.);
#13033=ORIENTED_EDGE('',*,*,#9307,.T.);
#13034=ORIENTED_EDGE('',*,*,#9308,.T.);
#13035=ORIENTED_EDGE('',*,*,#9306,.F.);
#13036=ORIENTED_EDGE('',*,*,#9301,.T.);
#13037=ORIENTED_EDGE('',*,*,#9302,.T.);
#13038=ORIENTED_EDGE('',*,*,#9309,.T.);
#13039=ORIENTED_EDGE('',*,*,#9307,.F.);
#13040=ORIENTED_EDGE('',*,*,#9308,.F.);
#13041=ORIENTED_EDGE('',*,*,#9309,.F.);
#13042=ORIENTED_EDGE('',*,*,#9310,.F.);
#13043=ORIENTED_EDGE('',*,*,#9311,.F.);
#13044=ORIENTED_EDGE('',*,*,#9312,.T.);
#13045=ORIENTED_EDGE('',*,*,#9304,.T.);
#13046=ORIENTED_EDGE('',*,*,#9305,.T.);
#13047=ORIENTED_EDGE('',*,*,#9312,.F.);
#13048=ORIENTED_EDGE('',*,*,#9313,.F.);
#13049=ORIENTED_EDGE('',*,*,#9314,.F.);
#13050=ORIENTED_EDGE('',*,*,#9315,.T.);
#13051=ORIENTED_EDGE('',*,*,#9316,.T.);
#13052=ORIENTED_EDGE('',*,*,#9317,.T.);
#13053=ORIENTED_EDGE('',*,*,#9315,.F.);
#13054=ORIENTED_EDGE('',*,*,#9310,.T.);
#13055=ORIENTED_EDGE('',*,*,#9311,.T.);
#13056=ORIENTED_EDGE('',*,*,#9318,.T.);
#13057=ORIENTED_EDGE('',*,*,#9316,.F.);
#13058=ORIENTED_EDGE('',*,*,#9317,.F.);
#13059=ORIENTED_EDGE('',*,*,#9318,.F.);
#13060=ORIENTED_EDGE('',*,*,#9319,.F.);
#13061=ORIENTED_EDGE('',*,*,#9320,.F.);
#13062=ORIENTED_EDGE('',*,*,#9321,.T.);
#13063=ORIENTED_EDGE('',*,*,#9313,.T.);
#13064=ORIENTED_EDGE('',*,*,#9314,.T.);
#13065=ORIENTED_EDGE('',*,*,#9321,.F.);
#13066=ORIENTED_EDGE('',*,*,#9322,.F.);
#13067=ORIENTED_EDGE('',*,*,#9323,.F.);
#13068=ORIENTED_EDGE('',*,*,#9324,.T.);
#13069=ORIENTED_EDGE('',*,*,#9325,.T.);
#13070=ORIENTED_EDGE('',*,*,#9326,.T.);
#13071=ORIENTED_EDGE('',*,*,#9324,.F.);
#13072=ORIENTED_EDGE('',*,*,#9319,.T.);
#13073=ORIENTED_EDGE('',*,*,#9320,.T.);
#13074=ORIENTED_EDGE('',*,*,#9327,.T.);
#13075=ORIENTED_EDGE('',*,*,#9325,.F.);
#13076=ORIENTED_EDGE('',*,*,#9326,.F.);
#13077=ORIENTED_EDGE('',*,*,#9327,.F.);
#13078=ORIENTED_EDGE('',*,*,#9328,.F.);
#13079=ORIENTED_EDGE('',*,*,#9329,.F.);
#13080=ORIENTED_EDGE('',*,*,#9330,.T.);
#13081=ORIENTED_EDGE('',*,*,#9322,.T.);
#13082=ORIENTED_EDGE('',*,*,#9323,.T.);
#13083=ORIENTED_EDGE('',*,*,#9330,.F.);
#13084=ORIENTED_EDGE('',*,*,#9331,.F.);
#13085=ORIENTED_EDGE('',*,*,#9332,.F.);
#13086=ORIENTED_EDGE('',*,*,#9333,.T.);
#13087=ORIENTED_EDGE('',*,*,#9334,.T.);
#13088=ORIENTED_EDGE('',*,*,#9335,.T.);
#13089=ORIENTED_EDGE('',*,*,#9333,.F.);
#13090=ORIENTED_EDGE('',*,*,#9328,.T.);
#13091=ORIENTED_EDGE('',*,*,#9329,.T.);
#13092=ORIENTED_EDGE('',*,*,#9336,.T.);
#13093=ORIENTED_EDGE('',*,*,#9334,.F.);
#13094=ORIENTED_EDGE('',*,*,#9335,.F.);
#13095=ORIENTED_EDGE('',*,*,#9336,.F.);
#13096=ORIENTED_EDGE('',*,*,#9337,.F.);
#13097=ORIENTED_EDGE('',*,*,#9338,.F.);
#13098=ORIENTED_EDGE('',*,*,#9339,.T.);
#13099=ORIENTED_EDGE('',*,*,#9331,.T.);
#13100=ORIENTED_EDGE('',*,*,#9332,.T.);
#13101=ORIENTED_EDGE('',*,*,#9339,.F.);
#13102=ORIENTED_EDGE('',*,*,#9340,.F.);
#13103=ORIENTED_EDGE('',*,*,#9341,.F.);
#13104=ORIENTED_EDGE('',*,*,#9342,.T.);
#13105=ORIENTED_EDGE('',*,*,#9343,.T.);
#13106=ORIENTED_EDGE('',*,*,#9344,.T.);
#13107=ORIENTED_EDGE('',*,*,#9342,.F.);
#13108=ORIENTED_EDGE('',*,*,#9337,.T.);
#13109=ORIENTED_EDGE('',*,*,#9338,.T.);
#13110=ORIENTED_EDGE('',*,*,#9345,.T.);
#13111=ORIENTED_EDGE('',*,*,#9343,.F.);
#13112=ORIENTED_EDGE('',*,*,#9344,.F.);
#13113=ORIENTED_EDGE('',*,*,#9345,.F.);
#13114=ORIENTED_EDGE('',*,*,#9346,.F.);
#13115=ORIENTED_EDGE('',*,*,#9347,.F.);
#13116=ORIENTED_EDGE('',*,*,#9348,.T.);
#13117=ORIENTED_EDGE('',*,*,#9340,.T.);
#13118=ORIENTED_EDGE('',*,*,#9341,.T.);
#13119=ORIENTED_EDGE('',*,*,#9348,.F.);
#13120=ORIENTED_EDGE('',*,*,#9349,.F.);
#13121=ORIENTED_EDGE('',*,*,#9350,.F.);
#13122=ORIENTED_EDGE('',*,*,#9351,.T.);
#13123=ORIENTED_EDGE('',*,*,#9352,.T.);
#13124=ORIENTED_EDGE('',*,*,#9353,.T.);
#13125=ORIENTED_EDGE('',*,*,#9351,.F.);
#13126=ORIENTED_EDGE('',*,*,#9346,.T.);
#13127=ORIENTED_EDGE('',*,*,#9347,.T.);
#13128=ORIENTED_EDGE('',*,*,#9354,.T.);
#13129=ORIENTED_EDGE('',*,*,#9352,.F.);
#13130=ORIENTED_EDGE('',*,*,#9353,.F.);
#13131=ORIENTED_EDGE('',*,*,#9354,.F.);
#13132=ORIENTED_EDGE('',*,*,#9355,.F.);
#13133=ORIENTED_EDGE('',*,*,#9356,.F.);
#13134=ORIENTED_EDGE('',*,*,#9357,.T.);
#13135=ORIENTED_EDGE('',*,*,#9349,.T.);
#13136=ORIENTED_EDGE('',*,*,#9350,.T.);
#13137=ORIENTED_EDGE('',*,*,#9357,.F.);
#13138=ORIENTED_EDGE('',*,*,#9358,.F.);
#13139=ORIENTED_EDGE('',*,*,#9359,.F.);
#13140=ORIENTED_EDGE('',*,*,#9360,.T.);
#13141=ORIENTED_EDGE('',*,*,#9361,.T.);
#13142=ORIENTED_EDGE('',*,*,#9362,.T.);
#13143=ORIENTED_EDGE('',*,*,#9360,.F.);
#13144=ORIENTED_EDGE('',*,*,#9355,.T.);
#13145=ORIENTED_EDGE('',*,*,#9356,.T.);
#13146=ORIENTED_EDGE('',*,*,#9363,.T.);
#13147=ORIENTED_EDGE('',*,*,#9361,.F.);
#13148=ORIENTED_EDGE('',*,*,#9362,.F.);
#13149=ORIENTED_EDGE('',*,*,#9363,.F.);
#13150=ORIENTED_EDGE('',*,*,#9364,.F.);
#13151=ORIENTED_EDGE('',*,*,#9365,.T.);
#13152=ORIENTED_EDGE('',*,*,#9366,.F.);
#13153=ORIENTED_EDGE('',*,*,#9367,.F.);
#13154=ORIENTED_EDGE('',*,*,#9368,.T.);
#13155=ORIENTED_EDGE('',*,*,#9369,.F.);
#13156=ORIENTED_EDGE('',*,*,#9370,.F.);
#13157=ORIENTED_EDGE('',*,*,#9371,.T.);
#13158=ORIENTED_EDGE('',*,*,#9372,.F.);
#13159=ORIENTED_EDGE('',*,*,#9373,.F.);
#13160=ORIENTED_EDGE('',*,*,#9374,.T.);
#13161=ORIENTED_EDGE('',*,*,#9375,.F.);
#13162=ORIENTED_EDGE('',*,*,#9376,.F.);
#13163=ORIENTED_EDGE('',*,*,#9377,.T.);
#13164=ORIENTED_EDGE('',*,*,#9378,.F.);
#13165=ORIENTED_EDGE('',*,*,#9379,.F.);
#13166=ORIENTED_EDGE('',*,*,#9380,.T.);
#13167=ORIENTED_EDGE('',*,*,#9381,.F.);
#13168=ORIENTED_EDGE('',*,*,#9382,.F.);
#13169=ORIENTED_EDGE('',*,*,#9383,.T.);
#13170=ORIENTED_EDGE('',*,*,#9384,.F.);
#13171=ORIENTED_EDGE('',*,*,#9385,.F.);
#13172=ORIENTED_EDGE('',*,*,#9386,.T.);
#13173=ORIENTED_EDGE('',*,*,#9387,.F.);
#13174=ORIENTED_EDGE('',*,*,#9388,.F.);
#13175=ORIENTED_EDGE('',*,*,#9389,.T.);
#13176=ORIENTED_EDGE('',*,*,#9390,.F.);
#13177=ORIENTED_EDGE('',*,*,#9391,.F.);
#13178=ORIENTED_EDGE('',*,*,#9392,.T.);
#13179=ORIENTED_EDGE('',*,*,#9393,.F.);
#13180=ORIENTED_EDGE('',*,*,#9394,.F.);
#13181=ORIENTED_EDGE('',*,*,#9395,.T.);
#13182=ORIENTED_EDGE('',*,*,#9396,.F.);
#13183=ORIENTED_EDGE('',*,*,#9397,.F.);
#13184=ORIENTED_EDGE('',*,*,#9398,.T.);
#13185=ORIENTED_EDGE('',*,*,#9399,.F.);
#13186=ORIENTED_EDGE('',*,*,#9400,.F.);
#13187=ORIENTED_EDGE('',*,*,#9401,.T.);
#13188=ORIENTED_EDGE('',*,*,#9402,.F.);
#13189=ORIENTED_EDGE('',*,*,#9403,.F.);
#13190=ORIENTED_EDGE('',*,*,#9404,.T.);
#13191=ORIENTED_EDGE('',*,*,#9405,.F.);
#13192=ORIENTED_EDGE('',*,*,#9406,.F.);
#13193=ORIENTED_EDGE('',*,*,#9407,.T.);
#13194=ORIENTED_EDGE('',*,*,#9408,.F.);
#13195=ORIENTED_EDGE('',*,*,#9409,.F.);
#13196=ORIENTED_EDGE('',*,*,#9410,.T.);
#13197=ORIENTED_EDGE('',*,*,#9411,.F.);
#13198=ORIENTED_EDGE('',*,*,#9412,.F.);
#13199=ORIENTED_EDGE('',*,*,#9413,.T.);
#13200=ORIENTED_EDGE('',*,*,#9414,.F.);
#13201=ORIENTED_EDGE('',*,*,#9415,.F.);
#13202=ORIENTED_EDGE('',*,*,#9416,.T.);
#13203=ORIENTED_EDGE('',*,*,#9417,.F.);
#13204=ORIENTED_EDGE('',*,*,#9418,.F.);
#13205=ORIENTED_EDGE('',*,*,#9419,.T.);
#13206=ORIENTED_EDGE('',*,*,#9420,.F.);
#13207=ORIENTED_EDGE('',*,*,#9421,.F.);
#13208=ORIENTED_EDGE('',*,*,#9422,.T.);
#13209=ORIENTED_EDGE('',*,*,#9423,.F.);
#13210=ORIENTED_EDGE('',*,*,#9424,.F.);
#13211=ORIENTED_EDGE('',*,*,#9425,.T.);
#13212=ORIENTED_EDGE('',*,*,#9426,.F.);
#13213=ORIENTED_EDGE('',*,*,#9427,.F.);
#13214=ORIENTED_EDGE('',*,*,#9428,.T.);
#13215=ORIENTED_EDGE('',*,*,#9429,.F.);
#13216=ORIENTED_EDGE('',*,*,#9430,.F.);
#13217=ORIENTED_EDGE('',*,*,#9431,.T.);
#13218=ORIENTED_EDGE('',*,*,#9432,.F.);
#13219=ORIENTED_EDGE('',*,*,#9433,.F.);
#13220=ORIENTED_EDGE('',*,*,#9434,.T.);
#13221=ORIENTED_EDGE('',*,*,#9435,.F.);
#13222=ORIENTED_EDGE('',*,*,#9436,.F.);
#13223=ORIENTED_EDGE('',*,*,#9437,.T.);
#13224=ORIENTED_EDGE('',*,*,#9438,.F.);
#13225=ORIENTED_EDGE('',*,*,#9439,.F.);
#13226=ORIENTED_EDGE('',*,*,#9440,.T.);
#13227=ORIENTED_EDGE('',*,*,#9441,.F.);
#13228=ORIENTED_EDGE('',*,*,#9442,.F.);
#13229=ORIENTED_EDGE('',*,*,#9443,.T.);
#13230=ORIENTED_EDGE('',*,*,#9444,.F.);
#13231=ORIENTED_EDGE('',*,*,#9445,.F.);
#13232=ORIENTED_EDGE('',*,*,#9446,.T.);
#13233=ORIENTED_EDGE('',*,*,#9447,.F.);
#13234=ORIENTED_EDGE('',*,*,#9448,.F.);
#13235=ORIENTED_EDGE('',*,*,#9449,.T.);
#13236=ORIENTED_EDGE('',*,*,#9450,.F.);
#13237=ORIENTED_EDGE('',*,*,#9451,.F.);
#13238=ORIENTED_EDGE('',*,*,#9452,.T.);
#13239=ORIENTED_EDGE('',*,*,#9453,.F.);
#13240=ORIENTED_EDGE('',*,*,#9454,.F.);
#13241=ORIENTED_EDGE('',*,*,#9455,.T.);
#13242=ORIENTED_EDGE('',*,*,#9456,.F.);
#13243=ORIENTED_EDGE('',*,*,#9457,.F.);
#13244=ORIENTED_EDGE('',*,*,#9458,.T.);
#13245=ORIENTED_EDGE('',*,*,#9459,.F.);
#13246=ORIENTED_EDGE('',*,*,#9460,.F.);
#13247=ORIENTED_EDGE('',*,*,#9461,.T.);
#13248=ORIENTED_EDGE('',*,*,#9462,.F.);
#13249=ORIENTED_EDGE('',*,*,#9463,.F.);
#13250=ORIENTED_EDGE('',*,*,#9464,.T.);
#13251=ORIENTED_EDGE('',*,*,#9465,.F.);
#13252=ORIENTED_EDGE('',*,*,#9466,.F.);
#13253=ORIENTED_EDGE('',*,*,#9467,.T.);
#13254=ORIENTED_EDGE('',*,*,#9468,.F.);
#13255=ORIENTED_EDGE('',*,*,#9469,.F.);
#13256=ORIENTED_EDGE('',*,*,#9470,.T.);
#13257=ORIENTED_EDGE('',*,*,#9471,.F.);
#13258=ORIENTED_EDGE('',*,*,#9472,.F.);
#13259=ORIENTED_EDGE('',*,*,#9473,.T.);
#13260=ORIENTED_EDGE('',*,*,#9474,.F.);
#13261=ORIENTED_EDGE('',*,*,#9475,.F.);
#13262=ORIENTED_EDGE('',*,*,#9476,.T.);
#13263=ORIENTED_EDGE('',*,*,#9477,.F.);
#13264=ORIENTED_EDGE('',*,*,#9478,.F.);
#13265=ORIENTED_EDGE('',*,*,#9479,.T.);
#13266=ORIENTED_EDGE('',*,*,#9480,.F.);
#13267=ORIENTED_EDGE('',*,*,#9481,.T.);
#13268=ORIENTED_EDGE('',*,*,#9482,.F.);
#13269=ORIENTED_EDGE('',*,*,#9481,.F.);
#13270=ORIENTED_EDGE('',*,*,#9483,.F.);
#13271=ORIENTED_EDGE('',*,*,#9484,.F.);
#13272=ORIENTED_EDGE('',*,*,#9485,.T.);
#13273=ORIENTED_EDGE('',*,*,#9486,.F.);
#13274=ORIENTED_EDGE('',*,*,#9487,.F.);
#13275=ORIENTED_EDGE('',*,*,#9488,.T.);
#13276=ORIENTED_EDGE('',*,*,#9489,.F.);
#13277=ORIENTED_EDGE('',*,*,#9490,.F.);
#13278=ORIENTED_EDGE('',*,*,#9491,.T.);
#13279=ORIENTED_EDGE('',*,*,#9492,.F.);
#13280=ORIENTED_EDGE('',*,*,#9493,.F.);
#13281=ORIENTED_EDGE('',*,*,#9494,.T.);
#13282=ORIENTED_EDGE('',*,*,#9495,.F.);
#13283=ORIENTED_EDGE('',*,*,#9496,.F.);
#13284=ORIENTED_EDGE('',*,*,#9497,.T.);
#13285=ORIENTED_EDGE('',*,*,#9498,.F.);
#13286=ORIENTED_EDGE('',*,*,#9499,.F.);
#13287=ORIENTED_EDGE('',*,*,#9500,.T.);
#13288=ORIENTED_EDGE('',*,*,#9501,.F.);
#13289=ORIENTED_EDGE('',*,*,#9502,.F.);
#13290=ORIENTED_EDGE('',*,*,#9503,.T.);
#13291=ORIENTED_EDGE('',*,*,#9504,.F.);
#13292=ORIENTED_EDGE('',*,*,#9505,.F.);
#13293=ORIENTED_EDGE('',*,*,#9506,.T.);
#13294=ORIENTED_EDGE('',*,*,#9507,.F.);
#13295=ORIENTED_EDGE('',*,*,#9508,.F.);
#13296=ORIENTED_EDGE('',*,*,#9509,.T.);
#13297=ORIENTED_EDGE('',*,*,#9510,.F.);
#13298=ORIENTED_EDGE('',*,*,#9511,.F.);
#13299=ORIENTED_EDGE('',*,*,#9512,.T.);
#13300=ORIENTED_EDGE('',*,*,#9513,.F.);
#13301=ORIENTED_EDGE('',*,*,#9514,.F.);
#13302=ORIENTED_EDGE('',*,*,#9515,.T.);
#13303=ORIENTED_EDGE('',*,*,#9516,.F.);
#13304=ORIENTED_EDGE('',*,*,#9517,.F.);
#13305=ORIENTED_EDGE('',*,*,#9518,.T.);
#13306=ORIENTED_EDGE('',*,*,#9519,.F.);
#13307=ORIENTED_EDGE('',*,*,#9520,.F.);
#13308=ORIENTED_EDGE('',*,*,#9521,.T.);
#13309=ORIENTED_EDGE('',*,*,#9522,.F.);
#13310=ORIENTED_EDGE('',*,*,#9523,.F.);
#13311=ORIENTED_EDGE('',*,*,#9524,.T.);
#13312=ORIENTED_EDGE('',*,*,#9525,.F.);
#13313=ORIENTED_EDGE('',*,*,#9526,.F.);
#13314=ORIENTED_EDGE('',*,*,#9527,.T.);
#13315=ORIENTED_EDGE('',*,*,#9528,.F.);
#13316=ORIENTED_EDGE('',*,*,#9529,.F.);
#13317=ORIENTED_EDGE('',*,*,#9530,.T.);
#13318=ORIENTED_EDGE('',*,*,#9531,.F.);
#13319=ORIENTED_EDGE('',*,*,#9532,.F.);
#13320=ORIENTED_EDGE('',*,*,#9533,.T.);
#13321=ORIENTED_EDGE('',*,*,#9534,.F.);
#13322=ORIENTED_EDGE('',*,*,#9535,.F.);
#13323=ORIENTED_EDGE('',*,*,#9536,.T.);
#13324=ORIENTED_EDGE('',*,*,#9537,.F.);
#13325=ORIENTED_EDGE('',*,*,#9538,.F.);
#13326=ORIENTED_EDGE('',*,*,#9539,.T.);
#13327=ORIENTED_EDGE('',*,*,#9540,.F.);
#13328=ORIENTED_EDGE('',*,*,#9541,.F.);
#13329=ORIENTED_EDGE('',*,*,#9542,.T.);
#13330=ORIENTED_EDGE('',*,*,#9543,.F.);
#13331=ORIENTED_EDGE('',*,*,#9544,.F.);
#13332=ORIENTED_EDGE('',*,*,#9545,.T.);
#13333=ORIENTED_EDGE('',*,*,#9546,.F.);
#13334=ORIENTED_EDGE('',*,*,#9547,.F.);
#13335=ORIENTED_EDGE('',*,*,#9548,.T.);
#13336=ORIENTED_EDGE('',*,*,#9549,.F.);
#13337=ORIENTED_EDGE('',*,*,#9550,.F.);
#13338=ORIENTED_EDGE('',*,*,#9551,.T.);
#13339=ORIENTED_EDGE('',*,*,#9552,.F.);
#13340=ORIENTED_EDGE('',*,*,#9553,.F.);
#13341=ORIENTED_EDGE('',*,*,#9554,.T.);
#13342=ORIENTED_EDGE('',*,*,#9555,.F.);
#13343=ORIENTED_EDGE('',*,*,#9556,.F.);
#13344=ORIENTED_EDGE('',*,*,#9557,.T.);
#13345=ORIENTED_EDGE('',*,*,#9558,.F.);
#13346=ORIENTED_EDGE('',*,*,#9559,.F.);
#13347=ORIENTED_EDGE('',*,*,#9560,.T.);
#13348=ORIENTED_EDGE('',*,*,#9561,.F.);
#13349=ORIENTED_EDGE('',*,*,#9562,.F.);
#13350=ORIENTED_EDGE('',*,*,#9563,.T.);
#13351=ORIENTED_EDGE('',*,*,#9564,.F.);
#13352=ORIENTED_EDGE('',*,*,#9565,.F.);
#13353=ORIENTED_EDGE('',*,*,#9566,.T.);
#13354=ORIENTED_EDGE('',*,*,#9567,.F.);
#13355=ORIENTED_EDGE('',*,*,#9568,.F.);
#13356=ORIENTED_EDGE('',*,*,#9569,.T.);
#13357=ORIENTED_EDGE('',*,*,#9570,.F.);
#13358=ORIENTED_EDGE('',*,*,#9571,.F.);
#13359=ORIENTED_EDGE('',*,*,#9572,.T.);
#13360=ORIENTED_EDGE('',*,*,#9573,.F.);
#13361=ORIENTED_EDGE('',*,*,#9574,.F.);
#13362=ORIENTED_EDGE('',*,*,#9575,.T.);
#13363=ORIENTED_EDGE('',*,*,#9576,.F.);
#13364=ORIENTED_EDGE('',*,*,#9577,.F.);
#13365=ORIENTED_EDGE('',*,*,#9578,.T.);
#13366=ORIENTED_EDGE('',*,*,#9579,.F.);
#13367=ORIENTED_EDGE('',*,*,#9580,.F.);
#13368=ORIENTED_EDGE('',*,*,#9581,.T.);
#13369=ORIENTED_EDGE('',*,*,#9582,.F.);
#13370=ORIENTED_EDGE('',*,*,#9583,.F.);
#13371=ORIENTED_EDGE('',*,*,#9584,.T.);
#13372=ORIENTED_EDGE('',*,*,#9585,.F.);
#13373=ORIENTED_EDGE('',*,*,#9586,.F.);
#13374=ORIENTED_EDGE('',*,*,#9587,.T.);
#13375=ORIENTED_EDGE('',*,*,#9588,.F.);
#13376=ORIENTED_EDGE('',*,*,#9589,.F.);
#13377=ORIENTED_EDGE('',*,*,#9590,.T.);
#13378=ORIENTED_EDGE('',*,*,#9591,.F.);
#13379=ORIENTED_EDGE('',*,*,#9592,.F.);
#13380=ORIENTED_EDGE('',*,*,#9593,.T.);
#13381=ORIENTED_EDGE('',*,*,#9594,.F.);
#13382=ORIENTED_EDGE('',*,*,#9595,.F.);
#13383=ORIENTED_EDGE('',*,*,#9596,.T.);
#13384=ORIENTED_EDGE('',*,*,#9597,.F.);
#13385=ORIENTED_EDGE('',*,*,#9598,.T.);
#13386=ORIENTED_EDGE('',*,*,#9599,.F.);
#13387=ORIENTED_EDGE('',*,*,#9600,.T.);
#13388=ORIENTED_EDGE('',*,*,#9601,.T.);
#13389=ORIENTED_EDGE('',*,*,#9602,.F.);
#13390=ORIENTED_EDGE('',*,*,#9603,.T.);
#13391=ORIENTED_EDGE('',*,*,#9604,.T.);
#13392=ORIENTED_EDGE('',*,*,#9605,.F.);
#13393=ORIENTED_EDGE('',*,*,#9606,.T.);
#13394=ORIENTED_EDGE('',*,*,#9607,.T.);
#13395=ORIENTED_EDGE('',*,*,#9608,.F.);
#13396=ORIENTED_EDGE('',*,*,#9609,.T.);
#13397=ORIENTED_EDGE('',*,*,#9610,.T.);
#13398=ORIENTED_EDGE('',*,*,#9611,.F.);
#13399=ORIENTED_EDGE('',*,*,#9612,.T.);
#13400=ORIENTED_EDGE('',*,*,#9613,.T.);
#13401=ORIENTED_EDGE('',*,*,#9614,.F.);
#13402=ORIENTED_EDGE('',*,*,#9615,.T.);
#13403=ORIENTED_EDGE('',*,*,#9616,.T.);
#13404=ORIENTED_EDGE('',*,*,#9617,.F.);
#13405=ORIENTED_EDGE('',*,*,#9618,.T.);
#13406=ORIENTED_EDGE('',*,*,#9619,.T.);
#13407=ORIENTED_EDGE('',*,*,#9620,.F.);
#13408=ORIENTED_EDGE('',*,*,#9621,.T.);
#13409=ORIENTED_EDGE('',*,*,#9622,.T.);
#13410=ORIENTED_EDGE('',*,*,#9623,.F.);
#13411=ORIENTED_EDGE('',*,*,#9624,.T.);
#13412=ORIENTED_EDGE('',*,*,#9625,.T.);
#13413=ORIENTED_EDGE('',*,*,#9626,.F.);
#13414=ORIENTED_EDGE('',*,*,#9627,.T.);
#13415=ORIENTED_EDGE('',*,*,#9628,.T.);
#13416=ORIENTED_EDGE('',*,*,#9629,.F.);
#13417=ORIENTED_EDGE('',*,*,#9630,.T.);
#13418=ORIENTED_EDGE('',*,*,#9631,.T.);
#13419=ORIENTED_EDGE('',*,*,#9632,.F.);
#13420=ORIENTED_EDGE('',*,*,#9633,.T.);
#13421=ORIENTED_EDGE('',*,*,#9634,.T.);
#13422=ORIENTED_EDGE('',*,*,#9635,.F.);
#13423=ORIENTED_EDGE('',*,*,#9636,.T.);
#13424=ORIENTED_EDGE('',*,*,#9637,.T.);
#13425=ORIENTED_EDGE('',*,*,#9638,.F.);
#13426=ORIENTED_EDGE('',*,*,#9639,.T.);
#13427=ORIENTED_EDGE('',*,*,#9640,.T.);
#13428=ORIENTED_EDGE('',*,*,#9641,.F.);
#13429=ORIENTED_EDGE('',*,*,#9642,.T.);
#13430=ORIENTED_EDGE('',*,*,#9643,.T.);
#13431=ORIENTED_EDGE('',*,*,#9644,.F.);
#13432=ORIENTED_EDGE('',*,*,#9645,.T.);
#13433=ORIENTED_EDGE('',*,*,#9646,.T.);
#13434=ORIENTED_EDGE('',*,*,#9647,.F.);
#13435=ORIENTED_EDGE('',*,*,#9648,.T.);
#13436=ORIENTED_EDGE('',*,*,#9649,.T.);
#13437=ORIENTED_EDGE('',*,*,#9650,.F.);
#13438=ORIENTED_EDGE('',*,*,#9651,.T.);
#13439=ORIENTED_EDGE('',*,*,#9652,.T.);
#13440=ORIENTED_EDGE('',*,*,#9653,.F.);
#13441=ORIENTED_EDGE('',*,*,#9654,.T.);
#13442=ORIENTED_EDGE('',*,*,#9655,.T.);
#13443=ORIENTED_EDGE('',*,*,#9656,.F.);
#13444=ORIENTED_EDGE('',*,*,#9657,.T.);
#13445=ORIENTED_EDGE('',*,*,#9658,.T.);
#13446=ORIENTED_EDGE('',*,*,#9659,.F.);
#13447=ORIENTED_EDGE('',*,*,#9660,.T.);
#13448=ORIENTED_EDGE('',*,*,#9661,.T.);
#13449=ORIENTED_EDGE('',*,*,#9662,.F.);
#13450=ORIENTED_EDGE('',*,*,#9663,.T.);
#13451=ORIENTED_EDGE('',*,*,#9664,.T.);
#13452=ORIENTED_EDGE('',*,*,#9665,.F.);
#13453=ORIENTED_EDGE('',*,*,#9666,.T.);
#13454=ORIENTED_EDGE('',*,*,#9667,.T.);
#13455=ORIENTED_EDGE('',*,*,#9668,.F.);
#13456=ORIENTED_EDGE('',*,*,#9669,.T.);
#13457=ORIENTED_EDGE('',*,*,#9670,.T.);
#13458=ORIENTED_EDGE('',*,*,#9671,.F.);
#13459=ORIENTED_EDGE('',*,*,#9672,.T.);
#13460=ORIENTED_EDGE('',*,*,#9673,.T.);
#13461=ORIENTED_EDGE('',*,*,#9674,.F.);
#13462=ORIENTED_EDGE('',*,*,#9675,.T.);
#13463=ORIENTED_EDGE('',*,*,#9676,.T.);
#13464=ORIENTED_EDGE('',*,*,#9677,.F.);
#13465=ORIENTED_EDGE('',*,*,#9678,.T.);
#13466=ORIENTED_EDGE('',*,*,#9679,.T.);
#13467=ORIENTED_EDGE('',*,*,#9680,.F.);
#13468=ORIENTED_EDGE('',*,*,#9681,.T.);
#13469=ORIENTED_EDGE('',*,*,#9682,.T.);
#13470=ORIENTED_EDGE('',*,*,#9683,.F.);
#13471=ORIENTED_EDGE('',*,*,#9684,.T.);
#13472=ORIENTED_EDGE('',*,*,#9685,.T.);
#13473=ORIENTED_EDGE('',*,*,#9686,.F.);
#13474=ORIENTED_EDGE('',*,*,#9687,.T.);
#13475=ORIENTED_EDGE('',*,*,#9688,.T.);
#13476=ORIENTED_EDGE('',*,*,#9689,.F.);
#13477=ORIENTED_EDGE('',*,*,#9690,.T.);
#13478=ORIENTED_EDGE('',*,*,#9691,.T.);
#13479=ORIENTED_EDGE('',*,*,#9692,.F.);
#13480=ORIENTED_EDGE('',*,*,#9693,.T.);
#13481=ORIENTED_EDGE('',*,*,#9694,.T.);
#13482=ORIENTED_EDGE('',*,*,#9695,.F.);
#13483=ORIENTED_EDGE('',*,*,#9696,.T.);
#13484=ORIENTED_EDGE('',*,*,#9697,.T.);
#13485=ORIENTED_EDGE('',*,*,#9698,.F.);
#13486=ORIENTED_EDGE('',*,*,#9699,.T.);
#13487=ORIENTED_EDGE('',*,*,#9700,.T.);
#13488=ORIENTED_EDGE('',*,*,#9701,.F.);
#13489=ORIENTED_EDGE('',*,*,#9702,.T.);
#13490=ORIENTED_EDGE('',*,*,#9703,.T.);
#13491=ORIENTED_EDGE('',*,*,#9704,.F.);
#13492=ORIENTED_EDGE('',*,*,#9705,.T.);
#13493=ORIENTED_EDGE('',*,*,#9706,.T.);
#13494=ORIENTED_EDGE('',*,*,#9707,.F.);
#13495=ORIENTED_EDGE('',*,*,#9708,.T.);
#13496=ORIENTED_EDGE('',*,*,#9709,.T.);
#13497=ORIENTED_EDGE('',*,*,#9710,.F.);
#13498=ORIENTED_EDGE('',*,*,#9711,.T.);
#13499=ORIENTED_EDGE('',*,*,#9712,.T.);
#13500=ORIENTED_EDGE('',*,*,#9713,.F.);
#13501=ORIENTED_EDGE('',*,*,#9714,.T.);
#13502=ORIENTED_EDGE('',*,*,#9715,.T.);
#13503=ORIENTED_EDGE('',*,*,#9716,.T.);
#13504=ORIENTED_EDGE('',*,*,#9715,.F.);
#13505=ORIENTED_EDGE('',*,*,#9717,.T.);
#13506=ORIENTED_EDGE('',*,*,#9718,.T.);
#13507=ORIENTED_EDGE('',*,*,#9719,.F.);
#13508=ORIENTED_EDGE('',*,*,#9720,.T.);
#13509=ORIENTED_EDGE('',*,*,#9721,.T.);
#13510=ORIENTED_EDGE('',*,*,#9722,.F.);
#13511=ORIENTED_EDGE('',*,*,#9723,.T.);
#13512=ORIENTED_EDGE('',*,*,#9724,.T.);
#13513=ORIENTED_EDGE('',*,*,#9725,.F.);
#13514=ORIENTED_EDGE('',*,*,#9726,.T.);
#13515=ORIENTED_EDGE('',*,*,#9727,.T.);
#13516=ORIENTED_EDGE('',*,*,#9728,.F.);
#13517=ORIENTED_EDGE('',*,*,#9729,.T.);
#13518=ORIENTED_EDGE('',*,*,#9730,.T.);
#13519=ORIENTED_EDGE('',*,*,#9731,.F.);
#13520=ORIENTED_EDGE('',*,*,#9732,.T.);
#13521=ORIENTED_EDGE('',*,*,#9733,.T.);
#13522=ORIENTED_EDGE('',*,*,#9734,.F.);
#13523=ORIENTED_EDGE('',*,*,#9735,.T.);
#13524=ORIENTED_EDGE('',*,*,#9736,.T.);
#13525=ORIENTED_EDGE('',*,*,#9737,.F.);
#13526=ORIENTED_EDGE('',*,*,#9738,.T.);
#13527=ORIENTED_EDGE('',*,*,#9739,.T.);
#13528=ORIENTED_EDGE('',*,*,#9740,.F.);
#13529=ORIENTED_EDGE('',*,*,#9741,.T.);
#13530=ORIENTED_EDGE('',*,*,#9742,.T.);
#13531=ORIENTED_EDGE('',*,*,#9743,.F.);
#13532=ORIENTED_EDGE('',*,*,#9744,.T.);
#13533=ORIENTED_EDGE('',*,*,#9745,.T.);
#13534=ORIENTED_EDGE('',*,*,#9746,.F.);
#13535=ORIENTED_EDGE('',*,*,#9747,.T.);
#13536=ORIENTED_EDGE('',*,*,#9748,.T.);
#13537=ORIENTED_EDGE('',*,*,#9749,.F.);
#13538=ORIENTED_EDGE('',*,*,#9750,.T.);
#13539=ORIENTED_EDGE('',*,*,#9751,.T.);
#13540=ORIENTED_EDGE('',*,*,#9752,.F.);
#13541=ORIENTED_EDGE('',*,*,#9753,.T.);
#13542=ORIENTED_EDGE('',*,*,#9754,.T.);
#13543=ORIENTED_EDGE('',*,*,#9755,.F.);
#13544=ORIENTED_EDGE('',*,*,#9756,.T.);
#13545=ORIENTED_EDGE('',*,*,#9757,.T.);
#13546=ORIENTED_EDGE('',*,*,#9758,.F.);
#13547=ORIENTED_EDGE('',*,*,#9759,.T.);
#13548=ORIENTED_EDGE('',*,*,#9760,.T.);
#13549=ORIENTED_EDGE('',*,*,#9761,.F.);
#13550=ORIENTED_EDGE('',*,*,#9762,.T.);
#13551=ORIENTED_EDGE('',*,*,#9763,.T.);
#13552=ORIENTED_EDGE('',*,*,#9764,.F.);
#13553=ORIENTED_EDGE('',*,*,#9765,.T.);
#13554=ORIENTED_EDGE('',*,*,#9766,.T.);
#13555=ORIENTED_EDGE('',*,*,#9767,.F.);
#13556=ORIENTED_EDGE('',*,*,#9768,.T.);
#13557=ORIENTED_EDGE('',*,*,#9769,.T.);
#13558=ORIENTED_EDGE('',*,*,#9770,.F.);
#13559=ORIENTED_EDGE('',*,*,#9771,.T.);
#13560=ORIENTED_EDGE('',*,*,#9772,.T.);
#13561=ORIENTED_EDGE('',*,*,#9773,.F.);
#13562=ORIENTED_EDGE('',*,*,#9774,.T.);
#13563=ORIENTED_EDGE('',*,*,#9775,.T.);
#13564=ORIENTED_EDGE('',*,*,#9776,.F.);
#13565=ORIENTED_EDGE('',*,*,#9777,.T.);
#13566=ORIENTED_EDGE('',*,*,#9778,.T.);
#13567=ORIENTED_EDGE('',*,*,#9779,.F.);
#13568=ORIENTED_EDGE('',*,*,#9780,.T.);
#13569=ORIENTED_EDGE('',*,*,#9781,.T.);
#13570=ORIENTED_EDGE('',*,*,#9782,.F.);
#13571=ORIENTED_EDGE('',*,*,#9783,.T.);
#13572=ORIENTED_EDGE('',*,*,#9784,.T.);
#13573=ORIENTED_EDGE('',*,*,#9785,.F.);
#13574=ORIENTED_EDGE('',*,*,#9786,.T.);
#13575=ORIENTED_EDGE('',*,*,#9787,.T.);
#13576=ORIENTED_EDGE('',*,*,#9788,.F.);
#13577=ORIENTED_EDGE('',*,*,#9789,.T.);
#13578=ORIENTED_EDGE('',*,*,#9790,.T.);
#13579=ORIENTED_EDGE('',*,*,#9791,.F.);
#13580=ORIENTED_EDGE('',*,*,#9792,.T.);
#13581=ORIENTED_EDGE('',*,*,#9793,.T.);
#13582=ORIENTED_EDGE('',*,*,#9794,.F.);
#13583=ORIENTED_EDGE('',*,*,#9795,.T.);
#13584=ORIENTED_EDGE('',*,*,#9796,.T.);
#13585=ORIENTED_EDGE('',*,*,#9797,.F.);
#13586=ORIENTED_EDGE('',*,*,#9798,.T.);
#13587=ORIENTED_EDGE('',*,*,#9799,.T.);
#13588=ORIENTED_EDGE('',*,*,#9800,.F.);
#13589=ORIENTED_EDGE('',*,*,#9801,.T.);
#13590=ORIENTED_EDGE('',*,*,#9802,.T.);
#13591=ORIENTED_EDGE('',*,*,#9803,.F.);
#13592=ORIENTED_EDGE('',*,*,#9804,.T.);
#13593=ORIENTED_EDGE('',*,*,#9805,.T.);
#13594=ORIENTED_EDGE('',*,*,#9806,.F.);
#13595=ORIENTED_EDGE('',*,*,#9807,.T.);
#13596=ORIENTED_EDGE('',*,*,#9808,.T.);
#13597=ORIENTED_EDGE('',*,*,#9809,.F.);
#13598=ORIENTED_EDGE('',*,*,#9810,.T.);
#13599=ORIENTED_EDGE('',*,*,#9811,.T.);
#13600=ORIENTED_EDGE('',*,*,#9812,.F.);
#13601=ORIENTED_EDGE('',*,*,#9813,.T.);
#13602=ORIENTED_EDGE('',*,*,#9814,.T.);
#13603=ORIENTED_EDGE('',*,*,#9815,.F.);
#13604=ORIENTED_EDGE('',*,*,#9816,.T.);
#13605=ORIENTED_EDGE('',*,*,#9817,.T.);
#13606=ORIENTED_EDGE('',*,*,#9818,.F.);
#13607=ORIENTED_EDGE('',*,*,#9819,.T.);
#13608=ORIENTED_EDGE('',*,*,#9820,.T.);
#13609=ORIENTED_EDGE('',*,*,#9821,.F.);
#13610=ORIENTED_EDGE('',*,*,#9822,.T.);
#13611=ORIENTED_EDGE('',*,*,#9823,.T.);
#13612=ORIENTED_EDGE('',*,*,#9824,.F.);
#13613=ORIENTED_EDGE('',*,*,#9825,.T.);
#13614=ORIENTED_EDGE('',*,*,#9826,.T.);
#13615=ORIENTED_EDGE('',*,*,#9827,.F.);
#13616=ORIENTED_EDGE('',*,*,#9828,.T.);
#13617=ORIENTED_EDGE('',*,*,#9829,.T.);
#13618=ORIENTED_EDGE('',*,*,#9830,.F.);
#13619=ORIENTED_EDGE('',*,*,#9831,.T.);
#13620=ORIENTED_EDGE('',*,*,#9227,.T.);
#13621=ORIENTED_EDGE('',*,*,#9832,.T.);
#13622=ORIENTED_EDGE('',*,*,#9358,.T.);
#13623=ORIENTED_EDGE('',*,*,#9359,.T.);
#13624=ORIENTED_EDGE('',*,*,#9832,.F.);
#13625=ORIENTED_EDGE('',*,*,#9833,.F.);
#13626=ORIENTED_EDGE('',*,*,#9779,.T.);
#13627=ORIENTED_EDGE('',*,*,#9834,.T.);
#13628=ORIENTED_EDGE('',*,*,#9536,.F.);
#13629=ORIENTED_EDGE('',*,*,#9835,.T.);
#13630=ORIENTED_EDGE('',*,*,#9533,.F.);
#13631=ORIENTED_EDGE('',*,*,#9836,.F.);
#13632=ORIENTED_EDGE('',*,*,#9782,.T.);
#13633=ORIENTED_EDGE('',*,*,#9837,.T.);
#13634=ORIENTED_EDGE('',*,*,#9530,.F.);
#13635=ORIENTED_EDGE('',*,*,#9838,.F.);
#13636=ORIENTED_EDGE('',*,*,#9785,.T.);
#13637=ORIENTED_EDGE('',*,*,#9839,.T.);
#13638=ORIENTED_EDGE('',*,*,#9527,.F.);
#13639=ORIENTED_EDGE('',*,*,#9840,.F.);
#13640=ORIENTED_EDGE('',*,*,#9788,.T.);
#13641=ORIENTED_EDGE('',*,*,#9841,.T.);
#13642=ORIENTED_EDGE('',*,*,#9524,.F.);
#13643=ORIENTED_EDGE('',*,*,#9842,.F.);
#13644=ORIENTED_EDGE('',*,*,#9791,.T.);
#13645=ORIENTED_EDGE('',*,*,#9843,.T.);
#13646=ORIENTED_EDGE('',*,*,#9521,.F.);
#13647=ORIENTED_EDGE('',*,*,#9844,.F.);
#13648=ORIENTED_EDGE('',*,*,#9794,.T.);
#13649=ORIENTED_EDGE('',*,*,#9845,.T.);
#13650=ORIENTED_EDGE('',*,*,#9518,.F.);
#13651=ORIENTED_EDGE('',*,*,#9846,.F.);
#13652=ORIENTED_EDGE('',*,*,#9797,.T.);
#13653=ORIENTED_EDGE('',*,*,#9847,.T.);
#13654=ORIENTED_EDGE('',*,*,#9515,.F.);
#13655=ORIENTED_EDGE('',*,*,#9848,.F.);
#13656=ORIENTED_EDGE('',*,*,#9800,.T.);
#13657=ORIENTED_EDGE('',*,*,#9849,.T.);
#13658=ORIENTED_EDGE('',*,*,#9512,.F.);
#13659=ORIENTED_EDGE('',*,*,#9850,.F.);
#13660=ORIENTED_EDGE('',*,*,#9803,.T.);
#13661=ORIENTED_EDGE('',*,*,#9851,.T.);
#13662=ORIENTED_EDGE('',*,*,#9509,.F.);
#13663=ORIENTED_EDGE('',*,*,#9852,.F.);
#13664=ORIENTED_EDGE('',*,*,#9806,.T.);
#13665=ORIENTED_EDGE('',*,*,#9853,.T.);
#13666=ORIENTED_EDGE('',*,*,#9506,.F.);
#13667=ORIENTED_EDGE('',*,*,#9854,.F.);
#13668=ORIENTED_EDGE('',*,*,#9809,.T.);
#13669=ORIENTED_EDGE('',*,*,#9855,.T.);
#13670=ORIENTED_EDGE('',*,*,#9503,.F.);
#13671=ORIENTED_EDGE('',*,*,#9856,.F.);
#13672=ORIENTED_EDGE('',*,*,#9812,.T.);
#13673=ORIENTED_EDGE('',*,*,#9857,.T.);
#13674=ORIENTED_EDGE('',*,*,#9500,.F.);
#13675=ORIENTED_EDGE('',*,*,#9858,.F.);
#13676=ORIENTED_EDGE('',*,*,#9815,.T.);
#13677=ORIENTED_EDGE('',*,*,#9859,.T.);
#13678=ORIENTED_EDGE('',*,*,#9497,.F.);
#13679=ORIENTED_EDGE('',*,*,#9860,.F.);
#13680=ORIENTED_EDGE('',*,*,#9818,.T.);
#13681=ORIENTED_EDGE('',*,*,#9861,.T.);
#13682=ORIENTED_EDGE('',*,*,#9494,.F.);
#13683=ORIENTED_EDGE('',*,*,#9862,.F.);
#13684=ORIENTED_EDGE('',*,*,#9821,.T.);
#13685=ORIENTED_EDGE('',*,*,#9863,.T.);
#13686=ORIENTED_EDGE('',*,*,#9491,.F.);
#13687=ORIENTED_EDGE('',*,*,#9864,.F.);
#13688=ORIENTED_EDGE('',*,*,#9824,.T.);
#13689=ORIENTED_EDGE('',*,*,#9865,.T.);
#13690=ORIENTED_EDGE('',*,*,#9488,.F.);
#13691=ORIENTED_EDGE('',*,*,#9866,.F.);
#13692=ORIENTED_EDGE('',*,*,#9827,.T.);
#13693=ORIENTED_EDGE('',*,*,#9867,.T.);
#13694=ORIENTED_EDGE('',*,*,#9485,.F.);
#13695=ORIENTED_EDGE('',*,*,#9868,.F.);
#13696=ORIENTED_EDGE('',*,*,#9830,.T.);
#13697=ORIENTED_EDGE('',*,*,#9869,.T.);
#13698=ORIENTED_EDGE('',*,*,#9479,.F.);
#13699=ORIENTED_EDGE('',*,*,#9870,.F.);
#13700=ORIENTED_EDGE('',*,*,#9599,.T.);
#13701=ORIENTED_EDGE('',*,*,#9871,.T.);
#13702=ORIENTED_EDGE('',*,*,#9476,.F.);
#13703=ORIENTED_EDGE('',*,*,#9872,.F.);
#13704=ORIENTED_EDGE('',*,*,#9602,.T.);
#13705=ORIENTED_EDGE('',*,*,#9873,.T.);
#13706=ORIENTED_EDGE('',*,*,#9473,.F.);
#13707=ORIENTED_EDGE('',*,*,#9874,.F.);
#13708=ORIENTED_EDGE('',*,*,#9605,.T.);
#13709=ORIENTED_EDGE('',*,*,#9875,.T.);
#13710=ORIENTED_EDGE('',*,*,#9470,.F.);
#13711=ORIENTED_EDGE('',*,*,#9876,.F.);
#13712=ORIENTED_EDGE('',*,*,#9608,.T.);
#13713=ORIENTED_EDGE('',*,*,#9877,.T.);
#13714=ORIENTED_EDGE('',*,*,#9467,.F.);
#13715=ORIENTED_EDGE('',*,*,#9878,.F.);
#13716=ORIENTED_EDGE('',*,*,#9611,.T.);
#13717=ORIENTED_EDGE('',*,*,#9879,.T.);
#13718=ORIENTED_EDGE('',*,*,#9464,.F.);
#13719=ORIENTED_EDGE('',*,*,#9880,.F.);
#13720=ORIENTED_EDGE('',*,*,#9614,.T.);
#13721=ORIENTED_EDGE('',*,*,#9881,.T.);
#13722=ORIENTED_EDGE('',*,*,#9461,.F.);
#13723=ORIENTED_EDGE('',*,*,#9882,.F.);
#13724=ORIENTED_EDGE('',*,*,#9617,.T.);
#13725=ORIENTED_EDGE('',*,*,#9883,.T.);
#13726=ORIENTED_EDGE('',*,*,#9458,.F.);
#13727=ORIENTED_EDGE('',*,*,#9884,.F.);
#13728=ORIENTED_EDGE('',*,*,#9620,.T.);
#13729=ORIENTED_EDGE('',*,*,#9885,.T.);
#13730=ORIENTED_EDGE('',*,*,#9455,.F.);
#13731=ORIENTED_EDGE('',*,*,#9886,.F.);
#13732=ORIENTED_EDGE('',*,*,#9623,.T.);
#13733=ORIENTED_EDGE('',*,*,#9887,.T.);
#13734=ORIENTED_EDGE('',*,*,#9452,.F.);
#13735=ORIENTED_EDGE('',*,*,#9888,.F.);
#13736=ORIENTED_EDGE('',*,*,#9626,.T.);
#13737=ORIENTED_EDGE('',*,*,#9889,.T.);
#13738=ORIENTED_EDGE('',*,*,#9449,.F.);
#13739=ORIENTED_EDGE('',*,*,#9890,.F.);
#13740=ORIENTED_EDGE('',*,*,#9629,.T.);
#13741=ORIENTED_EDGE('',*,*,#9891,.T.);
#13742=ORIENTED_EDGE('',*,*,#9446,.F.);
#13743=ORIENTED_EDGE('',*,*,#9892,.F.);
#13744=ORIENTED_EDGE('',*,*,#9632,.T.);
#13745=ORIENTED_EDGE('',*,*,#9893,.T.);
#13746=ORIENTED_EDGE('',*,*,#9443,.F.);
#13747=ORIENTED_EDGE('',*,*,#9894,.F.);
#13748=ORIENTED_EDGE('',*,*,#9635,.T.);
#13749=ORIENTED_EDGE('',*,*,#9895,.T.);
#13750=ORIENTED_EDGE('',*,*,#9440,.F.);
#13751=ORIENTED_EDGE('',*,*,#9896,.F.);
#13752=ORIENTED_EDGE('',*,*,#9638,.T.);
#13753=ORIENTED_EDGE('',*,*,#9897,.T.);
#13754=ORIENTED_EDGE('',*,*,#9437,.F.);
#13755=ORIENTED_EDGE('',*,*,#9898,.F.);
#13756=ORIENTED_EDGE('',*,*,#9641,.T.);
#13757=ORIENTED_EDGE('',*,*,#9899,.T.);
#13758=ORIENTED_EDGE('',*,*,#9434,.F.);
#13759=ORIENTED_EDGE('',*,*,#9900,.F.);
#13760=ORIENTED_EDGE('',*,*,#9644,.T.);
#13761=ORIENTED_EDGE('',*,*,#9901,.T.);
#13762=ORIENTED_EDGE('',*,*,#9431,.F.);
#13763=ORIENTED_EDGE('',*,*,#9902,.F.);
#13764=ORIENTED_EDGE('',*,*,#9647,.T.);
#13765=ORIENTED_EDGE('',*,*,#9903,.T.);
#13766=ORIENTED_EDGE('',*,*,#9428,.F.);
#13767=ORIENTED_EDGE('',*,*,#9904,.F.);
#13768=ORIENTED_EDGE('',*,*,#9650,.T.);
#13769=ORIENTED_EDGE('',*,*,#9905,.T.);
#13770=ORIENTED_EDGE('',*,*,#9425,.F.);
#13771=ORIENTED_EDGE('',*,*,#9906,.F.);
#13772=ORIENTED_EDGE('',*,*,#9653,.T.);
#13773=ORIENTED_EDGE('',*,*,#9907,.T.);
#13774=ORIENTED_EDGE('',*,*,#9422,.F.);
#13775=ORIENTED_EDGE('',*,*,#9908,.F.);
#13776=ORIENTED_EDGE('',*,*,#9656,.T.);
#13777=ORIENTED_EDGE('',*,*,#9909,.T.);
#13778=ORIENTED_EDGE('',*,*,#9419,.F.);
#13779=ORIENTED_EDGE('',*,*,#9910,.F.);
#13780=ORIENTED_EDGE('',*,*,#9659,.T.);
#13781=ORIENTED_EDGE('',*,*,#9911,.T.);
#13782=ORIENTED_EDGE('',*,*,#9416,.F.);
#13783=ORIENTED_EDGE('',*,*,#9912,.F.);
#13784=ORIENTED_EDGE('',*,*,#9662,.T.);
#13785=ORIENTED_EDGE('',*,*,#9913,.T.);
#13786=ORIENTED_EDGE('',*,*,#9413,.F.);
#13787=ORIENTED_EDGE('',*,*,#9914,.F.);
#13788=ORIENTED_EDGE('',*,*,#9665,.T.);
#13789=ORIENTED_EDGE('',*,*,#9915,.T.);
#13790=ORIENTED_EDGE('',*,*,#9410,.F.);
#13791=ORIENTED_EDGE('',*,*,#9916,.F.);
#13792=ORIENTED_EDGE('',*,*,#9668,.T.);
#13793=ORIENTED_EDGE('',*,*,#9917,.T.);
#13794=ORIENTED_EDGE('',*,*,#9407,.F.);
#13795=ORIENTED_EDGE('',*,*,#9918,.F.);
#13796=ORIENTED_EDGE('',*,*,#9671,.T.);
#13797=ORIENTED_EDGE('',*,*,#9919,.T.);
#13798=ORIENTED_EDGE('',*,*,#9404,.F.);
#13799=ORIENTED_EDGE('',*,*,#9920,.F.);
#13800=ORIENTED_EDGE('',*,*,#9674,.T.);
#13801=ORIENTED_EDGE('',*,*,#9921,.T.);
#13802=ORIENTED_EDGE('',*,*,#9401,.F.);
#13803=ORIENTED_EDGE('',*,*,#9922,.F.);
#13804=ORIENTED_EDGE('',*,*,#9677,.T.);
#13805=ORIENTED_EDGE('',*,*,#9923,.T.);
#13806=ORIENTED_EDGE('',*,*,#9398,.F.);
#13807=ORIENTED_EDGE('',*,*,#9924,.F.);
#13808=ORIENTED_EDGE('',*,*,#9680,.T.);
#13809=ORIENTED_EDGE('',*,*,#9925,.T.);
#13810=ORIENTED_EDGE('',*,*,#9395,.F.);
#13811=ORIENTED_EDGE('',*,*,#9926,.F.);
#13812=ORIENTED_EDGE('',*,*,#9683,.T.);
#13813=ORIENTED_EDGE('',*,*,#9927,.T.);
#13814=ORIENTED_EDGE('',*,*,#9392,.F.);
#13815=ORIENTED_EDGE('',*,*,#9928,.F.);
#13816=ORIENTED_EDGE('',*,*,#9686,.T.);
#13817=ORIENTED_EDGE('',*,*,#9929,.T.);
#13818=ORIENTED_EDGE('',*,*,#9389,.F.);
#13819=ORIENTED_EDGE('',*,*,#9930,.F.);
#13820=ORIENTED_EDGE('',*,*,#9689,.T.);
#13821=ORIENTED_EDGE('',*,*,#9931,.T.);
#13822=ORIENTED_EDGE('',*,*,#9386,.F.);
#13823=ORIENTED_EDGE('',*,*,#9932,.F.);
#13824=ORIENTED_EDGE('',*,*,#9692,.T.);
#13825=ORIENTED_EDGE('',*,*,#9933,.T.);
#13826=ORIENTED_EDGE('',*,*,#9383,.F.);
#13827=ORIENTED_EDGE('',*,*,#9934,.F.);
#13828=ORIENTED_EDGE('',*,*,#9695,.T.);
#13829=ORIENTED_EDGE('',*,*,#9935,.T.);
#13830=ORIENTED_EDGE('',*,*,#9380,.F.);
#13831=ORIENTED_EDGE('',*,*,#9936,.F.);
#13832=ORIENTED_EDGE('',*,*,#9698,.T.);
#13833=ORIENTED_EDGE('',*,*,#9937,.T.);
#13834=ORIENTED_EDGE('',*,*,#9377,.F.);
#13835=ORIENTED_EDGE('',*,*,#9938,.F.);
#13836=ORIENTED_EDGE('',*,*,#9701,.T.);
#13837=ORIENTED_EDGE('',*,*,#9939,.T.);
#13838=ORIENTED_EDGE('',*,*,#9374,.F.);
#13839=ORIENTED_EDGE('',*,*,#9940,.F.);
#13840=ORIENTED_EDGE('',*,*,#9704,.T.);
#13841=ORIENTED_EDGE('',*,*,#9941,.T.);
#13842=ORIENTED_EDGE('',*,*,#9371,.F.);
#13843=ORIENTED_EDGE('',*,*,#9942,.F.);
#13844=ORIENTED_EDGE('',*,*,#9707,.T.);
#13845=ORIENTED_EDGE('',*,*,#9943,.T.);
#13846=ORIENTED_EDGE('',*,*,#9368,.F.);
#13847=ORIENTED_EDGE('',*,*,#9944,.F.);
#13848=ORIENTED_EDGE('',*,*,#9710,.T.);
#13849=ORIENTED_EDGE('',*,*,#9945,.T.);
#13850=ORIENTED_EDGE('',*,*,#9365,.F.);
#13851=ORIENTED_EDGE('',*,*,#9946,.F.);
#13852=ORIENTED_EDGE('',*,*,#9713,.T.);
#13853=ORIENTED_EDGE('',*,*,#9947,.T.);
#13854=ORIENTED_EDGE('',*,*,#9596,.F.);
#13855=ORIENTED_EDGE('',*,*,#9948,.F.);
#13856=ORIENTED_EDGE('',*,*,#9719,.T.);
#13857=ORIENTED_EDGE('',*,*,#9949,.T.);
#13858=ORIENTED_EDGE('',*,*,#9593,.F.);
#13859=ORIENTED_EDGE('',*,*,#9950,.F.);
#13860=ORIENTED_EDGE('',*,*,#9722,.T.);
#13861=ORIENTED_EDGE('',*,*,#9951,.T.);
#13862=ORIENTED_EDGE('',*,*,#9590,.F.);
#13863=ORIENTED_EDGE('',*,*,#9952,.F.);
#13864=ORIENTED_EDGE('',*,*,#9725,.T.);
#13865=ORIENTED_EDGE('',*,*,#9953,.T.);
#13866=ORIENTED_EDGE('',*,*,#9587,.F.);
#13867=ORIENTED_EDGE('',*,*,#9954,.F.);
#13868=ORIENTED_EDGE('',*,*,#9728,.T.);
#13869=ORIENTED_EDGE('',*,*,#9955,.T.);
#13870=ORIENTED_EDGE('',*,*,#9584,.F.);
#13871=ORIENTED_EDGE('',*,*,#9956,.F.);
#13872=ORIENTED_EDGE('',*,*,#9731,.T.);
#13873=ORIENTED_EDGE('',*,*,#9957,.T.);
#13874=ORIENTED_EDGE('',*,*,#9581,.F.);
#13875=ORIENTED_EDGE('',*,*,#9958,.F.);
#13876=ORIENTED_EDGE('',*,*,#9734,.T.);
#13877=ORIENTED_EDGE('',*,*,#9959,.T.);
#13878=ORIENTED_EDGE('',*,*,#9578,.F.);
#13879=ORIENTED_EDGE('',*,*,#9960,.F.);
#13880=ORIENTED_EDGE('',*,*,#9737,.T.);
#13881=ORIENTED_EDGE('',*,*,#9961,.T.);
#13882=ORIENTED_EDGE('',*,*,#9575,.F.);
#13883=ORIENTED_EDGE('',*,*,#9962,.F.);
#13884=ORIENTED_EDGE('',*,*,#9740,.T.);
#13885=ORIENTED_EDGE('',*,*,#9963,.T.);
#13886=ORIENTED_EDGE('',*,*,#9572,.F.);
#13887=ORIENTED_EDGE('',*,*,#9964,.F.);
#13888=ORIENTED_EDGE('',*,*,#9743,.T.);
#13889=ORIENTED_EDGE('',*,*,#9965,.T.);
#13890=ORIENTED_EDGE('',*,*,#9569,.F.);
#13891=ORIENTED_EDGE('',*,*,#9966,.F.);
#13892=ORIENTED_EDGE('',*,*,#9746,.T.);
#13893=ORIENTED_EDGE('',*,*,#9967,.T.);
#13894=ORIENTED_EDGE('',*,*,#9566,.F.);
#13895=ORIENTED_EDGE('',*,*,#9968,.F.);
#13896=ORIENTED_EDGE('',*,*,#9749,.T.);
#13897=ORIENTED_EDGE('',*,*,#9969,.T.);
#13898=ORIENTED_EDGE('',*,*,#9563,.F.);
#13899=ORIENTED_EDGE('',*,*,#9970,.F.);
#13900=ORIENTED_EDGE('',*,*,#9752,.T.);
#13901=ORIENTED_EDGE('',*,*,#9971,.T.);
#13902=ORIENTED_EDGE('',*,*,#9560,.F.);
#13903=ORIENTED_EDGE('',*,*,#9972,.F.);
#13904=ORIENTED_EDGE('',*,*,#9755,.T.);
#13905=ORIENTED_EDGE('',*,*,#9973,.T.);
#13906=ORIENTED_EDGE('',*,*,#9557,.F.);
#13907=ORIENTED_EDGE('',*,*,#9974,.F.);
#13908=ORIENTED_EDGE('',*,*,#9758,.T.);
#13909=ORIENTED_EDGE('',*,*,#9975,.T.);
#13910=ORIENTED_EDGE('',*,*,#9554,.F.);
#13911=ORIENTED_EDGE('',*,*,#9976,.F.);
#13912=ORIENTED_EDGE('',*,*,#9761,.T.);
#13913=ORIENTED_EDGE('',*,*,#9977,.T.);
#13914=ORIENTED_EDGE('',*,*,#9551,.F.);
#13915=ORIENTED_EDGE('',*,*,#9978,.F.);
#13916=ORIENTED_EDGE('',*,*,#9764,.T.);
#13917=ORIENTED_EDGE('',*,*,#9979,.T.);
#13918=ORIENTED_EDGE('',*,*,#9548,.F.);
#13919=ORIENTED_EDGE('',*,*,#9980,.F.);
#13920=ORIENTED_EDGE('',*,*,#9767,.T.);
#13921=ORIENTED_EDGE('',*,*,#9981,.T.);
#13922=ORIENTED_EDGE('',*,*,#9545,.F.);
#13923=ORIENTED_EDGE('',*,*,#9982,.F.);
#13924=ORIENTED_EDGE('',*,*,#9770,.T.);
#13925=ORIENTED_EDGE('',*,*,#9983,.F.);
#13926=ORIENTED_EDGE('',*,*,#9776,.T.);
#13927=ORIENTED_EDGE('',*,*,#9984,.T.);
#13928=ORIENTED_EDGE('',*,*,#9539,.F.);
#13929=ORIENTED_EDGE('',*,*,#9716,.F.);
#13930=ORIENTED_EDGE('',*,*,#9225,.T.);
#13931=ORIENTED_EDGE('',*,*,#9985,.T.);
#13932=ORIENTED_EDGE('',*,*,#9542,.F.);
#13933=ORIENTED_EDGE('',*,*,#9986,.F.);
#13934=ORIENTED_EDGE('',*,*,#9773,.T.);
#13935=ORIENTED_EDGE('',*,*,#9482,.T.);
#13936=ORIENTED_EDGE('',*,*,#9231,.F.);
#13937=ORIENTED_EDGE('',*,*,#9986,.T.);
#13938=ORIENTED_EDGE('',*,*,#9541,.T.);
#13939=ORIENTED_EDGE('',*,*,#9987,.F.);
#13940=ORIENTED_EDGE('',*,*,#9774,.F.);
#13941=ORIENTED_EDGE('',*,*,#9987,.T.);
#13942=ORIENTED_EDGE('',*,*,#9540,.T.);
#13943=ORIENTED_EDGE('',*,*,#9984,.F.);
#13944=ORIENTED_EDGE('',*,*,#9775,.F.);
#13945=ORIENTED_EDGE('',*,*,#9983,.T.);
#13946=ORIENTED_EDGE('',*,*,#9538,.T.);
#13947=ORIENTED_EDGE('',*,*,#9988,.F.);
#13948=ORIENTED_EDGE('',*,*,#9777,.F.);
#13949=ORIENTED_EDGE('',*,*,#9988,.T.);
#13950=ORIENTED_EDGE('',*,*,#9537,.T.);
#13951=ORIENTED_EDGE('',*,*,#9834,.F.);
#13952=ORIENTED_EDGE('',*,*,#9778,.F.);
#13953=ORIENTED_EDGE('',*,*,#9982,.T.);
#13954=ORIENTED_EDGE('',*,*,#9544,.T.);
#13955=ORIENTED_EDGE('',*,*,#9989,.F.);
#13956=ORIENTED_EDGE('',*,*,#9771,.F.);
#13957=ORIENTED_EDGE('',*,*,#9989,.T.);
#13958=ORIENTED_EDGE('',*,*,#9543,.T.);
#13959=ORIENTED_EDGE('',*,*,#9985,.F.);
#13960=ORIENTED_EDGE('',*,*,#9772,.F.);
#13961=ORIENTED_EDGE('',*,*,#9980,.T.);
#13962=ORIENTED_EDGE('',*,*,#9547,.T.);
#13963=ORIENTED_EDGE('',*,*,#9990,.F.);
#13964=ORIENTED_EDGE('',*,*,#9768,.F.);
#13965=ORIENTED_EDGE('',*,*,#9990,.T.);
#13966=ORIENTED_EDGE('',*,*,#9546,.T.);
#13967=ORIENTED_EDGE('',*,*,#9981,.F.);
#13968=ORIENTED_EDGE('',*,*,#9769,.F.);
#13969=ORIENTED_EDGE('',*,*,#9978,.T.);
#13970=ORIENTED_EDGE('',*,*,#9550,.T.);
#13971=ORIENTED_EDGE('',*,*,#9991,.F.);
#13972=ORIENTED_EDGE('',*,*,#9765,.F.);
#13973=ORIENTED_EDGE('',*,*,#9991,.T.);
#13974=ORIENTED_EDGE('',*,*,#9549,.T.);
#13975=ORIENTED_EDGE('',*,*,#9979,.F.);
#13976=ORIENTED_EDGE('',*,*,#9766,.F.);
#13977=ORIENTED_EDGE('',*,*,#9976,.T.);
#13978=ORIENTED_EDGE('',*,*,#9553,.T.);
#13979=ORIENTED_EDGE('',*,*,#9992,.F.);
#13980=ORIENTED_EDGE('',*,*,#9762,.F.);
#13981=ORIENTED_EDGE('',*,*,#9992,.T.);
#13982=ORIENTED_EDGE('',*,*,#9552,.T.);
#13983=ORIENTED_EDGE('',*,*,#9977,.F.);
#13984=ORIENTED_EDGE('',*,*,#9763,.F.);
#13985=ORIENTED_EDGE('',*,*,#9974,.T.);
#13986=ORIENTED_EDGE('',*,*,#9556,.T.);
#13987=ORIENTED_EDGE('',*,*,#9993,.F.);
#13988=ORIENTED_EDGE('',*,*,#9759,.F.);
#13989=ORIENTED_EDGE('',*,*,#9993,.T.);
#13990=ORIENTED_EDGE('',*,*,#9555,.T.);
#13991=ORIENTED_EDGE('',*,*,#9975,.F.);
#13992=ORIENTED_EDGE('',*,*,#9760,.F.);
#13993=ORIENTED_EDGE('',*,*,#9972,.T.);
#13994=ORIENTED_EDGE('',*,*,#9559,.T.);
#13995=ORIENTED_EDGE('',*,*,#9994,.F.);
#13996=ORIENTED_EDGE('',*,*,#9756,.F.);
#13997=ORIENTED_EDGE('',*,*,#9994,.T.);
#13998=ORIENTED_EDGE('',*,*,#9558,.T.);
#13999=ORIENTED_EDGE('',*,*,#9973,.F.);
#14000=ORIENTED_EDGE('',*,*,#9757,.F.);
#14001=ORIENTED_EDGE('',*,*,#9970,.T.);
#14002=ORIENTED_EDGE('',*,*,#9562,.T.);
#14003=ORIENTED_EDGE('',*,*,#9995,.F.);
#14004=ORIENTED_EDGE('',*,*,#9753,.F.);
#14005=ORIENTED_EDGE('',*,*,#9995,.T.);
#14006=ORIENTED_EDGE('',*,*,#9561,.T.);
#14007=ORIENTED_EDGE('',*,*,#9971,.F.);
#14008=ORIENTED_EDGE('',*,*,#9754,.F.);
#14009=ORIENTED_EDGE('',*,*,#9968,.T.);
#14010=ORIENTED_EDGE('',*,*,#9565,.T.);
#14011=ORIENTED_EDGE('',*,*,#9996,.F.);
#14012=ORIENTED_EDGE('',*,*,#9750,.F.);
#14013=ORIENTED_EDGE('',*,*,#9996,.T.);
#14014=ORIENTED_EDGE('',*,*,#9564,.T.);
#14015=ORIENTED_EDGE('',*,*,#9969,.F.);
#14016=ORIENTED_EDGE('',*,*,#9751,.F.);
#14017=ORIENTED_EDGE('',*,*,#9966,.T.);
#14018=ORIENTED_EDGE('',*,*,#9568,.T.);
#14019=ORIENTED_EDGE('',*,*,#9997,.F.);
#14020=ORIENTED_EDGE('',*,*,#9747,.F.);
#14021=ORIENTED_EDGE('',*,*,#9997,.T.);
#14022=ORIENTED_EDGE('',*,*,#9567,.T.);
#14023=ORIENTED_EDGE('',*,*,#9967,.F.);
#14024=ORIENTED_EDGE('',*,*,#9748,.F.);
#14025=ORIENTED_EDGE('',*,*,#9964,.T.);
#14026=ORIENTED_EDGE('',*,*,#9571,.T.);
#14027=ORIENTED_EDGE('',*,*,#9998,.F.);
#14028=ORIENTED_EDGE('',*,*,#9744,.F.);
#14029=ORIENTED_EDGE('',*,*,#9998,.T.);
#14030=ORIENTED_EDGE('',*,*,#9570,.T.);
#14031=ORIENTED_EDGE('',*,*,#9965,.F.);
#14032=ORIENTED_EDGE('',*,*,#9745,.F.);
#14033=ORIENTED_EDGE('',*,*,#9962,.T.);
#14034=ORIENTED_EDGE('',*,*,#9574,.T.);
#14035=ORIENTED_EDGE('',*,*,#9999,.F.);
#14036=ORIENTED_EDGE('',*,*,#9741,.F.);
#14037=ORIENTED_EDGE('',*,*,#9999,.T.);
#14038=ORIENTED_EDGE('',*,*,#9573,.T.);
#14039=ORIENTED_EDGE('',*,*,#9963,.F.);
#14040=ORIENTED_EDGE('',*,*,#9742,.F.);
#14041=ORIENTED_EDGE('',*,*,#9960,.T.);
#14042=ORIENTED_EDGE('',*,*,#9577,.T.);
#14043=ORIENTED_EDGE('',*,*,#10000,.F.);
#14044=ORIENTED_EDGE('',*,*,#9738,.F.);
#14045=ORIENTED_EDGE('',*,*,#10000,.T.);
#14046=ORIENTED_EDGE('',*,*,#9576,.T.);
#14047=ORIENTED_EDGE('',*,*,#9961,.F.);
#14048=ORIENTED_EDGE('',*,*,#9739,.F.);
#14049=ORIENTED_EDGE('',*,*,#9958,.T.);
#14050=ORIENTED_EDGE('',*,*,#9580,.T.);
#14051=ORIENTED_EDGE('',*,*,#10001,.F.);
#14052=ORIENTED_EDGE('',*,*,#9735,.F.);
#14053=ORIENTED_EDGE('',*,*,#10001,.T.);
#14054=ORIENTED_EDGE('',*,*,#9579,.T.);
#14055=ORIENTED_EDGE('',*,*,#9959,.F.);
#14056=ORIENTED_EDGE('',*,*,#9736,.F.);
#14057=ORIENTED_EDGE('',*,*,#9956,.T.);
#14058=ORIENTED_EDGE('',*,*,#9583,.T.);
#14059=ORIENTED_EDGE('',*,*,#10002,.F.);
#14060=ORIENTED_EDGE('',*,*,#9732,.F.);
#14061=ORIENTED_EDGE('',*,*,#10002,.T.);
#14062=ORIENTED_EDGE('',*,*,#9582,.T.);
#14063=ORIENTED_EDGE('',*,*,#9957,.F.);
#14064=ORIENTED_EDGE('',*,*,#9733,.F.);
#14065=ORIENTED_EDGE('',*,*,#9954,.T.);
#14066=ORIENTED_EDGE('',*,*,#9586,.T.);
#14067=ORIENTED_EDGE('',*,*,#10003,.F.);
#14068=ORIENTED_EDGE('',*,*,#9729,.F.);
#14069=ORIENTED_EDGE('',*,*,#10003,.T.);
#14070=ORIENTED_EDGE('',*,*,#9585,.T.);
#14071=ORIENTED_EDGE('',*,*,#9955,.F.);
#14072=ORIENTED_EDGE('',*,*,#9730,.F.);
#14073=ORIENTED_EDGE('',*,*,#9952,.T.);
#14074=ORIENTED_EDGE('',*,*,#9589,.T.);
#14075=ORIENTED_EDGE('',*,*,#10004,.F.);
#14076=ORIENTED_EDGE('',*,*,#9726,.F.);
#14077=ORIENTED_EDGE('',*,*,#10004,.T.);
#14078=ORIENTED_EDGE('',*,*,#9588,.T.);
#14079=ORIENTED_EDGE('',*,*,#9953,.F.);
#14080=ORIENTED_EDGE('',*,*,#9727,.F.);
#14081=ORIENTED_EDGE('',*,*,#9950,.T.);
#14082=ORIENTED_EDGE('',*,*,#9592,.T.);
#14083=ORIENTED_EDGE('',*,*,#10005,.F.);
#14084=ORIENTED_EDGE('',*,*,#9723,.F.);
#14085=ORIENTED_EDGE('',*,*,#10005,.T.);
#14086=ORIENTED_EDGE('',*,*,#9591,.T.);
#14087=ORIENTED_EDGE('',*,*,#9951,.F.);
#14088=ORIENTED_EDGE('',*,*,#9724,.F.);
#14089=ORIENTED_EDGE('',*,*,#9948,.T.);
#14090=ORIENTED_EDGE('',*,*,#9595,.T.);
#14091=ORIENTED_EDGE('',*,*,#10006,.F.);
#14092=ORIENTED_EDGE('',*,*,#9720,.F.);
#14093=ORIENTED_EDGE('',*,*,#10006,.T.);
#14094=ORIENTED_EDGE('',*,*,#9594,.T.);
#14095=ORIENTED_EDGE('',*,*,#9949,.F.);
#14096=ORIENTED_EDGE('',*,*,#9721,.F.);
#14097=ORIENTED_EDGE('',*,*,#9946,.T.);
#14098=ORIENTED_EDGE('',*,*,#9364,.T.);
#14099=ORIENTED_EDGE('',*,*,#10007,.F.);
#14100=ORIENTED_EDGE('',*,*,#9717,.F.);
#14101=ORIENTED_EDGE('',*,*,#9714,.F.);
#14102=ORIENTED_EDGE('',*,*,#10007,.T.);
#14103=ORIENTED_EDGE('',*,*,#9597,.T.);
#14104=ORIENTED_EDGE('',*,*,#9947,.F.);
#14105=ORIENTED_EDGE('',*,*,#9718,.F.);
#14106=ORIENTED_EDGE('',*,*,#9944,.T.);
#14107=ORIENTED_EDGE('',*,*,#9367,.T.);
#14108=ORIENTED_EDGE('',*,*,#10008,.F.);
#14109=ORIENTED_EDGE('',*,*,#9711,.F.);
#14110=ORIENTED_EDGE('',*,*,#10008,.T.);
#14111=ORIENTED_EDGE('',*,*,#9366,.T.);
#14112=ORIENTED_EDGE('',*,*,#9945,.F.);
#14113=ORIENTED_EDGE('',*,*,#9712,.F.);
#14114=ORIENTED_EDGE('',*,*,#9942,.T.);
#14115=ORIENTED_EDGE('',*,*,#9370,.T.);
#14116=ORIENTED_EDGE('',*,*,#10009,.F.);
#14117=ORIENTED_EDGE('',*,*,#9708,.F.);
#14118=ORIENTED_EDGE('',*,*,#10009,.T.);
#14119=ORIENTED_EDGE('',*,*,#9369,.T.);
#14120=ORIENTED_EDGE('',*,*,#9943,.F.);
#14121=ORIENTED_EDGE('',*,*,#9709,.F.);
#14122=ORIENTED_EDGE('',*,*,#9940,.T.);
#14123=ORIENTED_EDGE('',*,*,#9373,.T.);
#14124=ORIENTED_EDGE('',*,*,#10010,.F.);
#14125=ORIENTED_EDGE('',*,*,#9705,.F.);
#14126=ORIENTED_EDGE('',*,*,#10010,.T.);
#14127=ORIENTED_EDGE('',*,*,#9372,.T.);
#14128=ORIENTED_EDGE('',*,*,#9941,.F.);
#14129=ORIENTED_EDGE('',*,*,#9706,.F.);
#14130=ORIENTED_EDGE('',*,*,#9938,.T.);
#14131=ORIENTED_EDGE('',*,*,#9376,.T.);
#14132=ORIENTED_EDGE('',*,*,#10011,.F.);
#14133=ORIENTED_EDGE('',*,*,#9702,.F.);
#14134=ORIENTED_EDGE('',*,*,#10011,.T.);
#14135=ORIENTED_EDGE('',*,*,#9375,.T.);
#14136=ORIENTED_EDGE('',*,*,#9939,.F.);
#14137=ORIENTED_EDGE('',*,*,#9703,.F.);
#14138=ORIENTED_EDGE('',*,*,#9936,.T.);
#14139=ORIENTED_EDGE('',*,*,#9379,.T.);
#14140=ORIENTED_EDGE('',*,*,#10012,.F.);
#14141=ORIENTED_EDGE('',*,*,#9699,.F.);
#14142=ORIENTED_EDGE('',*,*,#10012,.T.);
#14143=ORIENTED_EDGE('',*,*,#9378,.T.);
#14144=ORIENTED_EDGE('',*,*,#9937,.F.);
#14145=ORIENTED_EDGE('',*,*,#9700,.F.);
#14146=ORIENTED_EDGE('',*,*,#9934,.T.);
#14147=ORIENTED_EDGE('',*,*,#9382,.T.);
#14148=ORIENTED_EDGE('',*,*,#10013,.F.);
#14149=ORIENTED_EDGE('',*,*,#9696,.F.);
#14150=ORIENTED_EDGE('',*,*,#10013,.T.);
#14151=ORIENTED_EDGE('',*,*,#9381,.T.);
#14152=ORIENTED_EDGE('',*,*,#9935,.F.);
#14153=ORIENTED_EDGE('',*,*,#9697,.F.);
#14154=ORIENTED_EDGE('',*,*,#9932,.T.);
#14155=ORIENTED_EDGE('',*,*,#9385,.T.);
#14156=ORIENTED_EDGE('',*,*,#10014,.F.);
#14157=ORIENTED_EDGE('',*,*,#9693,.F.);
#14158=ORIENTED_EDGE('',*,*,#10014,.T.);
#14159=ORIENTED_EDGE('',*,*,#9384,.T.);
#14160=ORIENTED_EDGE('',*,*,#9933,.F.);
#14161=ORIENTED_EDGE('',*,*,#9694,.F.);
#14162=ORIENTED_EDGE('',*,*,#9930,.T.);
#14163=ORIENTED_EDGE('',*,*,#9388,.T.);
#14164=ORIENTED_EDGE('',*,*,#10015,.F.);
#14165=ORIENTED_EDGE('',*,*,#9690,.F.);
#14166=ORIENTED_EDGE('',*,*,#10015,.T.);
#14167=ORIENTED_EDGE('',*,*,#9387,.T.);
#14168=ORIENTED_EDGE('',*,*,#9931,.F.);
#14169=ORIENTED_EDGE('',*,*,#9691,.F.);
#14170=ORIENTED_EDGE('',*,*,#9928,.T.);
#14171=ORIENTED_EDGE('',*,*,#9391,.T.);
#14172=ORIENTED_EDGE('',*,*,#10016,.F.);
#14173=ORIENTED_EDGE('',*,*,#9687,.F.);
#14174=ORIENTED_EDGE('',*,*,#10016,.T.);
#14175=ORIENTED_EDGE('',*,*,#9390,.T.);
#14176=ORIENTED_EDGE('',*,*,#9929,.F.);
#14177=ORIENTED_EDGE('',*,*,#9688,.F.);
#14178=ORIENTED_EDGE('',*,*,#9926,.T.);
#14179=ORIENTED_EDGE('',*,*,#9394,.T.);
#14180=ORIENTED_EDGE('',*,*,#10017,.F.);
#14181=ORIENTED_EDGE('',*,*,#9684,.F.);
#14182=ORIENTED_EDGE('',*,*,#10017,.T.);
#14183=ORIENTED_EDGE('',*,*,#9393,.T.);
#14184=ORIENTED_EDGE('',*,*,#9927,.F.);
#14185=ORIENTED_EDGE('',*,*,#9685,.F.);
#14186=ORIENTED_EDGE('',*,*,#9924,.T.);
#14187=ORIENTED_EDGE('',*,*,#9397,.T.);
#14188=ORIENTED_EDGE('',*,*,#10018,.F.);
#14189=ORIENTED_EDGE('',*,*,#9681,.F.);
#14190=ORIENTED_EDGE('',*,*,#10018,.T.);
#14191=ORIENTED_EDGE('',*,*,#9396,.T.);
#14192=ORIENTED_EDGE('',*,*,#9925,.F.);
#14193=ORIENTED_EDGE('',*,*,#9682,.F.);
#14194=ORIENTED_EDGE('',*,*,#9922,.T.);
#14195=ORIENTED_EDGE('',*,*,#9400,.T.);
#14196=ORIENTED_EDGE('',*,*,#10019,.F.);
#14197=ORIENTED_EDGE('',*,*,#9678,.F.);
#14198=ORIENTED_EDGE('',*,*,#10019,.T.);
#14199=ORIENTED_EDGE('',*,*,#9399,.T.);
#14200=ORIENTED_EDGE('',*,*,#9923,.F.);
#14201=ORIENTED_EDGE('',*,*,#9679,.F.);
#14202=ORIENTED_EDGE('',*,*,#9920,.T.);
#14203=ORIENTED_EDGE('',*,*,#9403,.T.);
#14204=ORIENTED_EDGE('',*,*,#10020,.F.);
#14205=ORIENTED_EDGE('',*,*,#9675,.F.);
#14206=ORIENTED_EDGE('',*,*,#10020,.T.);
#14207=ORIENTED_EDGE('',*,*,#9402,.T.);
#14208=ORIENTED_EDGE('',*,*,#9921,.F.);
#14209=ORIENTED_EDGE('',*,*,#9676,.F.);
#14210=ORIENTED_EDGE('',*,*,#9918,.T.);
#14211=ORIENTED_EDGE('',*,*,#9406,.T.);
#14212=ORIENTED_EDGE('',*,*,#10021,.F.);
#14213=ORIENTED_EDGE('',*,*,#9672,.F.);
#14214=ORIENTED_EDGE('',*,*,#10021,.T.);
#14215=ORIENTED_EDGE('',*,*,#9405,.T.);
#14216=ORIENTED_EDGE('',*,*,#9919,.F.);
#14217=ORIENTED_EDGE('',*,*,#9673,.F.);
#14218=ORIENTED_EDGE('',*,*,#9916,.T.);
#14219=ORIENTED_EDGE('',*,*,#9409,.T.);
#14220=ORIENTED_EDGE('',*,*,#10022,.F.);
#14221=ORIENTED_EDGE('',*,*,#9669,.F.);
#14222=ORIENTED_EDGE('',*,*,#10022,.T.);
#14223=ORIENTED_EDGE('',*,*,#9408,.T.);
#14224=ORIENTED_EDGE('',*,*,#9917,.F.);
#14225=ORIENTED_EDGE('',*,*,#9670,.F.);
#14226=ORIENTED_EDGE('',*,*,#9914,.T.);
#14227=ORIENTED_EDGE('',*,*,#9412,.T.);
#14228=ORIENTED_EDGE('',*,*,#10023,.F.);
#14229=ORIENTED_EDGE('',*,*,#9666,.F.);
#14230=ORIENTED_EDGE('',*,*,#10023,.T.);
#14231=ORIENTED_EDGE('',*,*,#9411,.T.);
#14232=ORIENTED_EDGE('',*,*,#9915,.F.);
#14233=ORIENTED_EDGE('',*,*,#9667,.F.);
#14234=ORIENTED_EDGE('',*,*,#9912,.T.);
#14235=ORIENTED_EDGE('',*,*,#9415,.T.);
#14236=ORIENTED_EDGE('',*,*,#10024,.F.);
#14237=ORIENTED_EDGE('',*,*,#9663,.F.);
#14238=ORIENTED_EDGE('',*,*,#10024,.T.);
#14239=ORIENTED_EDGE('',*,*,#9414,.T.);
#14240=ORIENTED_EDGE('',*,*,#9913,.F.);
#14241=ORIENTED_EDGE('',*,*,#9664,.F.);
#14242=ORIENTED_EDGE('',*,*,#9910,.T.);
#14243=ORIENTED_EDGE('',*,*,#9418,.T.);
#14244=ORIENTED_EDGE('',*,*,#10025,.F.);
#14245=ORIENTED_EDGE('',*,*,#9660,.F.);
#14246=ORIENTED_EDGE('',*,*,#10025,.T.);
#14247=ORIENTED_EDGE('',*,*,#9417,.T.);
#14248=ORIENTED_EDGE('',*,*,#9911,.F.);
#14249=ORIENTED_EDGE('',*,*,#9661,.F.);
#14250=ORIENTED_EDGE('',*,*,#9908,.T.);
#14251=ORIENTED_EDGE('',*,*,#9421,.T.);
#14252=ORIENTED_EDGE('',*,*,#10026,.F.);
#14253=ORIENTED_EDGE('',*,*,#9657,.F.);
#14254=ORIENTED_EDGE('',*,*,#10026,.T.);
#14255=ORIENTED_EDGE('',*,*,#9420,.T.);
#14256=ORIENTED_EDGE('',*,*,#9909,.F.);
#14257=ORIENTED_EDGE('',*,*,#9658,.F.);
#14258=ORIENTED_EDGE('',*,*,#9906,.T.);
#14259=ORIENTED_EDGE('',*,*,#9424,.T.);
#14260=ORIENTED_EDGE('',*,*,#10027,.F.);
#14261=ORIENTED_EDGE('',*,*,#9654,.F.);
#14262=ORIENTED_EDGE('',*,*,#10027,.T.);
#14263=ORIENTED_EDGE('',*,*,#9423,.T.);
#14264=ORIENTED_EDGE('',*,*,#9907,.F.);
#14265=ORIENTED_EDGE('',*,*,#9655,.F.);
#14266=ORIENTED_EDGE('',*,*,#9904,.T.);
#14267=ORIENTED_EDGE('',*,*,#9427,.T.);
#14268=ORIENTED_EDGE('',*,*,#10028,.F.);
#14269=ORIENTED_EDGE('',*,*,#9651,.F.);
#14270=ORIENTED_EDGE('',*,*,#10028,.T.);
#14271=ORIENTED_EDGE('',*,*,#9426,.T.);
#14272=ORIENTED_EDGE('',*,*,#9905,.F.);
#14273=ORIENTED_EDGE('',*,*,#9652,.F.);
#14274=ORIENTED_EDGE('',*,*,#9902,.T.);
#14275=ORIENTED_EDGE('',*,*,#9430,.T.);
#14276=ORIENTED_EDGE('',*,*,#10029,.F.);
#14277=ORIENTED_EDGE('',*,*,#9648,.F.);
#14278=ORIENTED_EDGE('',*,*,#10029,.T.);
#14279=ORIENTED_EDGE('',*,*,#9429,.T.);
#14280=ORIENTED_EDGE('',*,*,#9903,.F.);
#14281=ORIENTED_EDGE('',*,*,#9649,.F.);
#14282=ORIENTED_EDGE('',*,*,#9900,.T.);
#14283=ORIENTED_EDGE('',*,*,#9433,.T.);
#14284=ORIENTED_EDGE('',*,*,#10030,.F.);
#14285=ORIENTED_EDGE('',*,*,#9645,.F.);
#14286=ORIENTED_EDGE('',*,*,#10030,.T.);
#14287=ORIENTED_EDGE('',*,*,#9432,.T.);
#14288=ORIENTED_EDGE('',*,*,#9901,.F.);
#14289=ORIENTED_EDGE('',*,*,#9646,.F.);
#14290=ORIENTED_EDGE('',*,*,#9898,.T.);
#14291=ORIENTED_EDGE('',*,*,#9436,.T.);
#14292=ORIENTED_EDGE('',*,*,#10031,.F.);
#14293=ORIENTED_EDGE('',*,*,#9642,.F.);
#14294=ORIENTED_EDGE('',*,*,#10031,.T.);
#14295=ORIENTED_EDGE('',*,*,#9435,.T.);
#14296=ORIENTED_EDGE('',*,*,#9899,.F.);
#14297=ORIENTED_EDGE('',*,*,#9643,.F.);
#14298=ORIENTED_EDGE('',*,*,#9896,.T.);
#14299=ORIENTED_EDGE('',*,*,#9439,.T.);
#14300=ORIENTED_EDGE('',*,*,#10032,.F.);
#14301=ORIENTED_EDGE('',*,*,#9639,.F.);
#14302=ORIENTED_EDGE('',*,*,#10032,.T.);
#14303=ORIENTED_EDGE('',*,*,#9438,.T.);
#14304=ORIENTED_EDGE('',*,*,#9897,.F.);
#14305=ORIENTED_EDGE('',*,*,#9640,.F.);
#14306=ORIENTED_EDGE('',*,*,#9894,.T.);
#14307=ORIENTED_EDGE('',*,*,#9442,.T.);
#14308=ORIENTED_EDGE('',*,*,#10033,.F.);
#14309=ORIENTED_EDGE('',*,*,#9636,.F.);
#14310=ORIENTED_EDGE('',*,*,#10033,.T.);
#14311=ORIENTED_EDGE('',*,*,#9441,.T.);
#14312=ORIENTED_EDGE('',*,*,#9895,.F.);
#14313=ORIENTED_EDGE('',*,*,#9637,.F.);
#14314=ORIENTED_EDGE('',*,*,#9892,.T.);
#14315=ORIENTED_EDGE('',*,*,#9445,.T.);
#14316=ORIENTED_EDGE('',*,*,#10034,.F.);
#14317=ORIENTED_EDGE('',*,*,#9633,.F.);
#14318=ORIENTED_EDGE('',*,*,#10034,.T.);
#14319=ORIENTED_EDGE('',*,*,#9444,.T.);
#14320=ORIENTED_EDGE('',*,*,#9893,.F.);
#14321=ORIENTED_EDGE('',*,*,#9634,.F.);
#14322=ORIENTED_EDGE('',*,*,#9890,.T.);
#14323=ORIENTED_EDGE('',*,*,#9448,.T.);
#14324=ORIENTED_EDGE('',*,*,#10035,.F.);
#14325=ORIENTED_EDGE('',*,*,#9630,.F.);
#14326=ORIENTED_EDGE('',*,*,#10035,.T.);
#14327=ORIENTED_EDGE('',*,*,#9447,.T.);
#14328=ORIENTED_EDGE('',*,*,#9891,.F.);
#14329=ORIENTED_EDGE('',*,*,#9631,.F.);
#14330=ORIENTED_EDGE('',*,*,#9888,.T.);
#14331=ORIENTED_EDGE('',*,*,#9451,.T.);
#14332=ORIENTED_EDGE('',*,*,#10036,.F.);
#14333=ORIENTED_EDGE('',*,*,#9627,.F.);
#14334=ORIENTED_EDGE('',*,*,#10036,.T.);
#14335=ORIENTED_EDGE('',*,*,#9450,.T.);
#14336=ORIENTED_EDGE('',*,*,#9889,.F.);
#14337=ORIENTED_EDGE('',*,*,#9628,.F.);
#14338=ORIENTED_EDGE('',*,*,#9886,.T.);
#14339=ORIENTED_EDGE('',*,*,#9454,.T.);
#14340=ORIENTED_EDGE('',*,*,#10037,.F.);
#14341=ORIENTED_EDGE('',*,*,#9624,.F.);
#14342=ORIENTED_EDGE('',*,*,#10037,.T.);
#14343=ORIENTED_EDGE('',*,*,#9453,.T.);
#14344=ORIENTED_EDGE('',*,*,#9887,.F.);
#14345=ORIENTED_EDGE('',*,*,#9625,.F.);
#14346=ORIENTED_EDGE('',*,*,#9884,.T.);
#14347=ORIENTED_EDGE('',*,*,#9457,.T.);
#14348=ORIENTED_EDGE('',*,*,#10038,.F.);
#14349=ORIENTED_EDGE('',*,*,#9621,.F.);
#14350=ORIENTED_EDGE('',*,*,#10038,.T.);
#14351=ORIENTED_EDGE('',*,*,#9456,.T.);
#14352=ORIENTED_EDGE('',*,*,#9885,.F.);
#14353=ORIENTED_EDGE('',*,*,#9622,.F.);
#14354=ORIENTED_EDGE('',*,*,#9882,.T.);
#14355=ORIENTED_EDGE('',*,*,#9460,.T.);
#14356=ORIENTED_EDGE('',*,*,#10039,.F.);
#14357=ORIENTED_EDGE('',*,*,#9618,.F.);
#14358=ORIENTED_EDGE('',*,*,#10039,.T.);
#14359=ORIENTED_EDGE('',*,*,#9459,.T.);
#14360=ORIENTED_EDGE('',*,*,#9883,.F.);
#14361=ORIENTED_EDGE('',*,*,#9619,.F.);
#14362=ORIENTED_EDGE('',*,*,#9880,.T.);
#14363=ORIENTED_EDGE('',*,*,#9463,.T.);
#14364=ORIENTED_EDGE('',*,*,#10040,.F.);
#14365=ORIENTED_EDGE('',*,*,#9615,.F.);
#14366=ORIENTED_EDGE('',*,*,#10040,.T.);
#14367=ORIENTED_EDGE('',*,*,#9462,.T.);
#14368=ORIENTED_EDGE('',*,*,#9881,.F.);
#14369=ORIENTED_EDGE('',*,*,#9616,.F.);
#14370=ORIENTED_EDGE('',*,*,#9878,.T.);
#14371=ORIENTED_EDGE('',*,*,#9466,.T.);
#14372=ORIENTED_EDGE('',*,*,#10041,.F.);
#14373=ORIENTED_EDGE('',*,*,#9612,.F.);
#14374=ORIENTED_EDGE('',*,*,#10041,.T.);
#14375=ORIENTED_EDGE('',*,*,#9465,.T.);
#14376=ORIENTED_EDGE('',*,*,#9879,.F.);
#14377=ORIENTED_EDGE('',*,*,#9613,.F.);
#14378=ORIENTED_EDGE('',*,*,#9876,.T.);
#14379=ORIENTED_EDGE('',*,*,#9469,.T.);
#14380=ORIENTED_EDGE('',*,*,#10042,.F.);
#14381=ORIENTED_EDGE('',*,*,#9609,.F.);
#14382=ORIENTED_EDGE('',*,*,#10042,.T.);
#14383=ORIENTED_EDGE('',*,*,#9468,.T.);
#14384=ORIENTED_EDGE('',*,*,#9877,.F.);
#14385=ORIENTED_EDGE('',*,*,#9610,.F.);
#14386=ORIENTED_EDGE('',*,*,#9874,.T.);
#14387=ORIENTED_EDGE('',*,*,#9472,.T.);
#14388=ORIENTED_EDGE('',*,*,#10043,.F.);
#14389=ORIENTED_EDGE('',*,*,#9606,.F.);
#14390=ORIENTED_EDGE('',*,*,#10043,.T.);
#14391=ORIENTED_EDGE('',*,*,#9471,.T.);
#14392=ORIENTED_EDGE('',*,*,#9875,.F.);
#14393=ORIENTED_EDGE('',*,*,#9607,.F.);
#14394=ORIENTED_EDGE('',*,*,#9872,.T.);
#14395=ORIENTED_EDGE('',*,*,#9475,.T.);
#14396=ORIENTED_EDGE('',*,*,#10044,.F.);
#14397=ORIENTED_EDGE('',*,*,#9603,.F.);
#14398=ORIENTED_EDGE('',*,*,#10044,.T.);
#14399=ORIENTED_EDGE('',*,*,#9474,.T.);
#14400=ORIENTED_EDGE('',*,*,#9873,.F.);
#14401=ORIENTED_EDGE('',*,*,#9604,.F.);
#14402=ORIENTED_EDGE('',*,*,#9870,.T.);
#14403=ORIENTED_EDGE('',*,*,#9478,.T.);
#14404=ORIENTED_EDGE('',*,*,#10045,.F.);
#14405=ORIENTED_EDGE('',*,*,#9600,.F.);
#14406=ORIENTED_EDGE('',*,*,#10045,.T.);
#14407=ORIENTED_EDGE('',*,*,#9477,.T.);
#14408=ORIENTED_EDGE('',*,*,#9871,.F.);
#14409=ORIENTED_EDGE('',*,*,#9601,.F.);
#14410=ORIENTED_EDGE('',*,*,#9868,.T.);
#14411=ORIENTED_EDGE('',*,*,#9484,.T.);
#14412=ORIENTED_EDGE('',*,*,#10046,.F.);
#14413=ORIENTED_EDGE('',*,*,#9831,.F.);
#14414=ORIENTED_EDGE('',*,*,#10046,.T.);
#14415=ORIENTED_EDGE('',*,*,#9483,.T.);
#14416=ORIENTED_EDGE('',*,*,#9480,.T.);
#14417=ORIENTED_EDGE('',*,*,#9869,.F.);
#14418=ORIENTED_EDGE('',*,*,#9598,.F.);
#14419=ORIENTED_EDGE('',*,*,#9866,.T.);
#14420=ORIENTED_EDGE('',*,*,#9487,.T.);
#14421=ORIENTED_EDGE('',*,*,#10047,.F.);
#14422=ORIENTED_EDGE('',*,*,#9828,.F.);
#14423=ORIENTED_EDGE('',*,*,#10047,.T.);
#14424=ORIENTED_EDGE('',*,*,#9486,.T.);
#14425=ORIENTED_EDGE('',*,*,#9867,.F.);
#14426=ORIENTED_EDGE('',*,*,#9829,.F.);
#14427=ORIENTED_EDGE('',*,*,#9864,.T.);
#14428=ORIENTED_EDGE('',*,*,#9490,.T.);
#14429=ORIENTED_EDGE('',*,*,#10048,.F.);
#14430=ORIENTED_EDGE('',*,*,#9825,.F.);
#14431=ORIENTED_EDGE('',*,*,#10048,.T.);
#14432=ORIENTED_EDGE('',*,*,#9489,.T.);
#14433=ORIENTED_EDGE('',*,*,#9865,.F.);
#14434=ORIENTED_EDGE('',*,*,#9826,.F.);
#14435=ORIENTED_EDGE('',*,*,#9862,.T.);
#14436=ORIENTED_EDGE('',*,*,#9493,.T.);
#14437=ORIENTED_EDGE('',*,*,#10049,.F.);
#14438=ORIENTED_EDGE('',*,*,#9822,.F.);
#14439=ORIENTED_EDGE('',*,*,#10049,.T.);
#14440=ORIENTED_EDGE('',*,*,#9492,.T.);
#14441=ORIENTED_EDGE('',*,*,#9863,.F.);
#14442=ORIENTED_EDGE('',*,*,#9823,.F.);
#14443=ORIENTED_EDGE('',*,*,#9860,.T.);
#14444=ORIENTED_EDGE('',*,*,#9496,.T.);
#14445=ORIENTED_EDGE('',*,*,#10050,.F.);
#14446=ORIENTED_EDGE('',*,*,#9819,.F.);
#14447=ORIENTED_EDGE('',*,*,#10050,.T.);
#14448=ORIENTED_EDGE('',*,*,#9495,.T.);
#14449=ORIENTED_EDGE('',*,*,#9861,.F.);
#14450=ORIENTED_EDGE('',*,*,#9820,.F.);
#14451=ORIENTED_EDGE('',*,*,#9858,.T.);
#14452=ORIENTED_EDGE('',*,*,#9499,.T.);
#14453=ORIENTED_EDGE('',*,*,#10051,.F.);
#14454=ORIENTED_EDGE('',*,*,#9816,.F.);
#14455=ORIENTED_EDGE('',*,*,#10051,.T.);
#14456=ORIENTED_EDGE('',*,*,#9498,.T.);
#14457=ORIENTED_EDGE('',*,*,#9859,.F.);
#14458=ORIENTED_EDGE('',*,*,#9817,.F.);
#14459=ORIENTED_EDGE('',*,*,#9856,.T.);
#14460=ORIENTED_EDGE('',*,*,#9502,.T.);
#14461=ORIENTED_EDGE('',*,*,#10052,.F.);
#14462=ORIENTED_EDGE('',*,*,#9813,.F.);
#14463=ORIENTED_EDGE('',*,*,#10052,.T.);
#14464=ORIENTED_EDGE('',*,*,#9501,.T.);
#14465=ORIENTED_EDGE('',*,*,#9857,.F.);
#14466=ORIENTED_EDGE('',*,*,#9814,.F.);
#14467=ORIENTED_EDGE('',*,*,#9854,.T.);
#14468=ORIENTED_EDGE('',*,*,#9505,.T.);
#14469=ORIENTED_EDGE('',*,*,#10053,.F.);
#14470=ORIENTED_EDGE('',*,*,#9810,.F.);
#14471=ORIENTED_EDGE('',*,*,#10053,.T.);
#14472=ORIENTED_EDGE('',*,*,#9504,.T.);
#14473=ORIENTED_EDGE('',*,*,#9855,.F.);
#14474=ORIENTED_EDGE('',*,*,#9811,.F.);
#14475=ORIENTED_EDGE('',*,*,#9852,.T.);
#14476=ORIENTED_EDGE('',*,*,#9508,.T.);
#14477=ORIENTED_EDGE('',*,*,#10054,.F.);
#14478=ORIENTED_EDGE('',*,*,#9807,.F.);
#14479=ORIENTED_EDGE('',*,*,#10054,.T.);
#14480=ORIENTED_EDGE('',*,*,#9507,.T.);
#14481=ORIENTED_EDGE('',*,*,#9853,.F.);
#14482=ORIENTED_EDGE('',*,*,#9808,.F.);
#14483=ORIENTED_EDGE('',*,*,#9850,.T.);
#14484=ORIENTED_EDGE('',*,*,#9511,.T.);
#14485=ORIENTED_EDGE('',*,*,#10055,.F.);
#14486=ORIENTED_EDGE('',*,*,#9804,.F.);
#14487=ORIENTED_EDGE('',*,*,#10055,.T.);
#14488=ORIENTED_EDGE('',*,*,#9510,.T.);
#14489=ORIENTED_EDGE('',*,*,#9851,.F.);
#14490=ORIENTED_EDGE('',*,*,#9805,.F.);
#14491=ORIENTED_EDGE('',*,*,#9848,.T.);
#14492=ORIENTED_EDGE('',*,*,#9514,.T.);
#14493=ORIENTED_EDGE('',*,*,#10056,.F.);
#14494=ORIENTED_EDGE('',*,*,#9801,.F.);
#14495=ORIENTED_EDGE('',*,*,#10056,.T.);
#14496=ORIENTED_EDGE('',*,*,#9513,.T.);
#14497=ORIENTED_EDGE('',*,*,#9849,.F.);
#14498=ORIENTED_EDGE('',*,*,#9802,.F.);
#14499=ORIENTED_EDGE('',*,*,#9846,.T.);
#14500=ORIENTED_EDGE('',*,*,#9517,.T.);
#14501=ORIENTED_EDGE('',*,*,#10057,.F.);
#14502=ORIENTED_EDGE('',*,*,#9798,.F.);
#14503=ORIENTED_EDGE('',*,*,#10057,.T.);
#14504=ORIENTED_EDGE('',*,*,#9516,.T.);
#14505=ORIENTED_EDGE('',*,*,#9847,.F.);
#14506=ORIENTED_EDGE('',*,*,#9799,.F.);
#14507=ORIENTED_EDGE('',*,*,#9844,.T.);
#14508=ORIENTED_EDGE('',*,*,#9520,.T.);
#14509=ORIENTED_EDGE('',*,*,#10058,.F.);
#14510=ORIENTED_EDGE('',*,*,#9795,.F.);
#14511=ORIENTED_EDGE('',*,*,#10058,.T.);
#14512=ORIENTED_EDGE('',*,*,#9519,.T.);
#14513=ORIENTED_EDGE('',*,*,#9845,.F.);
#14514=ORIENTED_EDGE('',*,*,#9796,.F.);
#14515=ORIENTED_EDGE('',*,*,#9842,.T.);
#14516=ORIENTED_EDGE('',*,*,#9523,.T.);
#14517=ORIENTED_EDGE('',*,*,#10059,.F.);
#14518=ORIENTED_EDGE('',*,*,#9792,.F.);
#14519=ORIENTED_EDGE('',*,*,#10059,.T.);
#14520=ORIENTED_EDGE('',*,*,#9522,.T.);
#14521=ORIENTED_EDGE('',*,*,#9843,.F.);
#14522=ORIENTED_EDGE('',*,*,#9793,.F.);
#14523=ORIENTED_EDGE('',*,*,#9840,.T.);
#14524=ORIENTED_EDGE('',*,*,#9526,.T.);
#14525=ORIENTED_EDGE('',*,*,#10060,.F.);
#14526=ORIENTED_EDGE('',*,*,#9789,.F.);
#14527=ORIENTED_EDGE('',*,*,#10060,.T.);
#14528=ORIENTED_EDGE('',*,*,#9525,.T.);
#14529=ORIENTED_EDGE('',*,*,#9841,.F.);
#14530=ORIENTED_EDGE('',*,*,#9790,.F.);
#14531=ORIENTED_EDGE('',*,*,#9838,.T.);
#14532=ORIENTED_EDGE('',*,*,#9529,.T.);
#14533=ORIENTED_EDGE('',*,*,#10061,.F.);
#14534=ORIENTED_EDGE('',*,*,#9786,.F.);
#14535=ORIENTED_EDGE('',*,*,#10061,.T.);
#14536=ORIENTED_EDGE('',*,*,#9528,.T.);
#14537=ORIENTED_EDGE('',*,*,#9839,.F.);
#14538=ORIENTED_EDGE('',*,*,#9787,.F.);
#14539=ORIENTED_EDGE('',*,*,#9836,.T.);
#14540=ORIENTED_EDGE('',*,*,#9532,.T.);
#14541=ORIENTED_EDGE('',*,*,#10062,.F.);
#14542=ORIENTED_EDGE('',*,*,#9783,.F.);
#14543=ORIENTED_EDGE('',*,*,#10062,.T.);
#14544=ORIENTED_EDGE('',*,*,#9531,.T.);
#14545=ORIENTED_EDGE('',*,*,#9837,.F.);
#14546=ORIENTED_EDGE('',*,*,#9784,.F.);
#14547=ORIENTED_EDGE('',*,*,#9833,.T.);
#14548=ORIENTED_EDGE('',*,*,#9535,.T.);
#14549=ORIENTED_EDGE('',*,*,#10063,.F.);
#14550=ORIENTED_EDGE('',*,*,#9780,.F.);
#14551=ORIENTED_EDGE('',*,*,#10063,.T.);
#14552=ORIENTED_EDGE('',*,*,#9534,.T.);
#14553=ORIENTED_EDGE('',*,*,#9835,.F.);
#14554=ORIENTED_EDGE('',*,*,#9781,.F.);
#14555=ORIENTED_EDGE('',*,*,#10064,.T.);
#14556=ORIENTED_EDGE('',*,*,#10065,.F.);
#14557=ORIENTED_EDGE('',*,*,#10066,.F.);
#14558=ORIENTED_EDGE('',*,*,#10067,.F.);
#14559=ORIENTED_EDGE('',*,*,#10068,.T.);
#14560=ORIENTED_EDGE('',*,*,#10069,.T.);
#14561=ORIENTED_EDGE('',*,*,#10070,.F.);
#14562=ORIENTED_EDGE('',*,*,#10071,.F.);
#14563=ORIENTED_EDGE('',*,*,#10069,.F.);
#14564=ORIENTED_EDGE('',*,*,#10072,.T.);
#14565=ORIENTED_EDGE('',*,*,#10073,.F.);
#14566=ORIENTED_EDGE('',*,*,#10074,.F.);
#14567=ORIENTED_EDGE('',*,*,#10075,.F.);
#14568=ORIENTED_EDGE('',*,*,#10076,.T.);
#14569=ORIENTED_EDGE('',*,*,#10077,.T.);
#14570=ORIENTED_EDGE('',*,*,#10070,.T.);
#14571=ORIENTED_EDGE('',*,*,#10071,.T.);
#14572=ORIENTED_EDGE('',*,*,#10077,.F.);
#14573=ORIENTED_EDGE('',*,*,#10078,.F.);
#14574=ORIENTED_EDGE('',*,*,#10079,.T.);
#14575=ORIENTED_EDGE('',*,*,#10080,.T.);
#14576=ORIENTED_EDGE('',*,*,#10079,.F.);
#14577=ORIENTED_EDGE('',*,*,#10081,.F.);
#14578=ORIENTED_EDGE('',*,*,#10074,.T.);
#14579=ORIENTED_EDGE('',*,*,#10080,.F.);
#14580=ORIENTED_EDGE('',*,*,#10082,.F.);
#14581=ORIENTED_EDGE('',*,*,#10066,.T.);
#14582=ORIENTED_EDGE('',*,*,#10076,.F.);
#14583=ORIENTED_EDGE('',*,*,#10078,.T.);
#14584=ORIENTED_EDGE('',*,*,#10073,.T.);
#14585=ORIENTED_EDGE('',*,*,#10083,.F.);
#14586=ORIENTED_EDGE('',*,*,#10075,.T.);
#14587=ORIENTED_EDGE('',*,*,#10081,.T.);
#14588=ORIENTED_EDGE('',*,*,#10067,.T.);
#14589=ORIENTED_EDGE('',*,*,#10082,.T.);
#14590=ORIENTED_EDGE('',*,*,#10065,.T.);
#14591=ORIENTED_EDGE('',*,*,#10084,.F.);
#14592=ORIENTED_EDGE('',*,*,#10084,.T.);
#14593=ORIENTED_EDGE('',*,*,#10064,.F.);
#14594=ORIENTED_EDGE('',*,*,#10083,.T.);
#14595=ORIENTED_EDGE('',*,*,#10072,.F.);
#14596=ORIENTED_EDGE('',*,*,#10068,.F.);
#14597=ORIENTED_EDGE('',*,*,#10085,.F.);
#14598=ORIENTED_EDGE('',*,*,#10086,.T.);
#14599=ORIENTED_EDGE('',*,*,#10087,.F.);
#14600=ORIENTED_EDGE('',*,*,#10086,.F.);
#14601=ORIENTED_EDGE('',*,*,#10088,.F.);
#14602=ORIENTED_EDGE('',*,*,#10089,.F.);
#14603=ORIENTED_EDGE('',*,*,#10090,.T.);
#14604=ORIENTED_EDGE('',*,*,#10091,.T.);
#14605=ORIENTED_EDGE('',*,*,#10090,.F.);
#14606=ORIENTED_EDGE('',*,*,#10092,.F.);
#14607=ORIENTED_EDGE('',*,*,#10093,.F.);
#14608=ORIENTED_EDGE('',*,*,#10094,.T.);
#14609=ORIENTED_EDGE('',*,*,#10095,.T.);
#14610=ORIENTED_EDGE('',*,*,#10096,.T.);
#14611=ORIENTED_EDGE('',*,*,#10094,.F.);
#14612=ORIENTED_EDGE('',*,*,#10088,.T.);
#14613=ORIENTED_EDGE('',*,*,#10089,.T.);
#14614=ORIENTED_EDGE('',*,*,#10097,.T.);
#14615=ORIENTED_EDGE('',*,*,#10095,.F.);
#14616=ORIENTED_EDGE('',*,*,#10096,.F.);
#14617=ORIENTED_EDGE('',*,*,#10097,.F.);
#14618=ORIENTED_EDGE('',*,*,#10098,.F.);
#14619=ORIENTED_EDGE('',*,*,#10099,.F.);
#14620=ORIENTED_EDGE('',*,*,#10100,.T.);
#14621=ORIENTED_EDGE('',*,*,#10092,.T.);
#14622=ORIENTED_EDGE('',*,*,#10093,.T.);
#14623=ORIENTED_EDGE('',*,*,#10100,.F.);
#14624=ORIENTED_EDGE('',*,*,#10101,.F.);
#14625=ORIENTED_EDGE('',*,*,#10102,.F.);
#14626=ORIENTED_EDGE('',*,*,#10103,.T.);
#14627=ORIENTED_EDGE('',*,*,#10104,.T.);
#14628=ORIENTED_EDGE('',*,*,#10105,.T.);
#14629=ORIENTED_EDGE('',*,*,#10103,.F.);
#14630=ORIENTED_EDGE('',*,*,#10098,.T.);
#14631=ORIENTED_EDGE('',*,*,#10099,.T.);
#14632=ORIENTED_EDGE('',*,*,#10106,.T.);
#14633=ORIENTED_EDGE('',*,*,#10104,.F.);
#14634=ORIENTED_EDGE('',*,*,#10105,.F.);
#14635=ORIENTED_EDGE('',*,*,#10106,.F.);
#14636=ORIENTED_EDGE('',*,*,#10107,.F.);
#14637=ORIENTED_EDGE('',*,*,#10108,.F.);
#14638=ORIENTED_EDGE('',*,*,#10109,.T.);
#14639=ORIENTED_EDGE('',*,*,#10101,.T.);
#14640=ORIENTED_EDGE('',*,*,#10102,.T.);
#14641=ORIENTED_EDGE('',*,*,#10109,.F.);
#14642=ORIENTED_EDGE('',*,*,#10110,.F.);
#14643=ORIENTED_EDGE('',*,*,#10111,.F.);
#14644=ORIENTED_EDGE('',*,*,#10112,.T.);
#14645=ORIENTED_EDGE('',*,*,#10113,.T.);
#14646=ORIENTED_EDGE('',*,*,#10114,.T.);
#14647=ORIENTED_EDGE('',*,*,#10112,.F.);
#14648=ORIENTED_EDGE('',*,*,#10107,.T.);
#14649=ORIENTED_EDGE('',*,*,#10108,.T.);
#14650=ORIENTED_EDGE('',*,*,#10115,.T.);
#14651=ORIENTED_EDGE('',*,*,#10113,.F.);
#14652=ORIENTED_EDGE('',*,*,#10114,.F.);
#14653=ORIENTED_EDGE('',*,*,#10115,.F.);
#14654=ORIENTED_EDGE('',*,*,#10116,.F.);
#14655=ORIENTED_EDGE('',*,*,#10117,.F.);
#14656=ORIENTED_EDGE('',*,*,#10118,.T.);
#14657=ORIENTED_EDGE('',*,*,#10110,.T.);
#14658=ORIENTED_EDGE('',*,*,#10111,.T.);
#14659=ORIENTED_EDGE('',*,*,#10118,.F.);
#14660=ORIENTED_EDGE('',*,*,#10119,.F.);
#14661=ORIENTED_EDGE('',*,*,#10120,.F.);
#14662=ORIENTED_EDGE('',*,*,#10121,.T.);
#14663=ORIENTED_EDGE('',*,*,#10122,.T.);
#14664=ORIENTED_EDGE('',*,*,#10123,.T.);
#14665=ORIENTED_EDGE('',*,*,#10121,.F.);
#14666=ORIENTED_EDGE('',*,*,#10116,.T.);
#14667=ORIENTED_EDGE('',*,*,#10117,.T.);
#14668=ORIENTED_EDGE('',*,*,#10124,.T.);
#14669=ORIENTED_EDGE('',*,*,#10122,.F.);
#14670=ORIENTED_EDGE('',*,*,#10123,.F.);
#14671=ORIENTED_EDGE('',*,*,#10124,.F.);
#14672=ORIENTED_EDGE('',*,*,#10125,.F.);
#14673=ORIENTED_EDGE('',*,*,#10126,.F.);
#14674=ORIENTED_EDGE('',*,*,#10127,.T.);
#14675=ORIENTED_EDGE('',*,*,#10119,.T.);
#14676=ORIENTED_EDGE('',*,*,#10120,.T.);
#14677=ORIENTED_EDGE('',*,*,#10127,.F.);
#14678=ORIENTED_EDGE('',*,*,#10128,.F.);
#14679=ORIENTED_EDGE('',*,*,#10129,.F.);
#14680=ORIENTED_EDGE('',*,*,#10130,.T.);
#14681=ORIENTED_EDGE('',*,*,#10131,.T.);
#14682=ORIENTED_EDGE('',*,*,#10132,.T.);
#14683=ORIENTED_EDGE('',*,*,#10130,.F.);
#14684=ORIENTED_EDGE('',*,*,#10125,.T.);
#14685=ORIENTED_EDGE('',*,*,#10126,.T.);
#14686=ORIENTED_EDGE('',*,*,#10133,.T.);
#14687=ORIENTED_EDGE('',*,*,#10131,.F.);
#14688=ORIENTED_EDGE('',*,*,#10132,.F.);
#14689=ORIENTED_EDGE('',*,*,#10133,.F.);
#14690=ORIENTED_EDGE('',*,*,#10134,.F.);
#14691=ORIENTED_EDGE('',*,*,#10135,.F.);
#14692=ORIENTED_EDGE('',*,*,#10136,.T.);
#14693=ORIENTED_EDGE('',*,*,#10128,.T.);
#14694=ORIENTED_EDGE('',*,*,#10129,.T.);
#14695=ORIENTED_EDGE('',*,*,#10136,.F.);
#14696=ORIENTED_EDGE('',*,*,#10137,.F.);
#14697=ORIENTED_EDGE('',*,*,#10138,.F.);
#14698=ORIENTED_EDGE('',*,*,#10139,.T.);
#14699=ORIENTED_EDGE('',*,*,#10140,.T.);
#14700=ORIENTED_EDGE('',*,*,#10141,.T.);
#14701=ORIENTED_EDGE('',*,*,#10139,.F.);
#14702=ORIENTED_EDGE('',*,*,#10134,.T.);
#14703=ORIENTED_EDGE('',*,*,#10135,.T.);
#14704=ORIENTED_EDGE('',*,*,#10142,.T.);
#14705=ORIENTED_EDGE('',*,*,#10140,.F.);
#14706=ORIENTED_EDGE('',*,*,#10141,.F.);
#14707=ORIENTED_EDGE('',*,*,#10142,.F.);
#14708=ORIENTED_EDGE('',*,*,#10143,.F.);
#14709=ORIENTED_EDGE('',*,*,#10144,.F.);
#14710=ORIENTED_EDGE('',*,*,#10145,.T.);
#14711=ORIENTED_EDGE('',*,*,#10137,.T.);
#14712=ORIENTED_EDGE('',*,*,#10138,.T.);
#14713=ORIENTED_EDGE('',*,*,#10145,.F.);
#14714=ORIENTED_EDGE('',*,*,#10146,.F.);
#14715=ORIENTED_EDGE('',*,*,#10147,.F.);
#14716=ORIENTED_EDGE('',*,*,#10148,.T.);
#14717=ORIENTED_EDGE('',*,*,#10149,.T.);
#14718=ORIENTED_EDGE('',*,*,#10150,.T.);
#14719=ORIENTED_EDGE('',*,*,#10148,.F.);
#14720=ORIENTED_EDGE('',*,*,#10143,.T.);
#14721=ORIENTED_EDGE('',*,*,#10144,.T.);
#14722=ORIENTED_EDGE('',*,*,#10151,.T.);
#14723=ORIENTED_EDGE('',*,*,#10149,.F.);
#14724=ORIENTED_EDGE('',*,*,#10150,.F.);
#14725=ORIENTED_EDGE('',*,*,#10151,.F.);
#14726=ORIENTED_EDGE('',*,*,#10152,.F.);
#14727=ORIENTED_EDGE('',*,*,#10153,.F.);
#14728=ORIENTED_EDGE('',*,*,#10154,.T.);
#14729=ORIENTED_EDGE('',*,*,#10146,.T.);
#14730=ORIENTED_EDGE('',*,*,#10147,.T.);
#14731=ORIENTED_EDGE('',*,*,#10154,.F.);
#14732=ORIENTED_EDGE('',*,*,#10155,.F.);
#14733=ORIENTED_EDGE('',*,*,#10156,.F.);
#14734=ORIENTED_EDGE('',*,*,#10157,.T.);
#14735=ORIENTED_EDGE('',*,*,#10158,.T.);
#14736=ORIENTED_EDGE('',*,*,#10159,.T.);
#14737=ORIENTED_EDGE('',*,*,#10157,.F.);
#14738=ORIENTED_EDGE('',*,*,#10152,.T.);
#14739=ORIENTED_EDGE('',*,*,#10153,.T.);
#14740=ORIENTED_EDGE('',*,*,#10160,.T.);
#14741=ORIENTED_EDGE('',*,*,#10158,.F.);
#14742=ORIENTED_EDGE('',*,*,#10159,.F.);
#14743=ORIENTED_EDGE('',*,*,#10160,.F.);
#14744=ORIENTED_EDGE('',*,*,#10161,.F.);
#14745=ORIENTED_EDGE('',*,*,#10162,.F.);
#14746=ORIENTED_EDGE('',*,*,#10163,.T.);
#14747=ORIENTED_EDGE('',*,*,#10155,.T.);
#14748=ORIENTED_EDGE('',*,*,#10156,.T.);
#14749=ORIENTED_EDGE('',*,*,#10163,.F.);
#14750=ORIENTED_EDGE('',*,*,#10164,.F.);
#14751=ORIENTED_EDGE('',*,*,#10165,.F.);
#14752=ORIENTED_EDGE('',*,*,#10166,.T.);
#14753=ORIENTED_EDGE('',*,*,#10167,.T.);
#14754=ORIENTED_EDGE('',*,*,#10168,.T.);
#14755=ORIENTED_EDGE('',*,*,#10166,.F.);
#14756=ORIENTED_EDGE('',*,*,#10161,.T.);
#14757=ORIENTED_EDGE('',*,*,#10162,.T.);
#14758=ORIENTED_EDGE('',*,*,#10169,.T.);
#14759=ORIENTED_EDGE('',*,*,#10167,.F.);
#14760=ORIENTED_EDGE('',*,*,#10168,.F.);
#14761=ORIENTED_EDGE('',*,*,#10169,.F.);
#14762=ORIENTED_EDGE('',*,*,#10170,.F.);
#14763=ORIENTED_EDGE('',*,*,#10171,.F.);
#14764=ORIENTED_EDGE('',*,*,#10172,.T.);
#14765=ORIENTED_EDGE('',*,*,#10164,.T.);
#14766=ORIENTED_EDGE('',*,*,#10165,.T.);
#14767=ORIENTED_EDGE('',*,*,#10172,.F.);
#14768=ORIENTED_EDGE('',*,*,#10173,.F.);
#14769=ORIENTED_EDGE('',*,*,#10174,.F.);
#14770=ORIENTED_EDGE('',*,*,#10175,.T.);
#14771=ORIENTED_EDGE('',*,*,#10176,.T.);
#14772=ORIENTED_EDGE('',*,*,#10177,.T.);
#14773=ORIENTED_EDGE('',*,*,#10175,.F.);
#14774=ORIENTED_EDGE('',*,*,#10170,.T.);
#14775=ORIENTED_EDGE('',*,*,#10171,.T.);
#14776=ORIENTED_EDGE('',*,*,#10178,.T.);
#14777=ORIENTED_EDGE('',*,*,#10176,.F.);
#14778=ORIENTED_EDGE('',*,*,#10177,.F.);
#14779=ORIENTED_EDGE('',*,*,#10178,.F.);
#14780=ORIENTED_EDGE('',*,*,#10179,.F.);
#14781=ORIENTED_EDGE('',*,*,#10180,.F.);
#14782=ORIENTED_EDGE('',*,*,#10181,.T.);
#14783=ORIENTED_EDGE('',*,*,#10173,.T.);
#14784=ORIENTED_EDGE('',*,*,#10174,.T.);
#14785=ORIENTED_EDGE('',*,*,#10181,.F.);
#14786=ORIENTED_EDGE('',*,*,#10182,.F.);
#14787=ORIENTED_EDGE('',*,*,#10183,.F.);
#14788=ORIENTED_EDGE('',*,*,#10184,.T.);
#14789=ORIENTED_EDGE('',*,*,#10185,.T.);
#14790=ORIENTED_EDGE('',*,*,#10186,.T.);
#14791=ORIENTED_EDGE('',*,*,#10184,.F.);
#14792=ORIENTED_EDGE('',*,*,#10179,.T.);
#14793=ORIENTED_EDGE('',*,*,#10180,.T.);
#14794=ORIENTED_EDGE('',*,*,#10187,.T.);
#14795=ORIENTED_EDGE('',*,*,#10185,.F.);
#14796=ORIENTED_EDGE('',*,*,#10186,.F.);
#14797=ORIENTED_EDGE('',*,*,#10187,.F.);
#14798=ORIENTED_EDGE('',*,*,#10188,.F.);
#14799=ORIENTED_EDGE('',*,*,#10189,.F.);
#14800=ORIENTED_EDGE('',*,*,#10190,.T.);
#14801=ORIENTED_EDGE('',*,*,#10182,.T.);
#14802=ORIENTED_EDGE('',*,*,#10183,.T.);
#14803=ORIENTED_EDGE('',*,*,#10190,.F.);
#14804=ORIENTED_EDGE('',*,*,#10191,.F.);
#14805=ORIENTED_EDGE('',*,*,#10192,.F.);
#14806=ORIENTED_EDGE('',*,*,#10193,.T.);
#14807=ORIENTED_EDGE('',*,*,#10194,.T.);
#14808=ORIENTED_EDGE('',*,*,#10195,.T.);
#14809=ORIENTED_EDGE('',*,*,#10193,.F.);
#14810=ORIENTED_EDGE('',*,*,#10188,.T.);
#14811=ORIENTED_EDGE('',*,*,#10189,.T.);
#14812=ORIENTED_EDGE('',*,*,#10196,.T.);
#14813=ORIENTED_EDGE('',*,*,#10194,.F.);
#14814=ORIENTED_EDGE('',*,*,#10195,.F.);
#14815=ORIENTED_EDGE('',*,*,#10196,.F.);
#14816=ORIENTED_EDGE('',*,*,#10197,.F.);
#14817=ORIENTED_EDGE('',*,*,#10198,.F.);
#14818=ORIENTED_EDGE('',*,*,#10199,.T.);
#14819=ORIENTED_EDGE('',*,*,#10191,.T.);
#14820=ORIENTED_EDGE('',*,*,#10192,.T.);
#14821=ORIENTED_EDGE('',*,*,#10199,.F.);
#14822=ORIENTED_EDGE('',*,*,#10200,.F.);
#14823=ORIENTED_EDGE('',*,*,#10201,.F.);
#14824=ORIENTED_EDGE('',*,*,#10202,.T.);
#14825=ORIENTED_EDGE('',*,*,#10203,.T.);
#14826=ORIENTED_EDGE('',*,*,#10204,.T.);
#14827=ORIENTED_EDGE('',*,*,#10202,.F.);
#14828=ORIENTED_EDGE('',*,*,#10197,.T.);
#14829=ORIENTED_EDGE('',*,*,#10198,.T.);
#14830=ORIENTED_EDGE('',*,*,#10205,.T.);
#14831=ORIENTED_EDGE('',*,*,#10203,.F.);
#14832=ORIENTED_EDGE('',*,*,#10204,.F.);
#14833=ORIENTED_EDGE('',*,*,#10205,.F.);
#14834=ORIENTED_EDGE('',*,*,#10087,.T.);
#14835=ORIENTED_EDGE('',*,*,#10206,.T.);
#14836=ORIENTED_EDGE('',*,*,#10207,.T.);
#14837=ORIENTED_EDGE('',*,*,#10206,.F.);
#14838=ORIENTED_EDGE('',*,*,#10208,.T.);
#14839=ORIENTED_EDGE('',*,*,#10209,.F.);
#14840=ORIENTED_EDGE('',*,*,#10210,.T.);
#14841=ORIENTED_EDGE('',*,*,#10211,.T.);
#14842=ORIENTED_EDGE('',*,*,#10212,.F.);
#14843=ORIENTED_EDGE('',*,*,#10213,.T.);
#14844=ORIENTED_EDGE('',*,*,#10214,.T.);
#14845=ORIENTED_EDGE('',*,*,#10215,.F.);
#14846=ORIENTED_EDGE('',*,*,#10216,.T.);
#14847=ORIENTED_EDGE('',*,*,#10217,.T.);
#14848=ORIENTED_EDGE('',*,*,#10218,.F.);
#14849=ORIENTED_EDGE('',*,*,#10219,.T.);
#14850=ORIENTED_EDGE('',*,*,#10220,.T.);
#14851=ORIENTED_EDGE('',*,*,#10221,.F.);
#14852=ORIENTED_EDGE('',*,*,#10222,.T.);
#14853=ORIENTED_EDGE('',*,*,#10223,.T.);
#14854=ORIENTED_EDGE('',*,*,#10224,.F.);
#14855=ORIENTED_EDGE('',*,*,#10225,.T.);
#14856=ORIENTED_EDGE('',*,*,#10226,.T.);
#14857=ORIENTED_EDGE('',*,*,#10227,.F.);
#14858=ORIENTED_EDGE('',*,*,#10228,.T.);
#14859=ORIENTED_EDGE('',*,*,#10229,.T.);
#14860=ORIENTED_EDGE('',*,*,#10230,.F.);
#14861=ORIENTED_EDGE('',*,*,#10231,.T.);
#14862=ORIENTED_EDGE('',*,*,#10232,.T.);
#14863=ORIENTED_EDGE('',*,*,#10233,.F.);
#14864=ORIENTED_EDGE('',*,*,#10234,.T.);
#14865=ORIENTED_EDGE('',*,*,#10235,.T.);
#14866=ORIENTED_EDGE('',*,*,#10236,.F.);
#14867=ORIENTED_EDGE('',*,*,#10237,.T.);
#14868=ORIENTED_EDGE('',*,*,#10238,.T.);
#14869=ORIENTED_EDGE('',*,*,#10239,.F.);
#14870=ORIENTED_EDGE('',*,*,#10240,.T.);
#14871=ORIENTED_EDGE('',*,*,#10241,.T.);
#14872=ORIENTED_EDGE('',*,*,#10242,.F.);
#14873=ORIENTED_EDGE('',*,*,#10243,.T.);
#14874=ORIENTED_EDGE('',*,*,#10244,.T.);
#14875=ORIENTED_EDGE('',*,*,#10245,.F.);
#14876=ORIENTED_EDGE('',*,*,#10246,.T.);
#14877=ORIENTED_EDGE('',*,*,#10247,.T.);
#14878=ORIENTED_EDGE('',*,*,#10248,.F.);
#14879=ORIENTED_EDGE('',*,*,#10249,.T.);
#14880=ORIENTED_EDGE('',*,*,#10250,.T.);
#14881=ORIENTED_EDGE('',*,*,#10251,.F.);
#14882=ORIENTED_EDGE('',*,*,#10252,.T.);
#14883=ORIENTED_EDGE('',*,*,#10253,.T.);
#14884=ORIENTED_EDGE('',*,*,#10254,.F.);
#14885=ORIENTED_EDGE('',*,*,#10255,.T.);
#14886=ORIENTED_EDGE('',*,*,#10256,.T.);
#14887=ORIENTED_EDGE('',*,*,#10257,.F.);
#14888=ORIENTED_EDGE('',*,*,#10258,.T.);
#14889=ORIENTED_EDGE('',*,*,#10259,.T.);
#14890=ORIENTED_EDGE('',*,*,#10260,.F.);
#14891=ORIENTED_EDGE('',*,*,#10261,.T.);
#14892=ORIENTED_EDGE('',*,*,#10262,.T.);
#14893=ORIENTED_EDGE('',*,*,#10263,.F.);
#14894=ORIENTED_EDGE('',*,*,#10264,.T.);
#14895=ORIENTED_EDGE('',*,*,#10265,.T.);
#14896=ORIENTED_EDGE('',*,*,#10266,.F.);
#14897=ORIENTED_EDGE('',*,*,#10267,.T.);
#14898=ORIENTED_EDGE('',*,*,#10268,.T.);
#14899=ORIENTED_EDGE('',*,*,#10269,.F.);
#14900=ORIENTED_EDGE('',*,*,#10270,.T.);
#14901=ORIENTED_EDGE('',*,*,#10271,.T.);
#14902=ORIENTED_EDGE('',*,*,#10272,.F.);
#14903=ORIENTED_EDGE('',*,*,#10273,.T.);
#14904=ORIENTED_EDGE('',*,*,#10274,.T.);
#14905=ORIENTED_EDGE('',*,*,#10275,.F.);
#14906=ORIENTED_EDGE('',*,*,#10276,.T.);
#14907=ORIENTED_EDGE('',*,*,#10277,.T.);
#14908=ORIENTED_EDGE('',*,*,#10278,.F.);
#14909=ORIENTED_EDGE('',*,*,#10279,.T.);
#14910=ORIENTED_EDGE('',*,*,#10280,.T.);
#14911=ORIENTED_EDGE('',*,*,#10281,.F.);
#14912=ORIENTED_EDGE('',*,*,#10282,.T.);
#14913=ORIENTED_EDGE('',*,*,#10283,.T.);
#14914=ORIENTED_EDGE('',*,*,#10284,.F.);
#14915=ORIENTED_EDGE('',*,*,#10285,.T.);
#14916=ORIENTED_EDGE('',*,*,#10286,.T.);
#14917=ORIENTED_EDGE('',*,*,#10287,.F.);
#14918=ORIENTED_EDGE('',*,*,#10288,.T.);
#14919=ORIENTED_EDGE('',*,*,#10289,.T.);
#14920=ORIENTED_EDGE('',*,*,#10290,.F.);
#14921=ORIENTED_EDGE('',*,*,#10291,.T.);
#14922=ORIENTED_EDGE('',*,*,#10292,.T.);
#14923=ORIENTED_EDGE('',*,*,#10293,.F.);
#14924=ORIENTED_EDGE('',*,*,#10294,.T.);
#14925=ORIENTED_EDGE('',*,*,#10295,.T.);
#14926=ORIENTED_EDGE('',*,*,#10296,.F.);
#14927=ORIENTED_EDGE('',*,*,#10297,.T.);
#14928=ORIENTED_EDGE('',*,*,#10298,.T.);
#14929=ORIENTED_EDGE('',*,*,#10299,.F.);
#14930=ORIENTED_EDGE('',*,*,#10300,.T.);
#14931=ORIENTED_EDGE('',*,*,#10301,.T.);
#14932=ORIENTED_EDGE('',*,*,#10302,.F.);
#14933=ORIENTED_EDGE('',*,*,#10303,.T.);
#14934=ORIENTED_EDGE('',*,*,#10304,.T.);
#14935=ORIENTED_EDGE('',*,*,#10305,.F.);
#14936=ORIENTED_EDGE('',*,*,#10306,.T.);
#14937=ORIENTED_EDGE('',*,*,#10307,.T.);
#14938=ORIENTED_EDGE('',*,*,#10308,.F.);
#14939=ORIENTED_EDGE('',*,*,#10309,.T.);
#14940=ORIENTED_EDGE('',*,*,#10310,.T.);
#14941=ORIENTED_EDGE('',*,*,#10311,.F.);
#14942=ORIENTED_EDGE('',*,*,#10312,.T.);
#14943=ORIENTED_EDGE('',*,*,#10313,.T.);
#14944=ORIENTED_EDGE('',*,*,#10314,.F.);
#14945=ORIENTED_EDGE('',*,*,#10315,.T.);
#14946=ORIENTED_EDGE('',*,*,#10316,.T.);
#14947=ORIENTED_EDGE('',*,*,#10317,.F.);
#14948=ORIENTED_EDGE('',*,*,#10318,.T.);
#14949=ORIENTED_EDGE('',*,*,#10319,.T.);
#14950=ORIENTED_EDGE('',*,*,#10320,.F.);
#14951=ORIENTED_EDGE('',*,*,#10321,.T.);
#14952=ORIENTED_EDGE('',*,*,#10322,.T.);
#14953=ORIENTED_EDGE('',*,*,#10323,.F.);
#14954=ORIENTED_EDGE('',*,*,#10324,.T.);
#14955=ORIENTED_EDGE('',*,*,#10325,.T.);
#14956=ORIENTED_EDGE('',*,*,#10326,.T.);
#14957=ORIENTED_EDGE('',*,*,#10325,.F.);
#14958=ORIENTED_EDGE('',*,*,#10327,.T.);
#14959=ORIENTED_EDGE('',*,*,#10328,.T.);
#14960=ORIENTED_EDGE('',*,*,#10329,.F.);
#14961=ORIENTED_EDGE('',*,*,#10330,.T.);
#14962=ORIENTED_EDGE('',*,*,#10331,.T.);
#14963=ORIENTED_EDGE('',*,*,#10332,.F.);
#14964=ORIENTED_EDGE('',*,*,#10333,.T.);
#14965=ORIENTED_EDGE('',*,*,#10334,.T.);
#14966=ORIENTED_EDGE('',*,*,#10335,.F.);
#14967=ORIENTED_EDGE('',*,*,#10336,.T.);
#14968=ORIENTED_EDGE('',*,*,#10337,.T.);
#14969=ORIENTED_EDGE('',*,*,#10338,.F.);
#14970=ORIENTED_EDGE('',*,*,#10339,.T.);
#14971=ORIENTED_EDGE('',*,*,#10340,.T.);
#14972=ORIENTED_EDGE('',*,*,#10341,.F.);
#14973=ORIENTED_EDGE('',*,*,#10342,.T.);
#14974=ORIENTED_EDGE('',*,*,#10343,.T.);
#14975=ORIENTED_EDGE('',*,*,#10344,.F.);
#14976=ORIENTED_EDGE('',*,*,#10345,.T.);
#14977=ORIENTED_EDGE('',*,*,#10346,.T.);
#14978=ORIENTED_EDGE('',*,*,#10347,.F.);
#14979=ORIENTED_EDGE('',*,*,#10348,.T.);
#14980=ORIENTED_EDGE('',*,*,#10349,.T.);
#14981=ORIENTED_EDGE('',*,*,#10350,.F.);
#14982=ORIENTED_EDGE('',*,*,#10351,.T.);
#14983=ORIENTED_EDGE('',*,*,#10352,.T.);
#14984=ORIENTED_EDGE('',*,*,#10353,.F.);
#14985=ORIENTED_EDGE('',*,*,#10354,.T.);
#14986=ORIENTED_EDGE('',*,*,#10355,.T.);
#14987=ORIENTED_EDGE('',*,*,#10356,.F.);
#14988=ORIENTED_EDGE('',*,*,#10357,.T.);
#14989=ORIENTED_EDGE('',*,*,#10358,.T.);
#14990=ORIENTED_EDGE('',*,*,#10359,.F.);
#14991=ORIENTED_EDGE('',*,*,#10360,.T.);
#14992=ORIENTED_EDGE('',*,*,#10361,.T.);
#14993=ORIENTED_EDGE('',*,*,#10362,.F.);
#14994=ORIENTED_EDGE('',*,*,#10363,.T.);
#14995=ORIENTED_EDGE('',*,*,#10364,.T.);
#14996=ORIENTED_EDGE('',*,*,#10365,.F.);
#14997=ORIENTED_EDGE('',*,*,#10366,.T.);
#14998=ORIENTED_EDGE('',*,*,#10367,.T.);
#14999=ORIENTED_EDGE('',*,*,#10368,.F.);
#15000=ORIENTED_EDGE('',*,*,#10369,.T.);
#15001=ORIENTED_EDGE('',*,*,#10370,.T.);
#15002=ORIENTED_EDGE('',*,*,#10371,.F.);
#15003=ORIENTED_EDGE('',*,*,#10372,.T.);
#15004=ORIENTED_EDGE('',*,*,#10373,.T.);
#15005=ORIENTED_EDGE('',*,*,#10374,.F.);
#15006=ORIENTED_EDGE('',*,*,#10375,.T.);
#15007=ORIENTED_EDGE('',*,*,#10376,.T.);
#15008=ORIENTED_EDGE('',*,*,#10377,.F.);
#15009=ORIENTED_EDGE('',*,*,#10378,.T.);
#15010=ORIENTED_EDGE('',*,*,#10379,.T.);
#15011=ORIENTED_EDGE('',*,*,#10380,.F.);
#15012=ORIENTED_EDGE('',*,*,#10381,.T.);
#15013=ORIENTED_EDGE('',*,*,#10382,.T.);
#15014=ORIENTED_EDGE('',*,*,#10383,.F.);
#15015=ORIENTED_EDGE('',*,*,#10384,.T.);
#15016=ORIENTED_EDGE('',*,*,#10385,.T.);
#15017=ORIENTED_EDGE('',*,*,#10386,.F.);
#15018=ORIENTED_EDGE('',*,*,#10387,.T.);
#15019=ORIENTED_EDGE('',*,*,#10388,.T.);
#15020=ORIENTED_EDGE('',*,*,#10389,.F.);
#15021=ORIENTED_EDGE('',*,*,#10390,.T.);
#15022=ORIENTED_EDGE('',*,*,#10391,.T.);
#15023=ORIENTED_EDGE('',*,*,#10392,.F.);
#15024=ORIENTED_EDGE('',*,*,#10393,.T.);
#15025=ORIENTED_EDGE('',*,*,#10394,.T.);
#15026=ORIENTED_EDGE('',*,*,#10395,.F.);
#15027=ORIENTED_EDGE('',*,*,#10396,.T.);
#15028=ORIENTED_EDGE('',*,*,#10397,.T.);
#15029=ORIENTED_EDGE('',*,*,#10398,.F.);
#15030=ORIENTED_EDGE('',*,*,#10399,.T.);
#15031=ORIENTED_EDGE('',*,*,#10400,.T.);
#15032=ORIENTED_EDGE('',*,*,#10401,.F.);
#15033=ORIENTED_EDGE('',*,*,#10402,.T.);
#15034=ORIENTED_EDGE('',*,*,#10403,.T.);
#15035=ORIENTED_EDGE('',*,*,#10404,.F.);
#15036=ORIENTED_EDGE('',*,*,#10405,.T.);
#15037=ORIENTED_EDGE('',*,*,#10406,.T.);
#15038=ORIENTED_EDGE('',*,*,#10407,.F.);
#15039=ORIENTED_EDGE('',*,*,#10408,.T.);
#15040=ORIENTED_EDGE('',*,*,#10409,.T.);
#15041=ORIENTED_EDGE('',*,*,#10410,.F.);
#15042=ORIENTED_EDGE('',*,*,#10411,.T.);
#15043=ORIENTED_EDGE('',*,*,#10412,.T.);
#15044=ORIENTED_EDGE('',*,*,#10413,.F.);
#15045=ORIENTED_EDGE('',*,*,#10414,.T.);
#15046=ORIENTED_EDGE('',*,*,#10415,.T.);
#15047=ORIENTED_EDGE('',*,*,#10416,.F.);
#15048=ORIENTED_EDGE('',*,*,#10417,.T.);
#15049=ORIENTED_EDGE('',*,*,#10418,.T.);
#15050=ORIENTED_EDGE('',*,*,#10419,.F.);
#15051=ORIENTED_EDGE('',*,*,#10420,.T.);
#15052=ORIENTED_EDGE('',*,*,#10421,.T.);
#15053=ORIENTED_EDGE('',*,*,#10422,.F.);
#15054=ORIENTED_EDGE('',*,*,#10423,.T.);
#15055=ORIENTED_EDGE('',*,*,#10424,.T.);
#15056=ORIENTED_EDGE('',*,*,#10425,.F.);
#15057=ORIENTED_EDGE('',*,*,#10426,.T.);
#15058=ORIENTED_EDGE('',*,*,#10427,.T.);
#15059=ORIENTED_EDGE('',*,*,#10428,.F.);
#15060=ORIENTED_EDGE('',*,*,#10429,.T.);
#15061=ORIENTED_EDGE('',*,*,#10430,.T.);
#15062=ORIENTED_EDGE('',*,*,#10431,.F.);
#15063=ORIENTED_EDGE('',*,*,#10432,.T.);
#15064=ORIENTED_EDGE('',*,*,#10433,.T.);
#15065=ORIENTED_EDGE('',*,*,#10434,.F.);
#15066=ORIENTED_EDGE('',*,*,#10435,.T.);
#15067=ORIENTED_EDGE('',*,*,#10436,.T.);
#15068=ORIENTED_EDGE('',*,*,#10437,.F.);
#15069=ORIENTED_EDGE('',*,*,#10438,.T.);
#15070=ORIENTED_EDGE('',*,*,#10439,.T.);
#15071=ORIENTED_EDGE('',*,*,#10440,.F.);
#15072=ORIENTED_EDGE('',*,*,#10441,.T.);
#15073=ORIENTED_EDGE('',*,*,#10442,.F.);
#15074=ORIENTED_EDGE('',*,*,#10443,.T.);
#15075=ORIENTED_EDGE('',*,*,#10444,.F.);
#15076=ORIENTED_EDGE('',*,*,#10445,.F.);
#15077=ORIENTED_EDGE('',*,*,#10446,.T.);
#15078=ORIENTED_EDGE('',*,*,#10447,.F.);
#15079=ORIENTED_EDGE('',*,*,#10448,.F.);
#15080=ORIENTED_EDGE('',*,*,#10449,.T.);
#15081=ORIENTED_EDGE('',*,*,#10450,.F.);
#15082=ORIENTED_EDGE('',*,*,#10451,.F.);
#15083=ORIENTED_EDGE('',*,*,#10452,.T.);
#15084=ORIENTED_EDGE('',*,*,#10453,.F.);
#15085=ORIENTED_EDGE('',*,*,#10454,.F.);
#15086=ORIENTED_EDGE('',*,*,#10455,.T.);
#15087=ORIENTED_EDGE('',*,*,#10456,.F.);
#15088=ORIENTED_EDGE('',*,*,#10457,.F.);
#15089=ORIENTED_EDGE('',*,*,#10458,.T.);
#15090=ORIENTED_EDGE('',*,*,#10459,.F.);
#15091=ORIENTED_EDGE('',*,*,#10460,.F.);
#15092=ORIENTED_EDGE('',*,*,#10461,.T.);
#15093=ORIENTED_EDGE('',*,*,#10462,.F.);
#15094=ORIENTED_EDGE('',*,*,#10463,.F.);
#15095=ORIENTED_EDGE('',*,*,#10464,.T.);
#15096=ORIENTED_EDGE('',*,*,#10465,.F.);
#15097=ORIENTED_EDGE('',*,*,#10466,.F.);
#15098=ORIENTED_EDGE('',*,*,#10467,.T.);
#15099=ORIENTED_EDGE('',*,*,#10468,.F.);
#15100=ORIENTED_EDGE('',*,*,#10469,.F.);
#15101=ORIENTED_EDGE('',*,*,#10470,.T.);
#15102=ORIENTED_EDGE('',*,*,#10471,.F.);
#15103=ORIENTED_EDGE('',*,*,#10472,.F.);
#15104=ORIENTED_EDGE('',*,*,#10473,.T.);
#15105=ORIENTED_EDGE('',*,*,#10474,.F.);
#15106=ORIENTED_EDGE('',*,*,#10475,.F.);
#15107=ORIENTED_EDGE('',*,*,#10476,.T.);
#15108=ORIENTED_EDGE('',*,*,#10477,.F.);
#15109=ORIENTED_EDGE('',*,*,#10478,.F.);
#15110=ORIENTED_EDGE('',*,*,#10479,.T.);
#15111=ORIENTED_EDGE('',*,*,#10480,.F.);
#15112=ORIENTED_EDGE('',*,*,#10481,.F.);
#15113=ORIENTED_EDGE('',*,*,#10482,.T.);
#15114=ORIENTED_EDGE('',*,*,#10483,.F.);
#15115=ORIENTED_EDGE('',*,*,#10484,.F.);
#15116=ORIENTED_EDGE('',*,*,#10485,.T.);
#15117=ORIENTED_EDGE('',*,*,#10486,.F.);
#15118=ORIENTED_EDGE('',*,*,#10487,.F.);
#15119=ORIENTED_EDGE('',*,*,#10488,.T.);
#15120=ORIENTED_EDGE('',*,*,#10489,.F.);
#15121=ORIENTED_EDGE('',*,*,#10490,.F.);
#15122=ORIENTED_EDGE('',*,*,#10491,.T.);
#15123=ORIENTED_EDGE('',*,*,#10492,.F.);
#15124=ORIENTED_EDGE('',*,*,#10493,.F.);
#15125=ORIENTED_EDGE('',*,*,#10494,.T.);
#15126=ORIENTED_EDGE('',*,*,#10495,.F.);
#15127=ORIENTED_EDGE('',*,*,#10496,.F.);
#15128=ORIENTED_EDGE('',*,*,#10497,.T.);
#15129=ORIENTED_EDGE('',*,*,#10498,.F.);
#15130=ORIENTED_EDGE('',*,*,#10499,.F.);
#15131=ORIENTED_EDGE('',*,*,#10500,.T.);
#15132=ORIENTED_EDGE('',*,*,#10501,.F.);
#15133=ORIENTED_EDGE('',*,*,#10502,.F.);
#15134=ORIENTED_EDGE('',*,*,#10503,.T.);
#15135=ORIENTED_EDGE('',*,*,#10504,.F.);
#15136=ORIENTED_EDGE('',*,*,#10505,.F.);
#15137=ORIENTED_EDGE('',*,*,#10506,.T.);
#15138=ORIENTED_EDGE('',*,*,#10507,.F.);
#15139=ORIENTED_EDGE('',*,*,#10508,.F.);
#15140=ORIENTED_EDGE('',*,*,#10509,.T.);
#15141=ORIENTED_EDGE('',*,*,#10510,.F.);
#15142=ORIENTED_EDGE('',*,*,#10511,.F.);
#15143=ORIENTED_EDGE('',*,*,#10512,.T.);
#15144=ORIENTED_EDGE('',*,*,#10513,.F.);
#15145=ORIENTED_EDGE('',*,*,#10514,.F.);
#15146=ORIENTED_EDGE('',*,*,#10515,.T.);
#15147=ORIENTED_EDGE('',*,*,#10516,.F.);
#15148=ORIENTED_EDGE('',*,*,#10517,.F.);
#15149=ORIENTED_EDGE('',*,*,#10518,.T.);
#15150=ORIENTED_EDGE('',*,*,#10519,.F.);
#15151=ORIENTED_EDGE('',*,*,#10520,.F.);
#15152=ORIENTED_EDGE('',*,*,#10521,.T.);
#15153=ORIENTED_EDGE('',*,*,#10522,.F.);
#15154=ORIENTED_EDGE('',*,*,#10523,.F.);
#15155=ORIENTED_EDGE('',*,*,#10524,.T.);
#15156=ORIENTED_EDGE('',*,*,#10525,.F.);
#15157=ORIENTED_EDGE('',*,*,#10526,.F.);
#15158=ORIENTED_EDGE('',*,*,#10527,.T.);
#15159=ORIENTED_EDGE('',*,*,#10528,.F.);
#15160=ORIENTED_EDGE('',*,*,#10529,.F.);
#15161=ORIENTED_EDGE('',*,*,#10530,.T.);
#15162=ORIENTED_EDGE('',*,*,#10531,.F.);
#15163=ORIENTED_EDGE('',*,*,#10532,.F.);
#15164=ORIENTED_EDGE('',*,*,#10533,.T.);
#15165=ORIENTED_EDGE('',*,*,#10534,.F.);
#15166=ORIENTED_EDGE('',*,*,#10535,.F.);
#15167=ORIENTED_EDGE('',*,*,#10536,.T.);
#15168=ORIENTED_EDGE('',*,*,#10537,.F.);
#15169=ORIENTED_EDGE('',*,*,#10538,.F.);
#15170=ORIENTED_EDGE('',*,*,#10539,.T.);
#15171=ORIENTED_EDGE('',*,*,#10540,.F.);
#15172=ORIENTED_EDGE('',*,*,#10541,.F.);
#15173=ORIENTED_EDGE('',*,*,#10542,.T.);
#15174=ORIENTED_EDGE('',*,*,#10543,.F.);
#15175=ORIENTED_EDGE('',*,*,#10544,.F.);
#15176=ORIENTED_EDGE('',*,*,#10545,.T.);
#15177=ORIENTED_EDGE('',*,*,#10546,.F.);
#15178=ORIENTED_EDGE('',*,*,#10547,.F.);
#15179=ORIENTED_EDGE('',*,*,#10548,.T.);
#15180=ORIENTED_EDGE('',*,*,#10549,.F.);
#15181=ORIENTED_EDGE('',*,*,#10550,.F.);
#15182=ORIENTED_EDGE('',*,*,#10551,.T.);
#15183=ORIENTED_EDGE('',*,*,#10552,.F.);
#15184=ORIENTED_EDGE('',*,*,#10553,.F.);
#15185=ORIENTED_EDGE('',*,*,#10554,.T.);
#15186=ORIENTED_EDGE('',*,*,#10555,.F.);
#15187=ORIENTED_EDGE('',*,*,#10556,.F.);
#15188=ORIENTED_EDGE('',*,*,#10557,.T.);
#15189=ORIENTED_EDGE('',*,*,#10558,.F.);
#15190=ORIENTED_EDGE('',*,*,#10559,.T.);
#15191=ORIENTED_EDGE('',*,*,#10560,.F.);
#15192=ORIENTED_EDGE('',*,*,#10559,.F.);
#15193=ORIENTED_EDGE('',*,*,#10561,.F.);
#15194=ORIENTED_EDGE('',*,*,#10562,.F.);
#15195=ORIENTED_EDGE('',*,*,#10563,.T.);
#15196=ORIENTED_EDGE('',*,*,#10564,.F.);
#15197=ORIENTED_EDGE('',*,*,#10565,.F.);
#15198=ORIENTED_EDGE('',*,*,#10566,.T.);
#15199=ORIENTED_EDGE('',*,*,#10567,.F.);
#15200=ORIENTED_EDGE('',*,*,#10568,.F.);
#15201=ORIENTED_EDGE('',*,*,#10569,.T.);
#15202=ORIENTED_EDGE('',*,*,#10570,.F.);
#15203=ORIENTED_EDGE('',*,*,#10571,.F.);
#15204=ORIENTED_EDGE('',*,*,#10572,.T.);
#15205=ORIENTED_EDGE('',*,*,#10573,.F.);
#15206=ORIENTED_EDGE('',*,*,#10574,.F.);
#15207=ORIENTED_EDGE('',*,*,#10575,.T.);
#15208=ORIENTED_EDGE('',*,*,#10576,.F.);
#15209=ORIENTED_EDGE('',*,*,#10577,.F.);
#15210=ORIENTED_EDGE('',*,*,#10578,.T.);
#15211=ORIENTED_EDGE('',*,*,#10579,.F.);
#15212=ORIENTED_EDGE('',*,*,#10580,.F.);
#15213=ORIENTED_EDGE('',*,*,#10581,.T.);
#15214=ORIENTED_EDGE('',*,*,#10582,.F.);
#15215=ORIENTED_EDGE('',*,*,#10583,.F.);
#15216=ORIENTED_EDGE('',*,*,#10584,.T.);
#15217=ORIENTED_EDGE('',*,*,#10585,.F.);
#15218=ORIENTED_EDGE('',*,*,#10586,.F.);
#15219=ORIENTED_EDGE('',*,*,#10587,.T.);
#15220=ORIENTED_EDGE('',*,*,#10588,.F.);
#15221=ORIENTED_EDGE('',*,*,#10589,.F.);
#15222=ORIENTED_EDGE('',*,*,#10590,.T.);
#15223=ORIENTED_EDGE('',*,*,#10591,.F.);
#15224=ORIENTED_EDGE('',*,*,#10592,.F.);
#15225=ORIENTED_EDGE('',*,*,#10593,.T.);
#15226=ORIENTED_EDGE('',*,*,#10594,.F.);
#15227=ORIENTED_EDGE('',*,*,#10595,.F.);
#15228=ORIENTED_EDGE('',*,*,#10596,.T.);
#15229=ORIENTED_EDGE('',*,*,#10597,.F.);
#15230=ORIENTED_EDGE('',*,*,#10598,.F.);
#15231=ORIENTED_EDGE('',*,*,#10599,.T.);
#15232=ORIENTED_EDGE('',*,*,#10600,.F.);
#15233=ORIENTED_EDGE('',*,*,#10601,.F.);
#15234=ORIENTED_EDGE('',*,*,#10602,.T.);
#15235=ORIENTED_EDGE('',*,*,#10603,.F.);
#15236=ORIENTED_EDGE('',*,*,#10604,.F.);
#15237=ORIENTED_EDGE('',*,*,#10605,.T.);
#15238=ORIENTED_EDGE('',*,*,#10606,.F.);
#15239=ORIENTED_EDGE('',*,*,#10607,.F.);
#15240=ORIENTED_EDGE('',*,*,#10608,.T.);
#15241=ORIENTED_EDGE('',*,*,#10609,.F.);
#15242=ORIENTED_EDGE('',*,*,#10610,.F.);
#15243=ORIENTED_EDGE('',*,*,#10611,.T.);
#15244=ORIENTED_EDGE('',*,*,#10612,.F.);
#15245=ORIENTED_EDGE('',*,*,#10613,.F.);
#15246=ORIENTED_EDGE('',*,*,#10614,.T.);
#15247=ORIENTED_EDGE('',*,*,#10615,.F.);
#15248=ORIENTED_EDGE('',*,*,#10616,.F.);
#15249=ORIENTED_EDGE('',*,*,#10617,.T.);
#15250=ORIENTED_EDGE('',*,*,#10618,.F.);
#15251=ORIENTED_EDGE('',*,*,#10619,.F.);
#15252=ORIENTED_EDGE('',*,*,#10620,.T.);
#15253=ORIENTED_EDGE('',*,*,#10621,.F.);
#15254=ORIENTED_EDGE('',*,*,#10622,.F.);
#15255=ORIENTED_EDGE('',*,*,#10623,.T.);
#15256=ORIENTED_EDGE('',*,*,#10624,.F.);
#15257=ORIENTED_EDGE('',*,*,#10625,.F.);
#15258=ORIENTED_EDGE('',*,*,#10626,.T.);
#15259=ORIENTED_EDGE('',*,*,#10627,.F.);
#15260=ORIENTED_EDGE('',*,*,#10628,.F.);
#15261=ORIENTED_EDGE('',*,*,#10629,.T.);
#15262=ORIENTED_EDGE('',*,*,#10630,.F.);
#15263=ORIENTED_EDGE('',*,*,#10631,.F.);
#15264=ORIENTED_EDGE('',*,*,#10632,.T.);
#15265=ORIENTED_EDGE('',*,*,#10633,.F.);
#15266=ORIENTED_EDGE('',*,*,#10634,.F.);
#15267=ORIENTED_EDGE('',*,*,#10635,.T.);
#15268=ORIENTED_EDGE('',*,*,#10636,.F.);
#15269=ORIENTED_EDGE('',*,*,#10637,.F.);
#15270=ORIENTED_EDGE('',*,*,#10638,.T.);
#15271=ORIENTED_EDGE('',*,*,#10639,.F.);
#15272=ORIENTED_EDGE('',*,*,#10640,.F.);
#15273=ORIENTED_EDGE('',*,*,#10641,.T.);
#15274=ORIENTED_EDGE('',*,*,#10642,.F.);
#15275=ORIENTED_EDGE('',*,*,#10643,.F.);
#15276=ORIENTED_EDGE('',*,*,#10644,.T.);
#15277=ORIENTED_EDGE('',*,*,#10645,.F.);
#15278=ORIENTED_EDGE('',*,*,#10646,.F.);
#15279=ORIENTED_EDGE('',*,*,#10647,.T.);
#15280=ORIENTED_EDGE('',*,*,#10648,.F.);
#15281=ORIENTED_EDGE('',*,*,#10649,.F.);
#15282=ORIENTED_EDGE('',*,*,#10650,.T.);
#15283=ORIENTED_EDGE('',*,*,#10651,.F.);
#15284=ORIENTED_EDGE('',*,*,#10652,.F.);
#15285=ORIENTED_EDGE('',*,*,#10653,.T.);
#15286=ORIENTED_EDGE('',*,*,#10654,.F.);
#15287=ORIENTED_EDGE('',*,*,#10655,.F.);
#15288=ORIENTED_EDGE('',*,*,#10656,.T.);
#15289=ORIENTED_EDGE('',*,*,#10657,.F.);
#15290=ORIENTED_EDGE('',*,*,#10658,.F.);
#15291=ORIENTED_EDGE('',*,*,#10659,.T.);
#15292=ORIENTED_EDGE('',*,*,#10660,.F.);
#15293=ORIENTED_EDGE('',*,*,#10661,.F.);
#15294=ORIENTED_EDGE('',*,*,#10662,.T.);
#15295=ORIENTED_EDGE('',*,*,#10663,.F.);
#15296=ORIENTED_EDGE('',*,*,#10664,.F.);
#15297=ORIENTED_EDGE('',*,*,#10665,.T.);
#15298=ORIENTED_EDGE('',*,*,#10666,.F.);
#15299=ORIENTED_EDGE('',*,*,#10667,.F.);
#15300=ORIENTED_EDGE('',*,*,#10668,.T.);
#15301=ORIENTED_EDGE('',*,*,#10669,.F.);
#15302=ORIENTED_EDGE('',*,*,#10670,.F.);
#15303=ORIENTED_EDGE('',*,*,#10671,.T.);
#15304=ORIENTED_EDGE('',*,*,#10672,.F.);
#15305=ORIENTED_EDGE('',*,*,#10673,.F.);
#15306=ORIENTED_EDGE('',*,*,#10674,.T.);
#15307=ORIENTED_EDGE('',*,*,#10675,.F.);
#15308=ORIENTED_EDGE('',*,*,#10676,.F.);
#15309=ORIENTED_EDGE('',*,*,#10677,.T.);
#15310=ORIENTED_EDGE('',*,*,#10200,.T.);
#15311=ORIENTED_EDGE('',*,*,#10201,.T.);
#15312=ORIENTED_EDGE('',*,*,#10677,.F.);
#15313=ORIENTED_EDGE('',*,*,#10678,.F.);
#15314=ORIENTED_EDGE('',*,*,#10389,.T.);
#15315=ORIENTED_EDGE('',*,*,#10679,.T.);
#15316=ORIENTED_EDGE('',*,*,#10614,.F.);
#15317=ORIENTED_EDGE('',*,*,#10680,.T.);
#15318=ORIENTED_EDGE('',*,*,#10611,.F.);
#15319=ORIENTED_EDGE('',*,*,#10681,.F.);
#15320=ORIENTED_EDGE('',*,*,#10392,.T.);
#15321=ORIENTED_EDGE('',*,*,#10682,.T.);
#15322=ORIENTED_EDGE('',*,*,#10608,.F.);
#15323=ORIENTED_EDGE('',*,*,#10683,.F.);
#15324=ORIENTED_EDGE('',*,*,#10395,.T.);
#15325=ORIENTED_EDGE('',*,*,#10684,.T.);
#15326=ORIENTED_EDGE('',*,*,#10605,.F.);
#15327=ORIENTED_EDGE('',*,*,#10685,.F.);
#15328=ORIENTED_EDGE('',*,*,#10398,.T.);
#15329=ORIENTED_EDGE('',*,*,#10686,.T.);
#15330=ORIENTED_EDGE('',*,*,#10602,.F.);
#15331=ORIENTED_EDGE('',*,*,#10687,.F.);
#15332=ORIENTED_EDGE('',*,*,#10401,.T.);
#15333=ORIENTED_EDGE('',*,*,#10688,.T.);
#15334=ORIENTED_EDGE('',*,*,#10599,.F.);
#15335=ORIENTED_EDGE('',*,*,#10689,.F.);
#15336=ORIENTED_EDGE('',*,*,#10404,.T.);
#15337=ORIENTED_EDGE('',*,*,#10690,.T.);
#15338=ORIENTED_EDGE('',*,*,#10596,.F.);
#15339=ORIENTED_EDGE('',*,*,#10691,.F.);
#15340=ORIENTED_EDGE('',*,*,#10407,.T.);
#15341=ORIENTED_EDGE('',*,*,#10692,.T.);
#15342=ORIENTED_EDGE('',*,*,#10593,.F.);
#15343=ORIENTED_EDGE('',*,*,#10693,.F.);
#15344=ORIENTED_EDGE('',*,*,#10410,.T.);
#15345=ORIENTED_EDGE('',*,*,#10694,.T.);
#15346=ORIENTED_EDGE('',*,*,#10590,.F.);
#15347=ORIENTED_EDGE('',*,*,#10695,.F.);
#15348=ORIENTED_EDGE('',*,*,#10413,.T.);
#15349=ORIENTED_EDGE('',*,*,#10696,.T.);
#15350=ORIENTED_EDGE('',*,*,#10587,.F.);
#15351=ORIENTED_EDGE('',*,*,#10697,.F.);
#15352=ORIENTED_EDGE('',*,*,#10416,.T.);
#15353=ORIENTED_EDGE('',*,*,#10698,.T.);
#15354=ORIENTED_EDGE('',*,*,#10584,.F.);
#15355=ORIENTED_EDGE('',*,*,#10699,.F.);
#15356=ORIENTED_EDGE('',*,*,#10419,.T.);
#15357=ORIENTED_EDGE('',*,*,#10700,.T.);
#15358=ORIENTED_EDGE('',*,*,#10581,.F.);
#15359=ORIENTED_EDGE('',*,*,#10701,.F.);
#15360=ORIENTED_EDGE('',*,*,#10422,.T.);
#15361=ORIENTED_EDGE('',*,*,#10702,.T.);
#15362=ORIENTED_EDGE('',*,*,#10578,.F.);
#15363=ORIENTED_EDGE('',*,*,#10703,.F.);
#15364=ORIENTED_EDGE('',*,*,#10425,.T.);
#15365=ORIENTED_EDGE('',*,*,#10704,.T.);
#15366=ORIENTED_EDGE('',*,*,#10575,.F.);
#15367=ORIENTED_EDGE('',*,*,#10705,.F.);
#15368=ORIENTED_EDGE('',*,*,#10428,.T.);
#15369=ORIENTED_EDGE('',*,*,#10706,.T.);
#15370=ORIENTED_EDGE('',*,*,#10572,.F.);
#15371=ORIENTED_EDGE('',*,*,#10707,.F.);
#15372=ORIENTED_EDGE('',*,*,#10431,.T.);
#15373=ORIENTED_EDGE('',*,*,#10708,.T.);
#15374=ORIENTED_EDGE('',*,*,#10569,.F.);
#15375=ORIENTED_EDGE('',*,*,#10709,.F.);
#15376=ORIENTED_EDGE('',*,*,#10434,.T.);
#15377=ORIENTED_EDGE('',*,*,#10710,.T.);
#15378=ORIENTED_EDGE('',*,*,#10566,.F.);
#15379=ORIENTED_EDGE('',*,*,#10711,.F.);
#15380=ORIENTED_EDGE('',*,*,#10437,.T.);
#15381=ORIENTED_EDGE('',*,*,#10712,.T.);
#15382=ORIENTED_EDGE('',*,*,#10563,.F.);
#15383=ORIENTED_EDGE('',*,*,#10713,.F.);
#15384=ORIENTED_EDGE('',*,*,#10440,.T.);
#15385=ORIENTED_EDGE('',*,*,#10714,.T.);
#15386=ORIENTED_EDGE('',*,*,#10557,.F.);
#15387=ORIENTED_EDGE('',*,*,#10715,.F.);
#15388=ORIENTED_EDGE('',*,*,#10209,.T.);
#15389=ORIENTED_EDGE('',*,*,#10716,.T.);
#15390=ORIENTED_EDGE('',*,*,#10554,.F.);
#15391=ORIENTED_EDGE('',*,*,#10717,.F.);
#15392=ORIENTED_EDGE('',*,*,#10212,.T.);
#15393=ORIENTED_EDGE('',*,*,#10718,.T.);
#15394=ORIENTED_EDGE('',*,*,#10551,.F.);
#15395=ORIENTED_EDGE('',*,*,#10719,.F.);
#15396=ORIENTED_EDGE('',*,*,#10215,.T.);
#15397=ORIENTED_EDGE('',*,*,#10720,.T.);
#15398=ORIENTED_EDGE('',*,*,#10548,.F.);
#15399=ORIENTED_EDGE('',*,*,#10721,.F.);
#15400=ORIENTED_EDGE('',*,*,#10218,.T.);
#15401=ORIENTED_EDGE('',*,*,#10722,.T.);
#15402=ORIENTED_EDGE('',*,*,#10545,.F.);
#15403=ORIENTED_EDGE('',*,*,#10723,.F.);
#15404=ORIENTED_EDGE('',*,*,#10221,.T.);
#15405=ORIENTED_EDGE('',*,*,#10724,.T.);
#15406=ORIENTED_EDGE('',*,*,#10542,.F.);
#15407=ORIENTED_EDGE('',*,*,#10725,.F.);
#15408=ORIENTED_EDGE('',*,*,#10224,.T.);
#15409=ORIENTED_EDGE('',*,*,#10726,.T.);
#15410=ORIENTED_EDGE('',*,*,#10539,.F.);
#15411=ORIENTED_EDGE('',*,*,#10727,.F.);
#15412=ORIENTED_EDGE('',*,*,#10227,.T.);
#15413=ORIENTED_EDGE('',*,*,#10728,.T.);
#15414=ORIENTED_EDGE('',*,*,#10536,.F.);
#15415=ORIENTED_EDGE('',*,*,#10729,.F.);
#15416=ORIENTED_EDGE('',*,*,#10230,.T.);
#15417=ORIENTED_EDGE('',*,*,#10730,.T.);
#15418=ORIENTED_EDGE('',*,*,#10533,.F.);
#15419=ORIENTED_EDGE('',*,*,#10731,.F.);
#15420=ORIENTED_EDGE('',*,*,#10233,.T.);
#15421=ORIENTED_EDGE('',*,*,#10732,.T.);
#15422=ORIENTED_EDGE('',*,*,#10530,.F.);
#15423=ORIENTED_EDGE('',*,*,#10733,.F.);
#15424=ORIENTED_EDGE('',*,*,#10236,.T.);
#15425=ORIENTED_EDGE('',*,*,#10734,.T.);
#15426=ORIENTED_EDGE('',*,*,#10527,.F.);
#15427=ORIENTED_EDGE('',*,*,#10735,.F.);
#15428=ORIENTED_EDGE('',*,*,#10239,.T.);
#15429=ORIENTED_EDGE('',*,*,#10736,.T.);
#15430=ORIENTED_EDGE('',*,*,#10524,.F.);
#15431=ORIENTED_EDGE('',*,*,#10737,.F.);
#15432=ORIENTED_EDGE('',*,*,#10242,.T.);
#15433=ORIENTED_EDGE('',*,*,#10738,.T.);
#15434=ORIENTED_EDGE('',*,*,#10521,.F.);
#15435=ORIENTED_EDGE('',*,*,#10739,.F.);
#15436=ORIENTED_EDGE('',*,*,#10245,.T.);
#15437=ORIENTED_EDGE('',*,*,#10740,.T.);
#15438=ORIENTED_EDGE('',*,*,#10518,.F.);
#15439=ORIENTED_EDGE('',*,*,#10741,.F.);
#15440=ORIENTED_EDGE('',*,*,#10248,.T.);
#15441=ORIENTED_EDGE('',*,*,#10742,.T.);
#15442=ORIENTED_EDGE('',*,*,#10515,.F.);
#15443=ORIENTED_EDGE('',*,*,#10743,.F.);
#15444=ORIENTED_EDGE('',*,*,#10251,.T.);
#15445=ORIENTED_EDGE('',*,*,#10744,.T.);
#15446=ORIENTED_EDGE('',*,*,#10512,.F.);
#15447=ORIENTED_EDGE('',*,*,#10745,.F.);
#15448=ORIENTED_EDGE('',*,*,#10254,.T.);
#15449=ORIENTED_EDGE('',*,*,#10746,.T.);
#15450=ORIENTED_EDGE('',*,*,#10509,.F.);
#15451=ORIENTED_EDGE('',*,*,#10747,.F.);
#15452=ORIENTED_EDGE('',*,*,#10257,.T.);
#15453=ORIENTED_EDGE('',*,*,#10748,.T.);
#15454=ORIENTED_EDGE('',*,*,#10506,.F.);
#15455=ORIENTED_EDGE('',*,*,#10749,.F.);
#15456=ORIENTED_EDGE('',*,*,#10260,.T.);
#15457=ORIENTED_EDGE('',*,*,#10750,.T.);
#15458=ORIENTED_EDGE('',*,*,#10503,.F.);
#15459=ORIENTED_EDGE('',*,*,#10751,.F.);
#15460=ORIENTED_EDGE('',*,*,#10263,.T.);
#15461=ORIENTED_EDGE('',*,*,#10752,.T.);
#15462=ORIENTED_EDGE('',*,*,#10500,.F.);
#15463=ORIENTED_EDGE('',*,*,#10753,.F.);
#15464=ORIENTED_EDGE('',*,*,#10266,.T.);
#15465=ORIENTED_EDGE('',*,*,#10754,.T.);
#15466=ORIENTED_EDGE('',*,*,#10497,.F.);
#15467=ORIENTED_EDGE('',*,*,#10755,.F.);
#15468=ORIENTED_EDGE('',*,*,#10269,.T.);
#15469=ORIENTED_EDGE('',*,*,#10756,.T.);
#15470=ORIENTED_EDGE('',*,*,#10494,.F.);
#15471=ORIENTED_EDGE('',*,*,#10757,.F.);
#15472=ORIENTED_EDGE('',*,*,#10272,.T.);
#15473=ORIENTED_EDGE('',*,*,#10758,.T.);
#15474=ORIENTED_EDGE('',*,*,#10491,.F.);
#15475=ORIENTED_EDGE('',*,*,#10759,.F.);
#15476=ORIENTED_EDGE('',*,*,#10275,.T.);
#15477=ORIENTED_EDGE('',*,*,#10760,.T.);
#15478=ORIENTED_EDGE('',*,*,#10488,.F.);
#15479=ORIENTED_EDGE('',*,*,#10761,.F.);
#15480=ORIENTED_EDGE('',*,*,#10278,.T.);
#15481=ORIENTED_EDGE('',*,*,#10762,.T.);
#15482=ORIENTED_EDGE('',*,*,#10485,.F.);
#15483=ORIENTED_EDGE('',*,*,#10763,.F.);
#15484=ORIENTED_EDGE('',*,*,#10281,.T.);
#15485=ORIENTED_EDGE('',*,*,#10764,.T.);
#15486=ORIENTED_EDGE('',*,*,#10482,.F.);
#15487=ORIENTED_EDGE('',*,*,#10765,.F.);
#15488=ORIENTED_EDGE('',*,*,#10284,.T.);
#15489=ORIENTED_EDGE('',*,*,#10766,.T.);
#15490=ORIENTED_EDGE('',*,*,#10479,.F.);
#15491=ORIENTED_EDGE('',*,*,#10767,.F.);
#15492=ORIENTED_EDGE('',*,*,#10287,.T.);
#15493=ORIENTED_EDGE('',*,*,#10768,.T.);
#15494=ORIENTED_EDGE('',*,*,#10476,.F.);
#15495=ORIENTED_EDGE('',*,*,#10769,.F.);
#15496=ORIENTED_EDGE('',*,*,#10290,.T.);
#15497=ORIENTED_EDGE('',*,*,#10770,.T.);
#15498=ORIENTED_EDGE('',*,*,#10473,.F.);
#15499=ORIENTED_EDGE('',*,*,#10771,.F.);
#15500=ORIENTED_EDGE('',*,*,#10293,.T.);
#15501=ORIENTED_EDGE('',*,*,#10772,.T.);
#15502=ORIENTED_EDGE('',*,*,#10470,.F.);
#15503=ORIENTED_EDGE('',*,*,#10773,.F.);
#15504=ORIENTED_EDGE('',*,*,#10296,.T.);
#15505=ORIENTED_EDGE('',*,*,#10774,.T.);
#15506=ORIENTED_EDGE('',*,*,#10467,.F.);
#15507=ORIENTED_EDGE('',*,*,#10775,.F.);
#15508=ORIENTED_EDGE('',*,*,#10299,.T.);
#15509=ORIENTED_EDGE('',*,*,#10776,.T.);
#15510=ORIENTED_EDGE('',*,*,#10464,.F.);
#15511=ORIENTED_EDGE('',*,*,#10777,.F.);
#15512=ORIENTED_EDGE('',*,*,#10302,.T.);
#15513=ORIENTED_EDGE('',*,*,#10778,.T.);
#15514=ORIENTED_EDGE('',*,*,#10461,.F.);
#15515=ORIENTED_EDGE('',*,*,#10779,.F.);
#15516=ORIENTED_EDGE('',*,*,#10305,.T.);
#15517=ORIENTED_EDGE('',*,*,#10780,.T.);
#15518=ORIENTED_EDGE('',*,*,#10458,.F.);
#15519=ORIENTED_EDGE('',*,*,#10781,.F.);
#15520=ORIENTED_EDGE('',*,*,#10308,.T.);
#15521=ORIENTED_EDGE('',*,*,#10782,.T.);
#15522=ORIENTED_EDGE('',*,*,#10455,.F.);
#15523=ORIENTED_EDGE('',*,*,#10783,.F.);
#15524=ORIENTED_EDGE('',*,*,#10311,.T.);
#15525=ORIENTED_EDGE('',*,*,#10784,.T.);
#15526=ORIENTED_EDGE('',*,*,#10452,.F.);
#15527=ORIENTED_EDGE('',*,*,#10785,.F.);
#15528=ORIENTED_EDGE('',*,*,#10314,.T.);
#15529=ORIENTED_EDGE('',*,*,#10786,.T.);
#15530=ORIENTED_EDGE('',*,*,#10449,.F.);
#15531=ORIENTED_EDGE('',*,*,#10787,.F.);
#15532=ORIENTED_EDGE('',*,*,#10317,.T.);
#15533=ORIENTED_EDGE('',*,*,#10788,.T.);
#15534=ORIENTED_EDGE('',*,*,#10446,.F.);
#15535=ORIENTED_EDGE('',*,*,#10789,.F.);
#15536=ORIENTED_EDGE('',*,*,#10320,.T.);
#15537=ORIENTED_EDGE('',*,*,#10790,.T.);
#15538=ORIENTED_EDGE('',*,*,#10443,.F.);
#15539=ORIENTED_EDGE('',*,*,#10791,.F.);
#15540=ORIENTED_EDGE('',*,*,#10323,.T.);
#15541=ORIENTED_EDGE('',*,*,#10792,.T.);
#15542=ORIENTED_EDGE('',*,*,#10674,.F.);
#15543=ORIENTED_EDGE('',*,*,#10793,.F.);
#15544=ORIENTED_EDGE('',*,*,#10329,.T.);
#15545=ORIENTED_EDGE('',*,*,#10794,.T.);
#15546=ORIENTED_EDGE('',*,*,#10671,.F.);
#15547=ORIENTED_EDGE('',*,*,#10795,.F.);
#15548=ORIENTED_EDGE('',*,*,#10332,.T.);
#15549=ORIENTED_EDGE('',*,*,#10796,.T.);
#15550=ORIENTED_EDGE('',*,*,#10668,.F.);
#15551=ORIENTED_EDGE('',*,*,#10797,.F.);
#15552=ORIENTED_EDGE('',*,*,#10335,.T.);
#15553=ORIENTED_EDGE('',*,*,#10798,.T.);
#15554=ORIENTED_EDGE('',*,*,#10665,.F.);
#15555=ORIENTED_EDGE('',*,*,#10799,.F.);
#15556=ORIENTED_EDGE('',*,*,#10338,.T.);
#15557=ORIENTED_EDGE('',*,*,#10800,.T.);
#15558=ORIENTED_EDGE('',*,*,#10662,.F.);
#15559=ORIENTED_EDGE('',*,*,#10801,.F.);
#15560=ORIENTED_EDGE('',*,*,#10341,.T.);
#15561=ORIENTED_EDGE('',*,*,#10802,.T.);
#15562=ORIENTED_EDGE('',*,*,#10659,.F.);
#15563=ORIENTED_EDGE('',*,*,#10803,.F.);
#15564=ORIENTED_EDGE('',*,*,#10344,.T.);
#15565=ORIENTED_EDGE('',*,*,#10804,.T.);
#15566=ORIENTED_EDGE('',*,*,#10656,.F.);
#15567=ORIENTED_EDGE('',*,*,#10805,.F.);
#15568=ORIENTED_EDGE('',*,*,#10347,.T.);
#15569=ORIENTED_EDGE('',*,*,#10806,.T.);
#15570=ORIENTED_EDGE('',*,*,#10653,.F.);
#15571=ORIENTED_EDGE('',*,*,#10807,.F.);
#15572=ORIENTED_EDGE('',*,*,#10350,.T.);
#15573=ORIENTED_EDGE('',*,*,#10808,.T.);
#15574=ORIENTED_EDGE('',*,*,#10650,.F.);
#15575=ORIENTED_EDGE('',*,*,#10809,.F.);
#15576=ORIENTED_EDGE('',*,*,#10353,.T.);
#15577=ORIENTED_EDGE('',*,*,#10810,.T.);
#15578=ORIENTED_EDGE('',*,*,#10647,.F.);
#15579=ORIENTED_EDGE('',*,*,#10811,.F.);
#15580=ORIENTED_EDGE('',*,*,#10356,.T.);
#15581=ORIENTED_EDGE('',*,*,#10812,.T.);
#15582=ORIENTED_EDGE('',*,*,#10644,.F.);
#15583=ORIENTED_EDGE('',*,*,#10813,.F.);
#15584=ORIENTED_EDGE('',*,*,#10359,.T.);
#15585=ORIENTED_EDGE('',*,*,#10814,.T.);
#15586=ORIENTED_EDGE('',*,*,#10641,.F.);
#15587=ORIENTED_EDGE('',*,*,#10815,.F.);
#15588=ORIENTED_EDGE('',*,*,#10362,.T.);
#15589=ORIENTED_EDGE('',*,*,#10816,.T.);
#15590=ORIENTED_EDGE('',*,*,#10638,.F.);
#15591=ORIENTED_EDGE('',*,*,#10817,.F.);
#15592=ORIENTED_EDGE('',*,*,#10365,.T.);
#15593=ORIENTED_EDGE('',*,*,#10818,.T.);
#15594=ORIENTED_EDGE('',*,*,#10635,.F.);
#15595=ORIENTED_EDGE('',*,*,#10819,.F.);
#15596=ORIENTED_EDGE('',*,*,#10368,.T.);
#15597=ORIENTED_EDGE('',*,*,#10820,.T.);
#15598=ORIENTED_EDGE('',*,*,#10632,.F.);
#15599=ORIENTED_EDGE('',*,*,#10821,.F.);
#15600=ORIENTED_EDGE('',*,*,#10371,.T.);
#15601=ORIENTED_EDGE('',*,*,#10822,.T.);
#15602=ORIENTED_EDGE('',*,*,#10629,.F.);
#15603=ORIENTED_EDGE('',*,*,#10823,.F.);
#15604=ORIENTED_EDGE('',*,*,#10374,.T.);
#15605=ORIENTED_EDGE('',*,*,#10824,.T.);
#15606=ORIENTED_EDGE('',*,*,#10626,.F.);
#15607=ORIENTED_EDGE('',*,*,#10825,.F.);
#15608=ORIENTED_EDGE('',*,*,#10377,.T.);
#15609=ORIENTED_EDGE('',*,*,#10826,.T.);
#15610=ORIENTED_EDGE('',*,*,#10623,.F.);
#15611=ORIENTED_EDGE('',*,*,#10827,.F.);
#15612=ORIENTED_EDGE('',*,*,#10380,.T.);
#15613=ORIENTED_EDGE('',*,*,#10828,.F.);
#15614=ORIENTED_EDGE('',*,*,#10386,.T.);
#15615=ORIENTED_EDGE('',*,*,#10829,.T.);
#15616=ORIENTED_EDGE('',*,*,#10617,.F.);
#15617=ORIENTED_EDGE('',*,*,#10560,.T.);
#15618=ORIENTED_EDGE('',*,*,#10830,.T.);
#15619=ORIENTED_EDGE('',*,*,#10620,.F.);
#15620=ORIENTED_EDGE('',*,*,#10831,.F.);
#15621=ORIENTED_EDGE('',*,*,#10383,.T.);
#15622=ORIENTED_EDGE('',*,*,#10326,.F.);
#15623=ORIENTED_EDGE('',*,*,#10085,.T.);
#15624=ORIENTED_EDGE('',*,*,#10207,.F.);
#15625=ORIENTED_EDGE('',*,*,#10676,.T.);
#15626=ORIENTED_EDGE('',*,*,#10091,.F.);
#15627=ORIENTED_EDGE('',*,*,#10619,.T.);
#15628=ORIENTED_EDGE('',*,*,#10832,.F.);
#15629=ORIENTED_EDGE('',*,*,#10384,.F.);
#15630=ORIENTED_EDGE('',*,*,#10831,.T.);
#15631=ORIENTED_EDGE('',*,*,#10618,.T.);
#15632=ORIENTED_EDGE('',*,*,#10829,.F.);
#15633=ORIENTED_EDGE('',*,*,#10385,.F.);
#15634=ORIENTED_EDGE('',*,*,#10832,.T.);
#15635=ORIENTED_EDGE('',*,*,#10616,.T.);
#15636=ORIENTED_EDGE('',*,*,#10833,.F.);
#15637=ORIENTED_EDGE('',*,*,#10387,.F.);
#15638=ORIENTED_EDGE('',*,*,#10828,.T.);
#15639=ORIENTED_EDGE('',*,*,#10615,.T.);
#15640=ORIENTED_EDGE('',*,*,#10679,.F.);
#15641=ORIENTED_EDGE('',*,*,#10388,.F.);
#15642=ORIENTED_EDGE('',*,*,#10833,.T.);
#15643=ORIENTED_EDGE('',*,*,#10622,.T.);
#15644=ORIENTED_EDGE('',*,*,#10834,.F.);
#15645=ORIENTED_EDGE('',*,*,#10381,.F.);
#15646=ORIENTED_EDGE('',*,*,#10827,.T.);
#15647=ORIENTED_EDGE('',*,*,#10621,.T.);
#15648=ORIENTED_EDGE('',*,*,#10830,.F.);
#15649=ORIENTED_EDGE('',*,*,#10382,.F.);
#15650=ORIENTED_EDGE('',*,*,#10834,.T.);
#15651=ORIENTED_EDGE('',*,*,#10625,.T.);
#15652=ORIENTED_EDGE('',*,*,#10835,.F.);
#15653=ORIENTED_EDGE('',*,*,#10378,.F.);
#15654=ORIENTED_EDGE('',*,*,#10825,.T.);
#15655=ORIENTED_EDGE('',*,*,#10624,.T.);
#15656=ORIENTED_EDGE('',*,*,#10826,.F.);
#15657=ORIENTED_EDGE('',*,*,#10379,.F.);
#15658=ORIENTED_EDGE('',*,*,#10835,.T.);
#15659=ORIENTED_EDGE('',*,*,#10628,.T.);
#15660=ORIENTED_EDGE('',*,*,#10836,.F.);
#15661=ORIENTED_EDGE('',*,*,#10375,.F.);
#15662=ORIENTED_EDGE('',*,*,#10823,.T.);
#15663=ORIENTED_EDGE('',*,*,#10627,.T.);
#15664=ORIENTED_EDGE('',*,*,#10824,.F.);
#15665=ORIENTED_EDGE('',*,*,#10376,.F.);
#15666=ORIENTED_EDGE('',*,*,#10836,.T.);
#15667=ORIENTED_EDGE('',*,*,#10631,.T.);
#15668=ORIENTED_EDGE('',*,*,#10837,.F.);
#15669=ORIENTED_EDGE('',*,*,#10372,.F.);
#15670=ORIENTED_EDGE('',*,*,#10821,.T.);
#15671=ORIENTED_EDGE('',*,*,#10630,.T.);
#15672=ORIENTED_EDGE('',*,*,#10822,.F.);
#15673=ORIENTED_EDGE('',*,*,#10373,.F.);
#15674=ORIENTED_EDGE('',*,*,#10837,.T.);
#15675=ORIENTED_EDGE('',*,*,#10634,.T.);
#15676=ORIENTED_EDGE('',*,*,#10838,.F.);
#15677=ORIENTED_EDGE('',*,*,#10369,.F.);
#15678=ORIENTED_EDGE('',*,*,#10819,.T.);
#15679=ORIENTED_EDGE('',*,*,#10633,.T.);
#15680=ORIENTED_EDGE('',*,*,#10820,.F.);
#15681=ORIENTED_EDGE('',*,*,#10370,.F.);
#15682=ORIENTED_EDGE('',*,*,#10838,.T.);
#15683=ORIENTED_EDGE('',*,*,#10637,.T.);
#15684=ORIENTED_EDGE('',*,*,#10839,.F.);
#15685=ORIENTED_EDGE('',*,*,#10366,.F.);
#15686=ORIENTED_EDGE('',*,*,#10817,.T.);
#15687=ORIENTED_EDGE('',*,*,#10636,.T.);
#15688=ORIENTED_EDGE('',*,*,#10818,.F.);
#15689=ORIENTED_EDGE('',*,*,#10367,.F.);
#15690=ORIENTED_EDGE('',*,*,#10839,.T.);
#15691=ORIENTED_EDGE('',*,*,#10640,.T.);
#15692=ORIENTED_EDGE('',*,*,#10840,.F.);
#15693=ORIENTED_EDGE('',*,*,#10363,.F.);
#15694=ORIENTED_EDGE('',*,*,#10815,.T.);
#15695=ORIENTED_EDGE('',*,*,#10639,.T.);
#15696=ORIENTED_EDGE('',*,*,#10816,.F.);
#15697=ORIENTED_EDGE('',*,*,#10364,.F.);
#15698=ORIENTED_EDGE('',*,*,#10840,.T.);
#15699=ORIENTED_EDGE('',*,*,#10643,.T.);
#15700=ORIENTED_EDGE('',*,*,#10841,.F.);
#15701=ORIENTED_EDGE('',*,*,#10360,.F.);
#15702=ORIENTED_EDGE('',*,*,#10813,.T.);
#15703=ORIENTED_EDGE('',*,*,#10642,.T.);
#15704=ORIENTED_EDGE('',*,*,#10814,.F.);
#15705=ORIENTED_EDGE('',*,*,#10361,.F.);
#15706=ORIENTED_EDGE('',*,*,#10841,.T.);
#15707=ORIENTED_EDGE('',*,*,#10646,.T.);
#15708=ORIENTED_EDGE('',*,*,#10842,.F.);
#15709=ORIENTED_EDGE('',*,*,#10357,.F.);
#15710=ORIENTED_EDGE('',*,*,#10811,.T.);
#15711=ORIENTED_EDGE('',*,*,#10645,.T.);
#15712=ORIENTED_EDGE('',*,*,#10812,.F.);
#15713=ORIENTED_EDGE('',*,*,#10358,.F.);
#15714=ORIENTED_EDGE('',*,*,#10842,.T.);
#15715=ORIENTED_EDGE('',*,*,#10649,.T.);
#15716=ORIENTED_EDGE('',*,*,#10843,.F.);
#15717=ORIENTED_EDGE('',*,*,#10354,.F.);
#15718=ORIENTED_EDGE('',*,*,#10809,.T.);
#15719=ORIENTED_EDGE('',*,*,#10648,.T.);
#15720=ORIENTED_EDGE('',*,*,#10810,.F.);
#15721=ORIENTED_EDGE('',*,*,#10355,.F.);
#15722=ORIENTED_EDGE('',*,*,#10843,.T.);
#15723=ORIENTED_EDGE('',*,*,#10652,.T.);
#15724=ORIENTED_EDGE('',*,*,#10844,.F.);
#15725=ORIENTED_EDGE('',*,*,#10351,.F.);
#15726=ORIENTED_EDGE('',*,*,#10807,.T.);
#15727=ORIENTED_EDGE('',*,*,#10651,.T.);
#15728=ORIENTED_EDGE('',*,*,#10808,.F.);
#15729=ORIENTED_EDGE('',*,*,#10352,.F.);
#15730=ORIENTED_EDGE('',*,*,#10844,.T.);
#15731=ORIENTED_EDGE('',*,*,#10655,.T.);
#15732=ORIENTED_EDGE('',*,*,#10845,.F.);
#15733=ORIENTED_EDGE('',*,*,#10348,.F.);
#15734=ORIENTED_EDGE('',*,*,#10805,.T.);
#15735=ORIENTED_EDGE('',*,*,#10654,.T.);
#15736=ORIENTED_EDGE('',*,*,#10806,.F.);
#15737=ORIENTED_EDGE('',*,*,#10349,.F.);
#15738=ORIENTED_EDGE('',*,*,#10845,.T.);
#15739=ORIENTED_EDGE('',*,*,#10658,.T.);
#15740=ORIENTED_EDGE('',*,*,#10846,.F.);
#15741=ORIENTED_EDGE('',*,*,#10345,.F.);
#15742=ORIENTED_EDGE('',*,*,#10803,.T.);
#15743=ORIENTED_EDGE('',*,*,#10657,.T.);
#15744=ORIENTED_EDGE('',*,*,#10804,.F.);
#15745=ORIENTED_EDGE('',*,*,#10346,.F.);
#15746=ORIENTED_EDGE('',*,*,#10846,.T.);
#15747=ORIENTED_EDGE('',*,*,#10661,.T.);
#15748=ORIENTED_EDGE('',*,*,#10847,.F.);
#15749=ORIENTED_EDGE('',*,*,#10342,.F.);
#15750=ORIENTED_EDGE('',*,*,#10801,.T.);
#15751=ORIENTED_EDGE('',*,*,#10660,.T.);
#15752=ORIENTED_EDGE('',*,*,#10802,.F.);
#15753=ORIENTED_EDGE('',*,*,#10343,.F.);
#15754=ORIENTED_EDGE('',*,*,#10847,.T.);
#15755=ORIENTED_EDGE('',*,*,#10664,.T.);
#15756=ORIENTED_EDGE('',*,*,#10848,.F.);
#15757=ORIENTED_EDGE('',*,*,#10339,.F.);
#15758=ORIENTED_EDGE('',*,*,#10799,.T.);
#15759=ORIENTED_EDGE('',*,*,#10663,.T.);
#15760=ORIENTED_EDGE('',*,*,#10800,.F.);
#15761=ORIENTED_EDGE('',*,*,#10340,.F.);
#15762=ORIENTED_EDGE('',*,*,#10848,.T.);
#15763=ORIENTED_EDGE('',*,*,#10667,.T.);
#15764=ORIENTED_EDGE('',*,*,#10849,.F.);
#15765=ORIENTED_EDGE('',*,*,#10336,.F.);
#15766=ORIENTED_EDGE('',*,*,#10797,.T.);
#15767=ORIENTED_EDGE('',*,*,#10666,.T.);
#15768=ORIENTED_EDGE('',*,*,#10798,.F.);
#15769=ORIENTED_EDGE('',*,*,#10337,.F.);
#15770=ORIENTED_EDGE('',*,*,#10849,.T.);
#15771=ORIENTED_EDGE('',*,*,#10670,.T.);
#15772=ORIENTED_EDGE('',*,*,#10850,.F.);
#15773=ORIENTED_EDGE('',*,*,#10333,.F.);
#15774=ORIENTED_EDGE('',*,*,#10795,.T.);
#15775=ORIENTED_EDGE('',*,*,#10669,.T.);
#15776=ORIENTED_EDGE('',*,*,#10796,.F.);
#15777=ORIENTED_EDGE('',*,*,#10334,.F.);
#15778=ORIENTED_EDGE('',*,*,#10850,.T.);
#15779=ORIENTED_EDGE('',*,*,#10673,.T.);
#15780=ORIENTED_EDGE('',*,*,#10851,.F.);
#15781=ORIENTED_EDGE('',*,*,#10330,.F.);
#15782=ORIENTED_EDGE('',*,*,#10793,.T.);
#15783=ORIENTED_EDGE('',*,*,#10672,.T.);
#15784=ORIENTED_EDGE('',*,*,#10794,.F.);
#15785=ORIENTED_EDGE('',*,*,#10331,.F.);
#15786=ORIENTED_EDGE('',*,*,#10851,.T.);
#15787=ORIENTED_EDGE('',*,*,#10442,.T.);
#15788=ORIENTED_EDGE('',*,*,#10852,.F.);
#15789=ORIENTED_EDGE('',*,*,#10327,.F.);
#15790=ORIENTED_EDGE('',*,*,#10324,.F.);
#15791=ORIENTED_EDGE('',*,*,#10791,.T.);
#15792=ORIENTED_EDGE('',*,*,#10675,.T.);
#15793=ORIENTED_EDGE('',*,*,#10792,.F.);
#15794=ORIENTED_EDGE('',*,*,#10328,.F.);
#15795=ORIENTED_EDGE('',*,*,#10852,.T.);
#15796=ORIENTED_EDGE('',*,*,#10445,.T.);
#15797=ORIENTED_EDGE('',*,*,#10853,.F.);
#15798=ORIENTED_EDGE('',*,*,#10321,.F.);
#15799=ORIENTED_EDGE('',*,*,#10789,.T.);
#15800=ORIENTED_EDGE('',*,*,#10444,.T.);
#15801=ORIENTED_EDGE('',*,*,#10790,.F.);
#15802=ORIENTED_EDGE('',*,*,#10322,.F.);
#15803=ORIENTED_EDGE('',*,*,#10853,.T.);
#15804=ORIENTED_EDGE('',*,*,#10448,.T.);
#15805=ORIENTED_EDGE('',*,*,#10854,.F.);
#15806=ORIENTED_EDGE('',*,*,#10318,.F.);
#15807=ORIENTED_EDGE('',*,*,#10787,.T.);
#15808=ORIENTED_EDGE('',*,*,#10447,.T.);
#15809=ORIENTED_EDGE('',*,*,#10788,.F.);
#15810=ORIENTED_EDGE('',*,*,#10319,.F.);
#15811=ORIENTED_EDGE('',*,*,#10854,.T.);
#15812=ORIENTED_EDGE('',*,*,#10451,.T.);
#15813=ORIENTED_EDGE('',*,*,#10855,.F.);
#15814=ORIENTED_EDGE('',*,*,#10315,.F.);
#15815=ORIENTED_EDGE('',*,*,#10785,.T.);
#15816=ORIENTED_EDGE('',*,*,#10450,.T.);
#15817=ORIENTED_EDGE('',*,*,#10786,.F.);
#15818=ORIENTED_EDGE('',*,*,#10316,.F.);
#15819=ORIENTED_EDGE('',*,*,#10855,.T.);
#15820=ORIENTED_EDGE('',*,*,#10454,.T.);
#15821=ORIENTED_EDGE('',*,*,#10856,.F.);
#15822=ORIENTED_EDGE('',*,*,#10312,.F.);
#15823=ORIENTED_EDGE('',*,*,#10783,.T.);
#15824=ORIENTED_EDGE('',*,*,#10453,.T.);
#15825=ORIENTED_EDGE('',*,*,#10784,.F.);
#15826=ORIENTED_EDGE('',*,*,#10313,.F.);
#15827=ORIENTED_EDGE('',*,*,#10856,.T.);
#15828=ORIENTED_EDGE('',*,*,#10457,.T.);
#15829=ORIENTED_EDGE('',*,*,#10857,.F.);
#15830=ORIENTED_EDGE('',*,*,#10309,.F.);
#15831=ORIENTED_EDGE('',*,*,#10781,.T.);
#15832=ORIENTED_EDGE('',*,*,#10456,.T.);
#15833=ORIENTED_EDGE('',*,*,#10782,.F.);
#15834=ORIENTED_EDGE('',*,*,#10310,.F.);
#15835=ORIENTED_EDGE('',*,*,#10857,.T.);
#15836=ORIENTED_EDGE('',*,*,#10460,.T.);
#15837=ORIENTED_EDGE('',*,*,#10858,.F.);
#15838=ORIENTED_EDGE('',*,*,#10306,.F.);
#15839=ORIENTED_EDGE('',*,*,#10779,.T.);
#15840=ORIENTED_EDGE('',*,*,#10459,.T.);
#15841=ORIENTED_EDGE('',*,*,#10780,.F.);
#15842=ORIENTED_EDGE('',*,*,#10307,.F.);
#15843=ORIENTED_EDGE('',*,*,#10858,.T.);
#15844=ORIENTED_EDGE('',*,*,#10463,.T.);
#15845=ORIENTED_EDGE('',*,*,#10859,.F.);
#15846=ORIENTED_EDGE('',*,*,#10303,.F.);
#15847=ORIENTED_EDGE('',*,*,#10777,.T.);
#15848=ORIENTED_EDGE('',*,*,#10462,.T.);
#15849=ORIENTED_EDGE('',*,*,#10778,.F.);
#15850=ORIENTED_EDGE('',*,*,#10304,.F.);
#15851=ORIENTED_EDGE('',*,*,#10859,.T.);
#15852=ORIENTED_EDGE('',*,*,#10466,.T.);
#15853=ORIENTED_EDGE('',*,*,#10860,.F.);
#15854=ORIENTED_EDGE('',*,*,#10300,.F.);
#15855=ORIENTED_EDGE('',*,*,#10775,.T.);
#15856=ORIENTED_EDGE('',*,*,#10465,.T.);
#15857=ORIENTED_EDGE('',*,*,#10776,.F.);
#15858=ORIENTED_EDGE('',*,*,#10301,.F.);
#15859=ORIENTED_EDGE('',*,*,#10860,.T.);
#15860=ORIENTED_EDGE('',*,*,#10469,.T.);
#15861=ORIENTED_EDGE('',*,*,#10861,.F.);
#15862=ORIENTED_EDGE('',*,*,#10297,.F.);
#15863=ORIENTED_EDGE('',*,*,#10773,.T.);
#15864=ORIENTED_EDGE('',*,*,#10468,.T.);
#15865=ORIENTED_EDGE('',*,*,#10774,.F.);
#15866=ORIENTED_EDGE('',*,*,#10298,.F.);
#15867=ORIENTED_EDGE('',*,*,#10861,.T.);
#15868=ORIENTED_EDGE('',*,*,#10472,.T.);
#15869=ORIENTED_EDGE('',*,*,#10862,.F.);
#15870=ORIENTED_EDGE('',*,*,#10294,.F.);
#15871=ORIENTED_EDGE('',*,*,#10771,.T.);
#15872=ORIENTED_EDGE('',*,*,#10471,.T.);
#15873=ORIENTED_EDGE('',*,*,#10772,.F.);
#15874=ORIENTED_EDGE('',*,*,#10295,.F.);
#15875=ORIENTED_EDGE('',*,*,#10862,.T.);
#15876=ORIENTED_EDGE('',*,*,#10475,.T.);
#15877=ORIENTED_EDGE('',*,*,#10863,.F.);
#15878=ORIENTED_EDGE('',*,*,#10291,.F.);
#15879=ORIENTED_EDGE('',*,*,#10769,.T.);
#15880=ORIENTED_EDGE('',*,*,#10474,.T.);
#15881=ORIENTED_EDGE('',*,*,#10770,.F.);
#15882=ORIENTED_EDGE('',*,*,#10292,.F.);
#15883=ORIENTED_EDGE('',*,*,#10863,.T.);
#15884=ORIENTED_EDGE('',*,*,#10478,.T.);
#15885=ORIENTED_EDGE('',*,*,#10864,.F.);
#15886=ORIENTED_EDGE('',*,*,#10288,.F.);
#15887=ORIENTED_EDGE('',*,*,#10767,.T.);
#15888=ORIENTED_EDGE('',*,*,#10477,.T.);
#15889=ORIENTED_EDGE('',*,*,#10768,.F.);
#15890=ORIENTED_EDGE('',*,*,#10289,.F.);
#15891=ORIENTED_EDGE('',*,*,#10864,.T.);
#15892=ORIENTED_EDGE('',*,*,#10481,.T.);
#15893=ORIENTED_EDGE('',*,*,#10865,.F.);
#15894=ORIENTED_EDGE('',*,*,#10285,.F.);
#15895=ORIENTED_EDGE('',*,*,#10765,.T.);
#15896=ORIENTED_EDGE('',*,*,#10480,.T.);
#15897=ORIENTED_EDGE('',*,*,#10766,.F.);
#15898=ORIENTED_EDGE('',*,*,#10286,.F.);
#15899=ORIENTED_EDGE('',*,*,#10865,.T.);
#15900=ORIENTED_EDGE('',*,*,#10484,.T.);
#15901=ORIENTED_EDGE('',*,*,#10866,.F.);
#15902=ORIENTED_EDGE('',*,*,#10282,.F.);
#15903=ORIENTED_EDGE('',*,*,#10763,.T.);
#15904=ORIENTED_EDGE('',*,*,#10483,.T.);
#15905=ORIENTED_EDGE('',*,*,#10764,.F.);
#15906=ORIENTED_EDGE('',*,*,#10283,.F.);
#15907=ORIENTED_EDGE('',*,*,#10866,.T.);
#15908=ORIENTED_EDGE('',*,*,#10487,.T.);
#15909=ORIENTED_EDGE('',*,*,#10867,.F.);
#15910=ORIENTED_EDGE('',*,*,#10279,.F.);
#15911=ORIENTED_EDGE('',*,*,#10761,.T.);
#15912=ORIENTED_EDGE('',*,*,#10486,.T.);
#15913=ORIENTED_EDGE('',*,*,#10762,.F.);
#15914=ORIENTED_EDGE('',*,*,#10280,.F.);
#15915=ORIENTED_EDGE('',*,*,#10867,.T.);
#15916=ORIENTED_EDGE('',*,*,#10490,.T.);
#15917=ORIENTED_EDGE('',*,*,#10868,.F.);
#15918=ORIENTED_EDGE('',*,*,#10276,.F.);
#15919=ORIENTED_EDGE('',*,*,#10759,.T.);
#15920=ORIENTED_EDGE('',*,*,#10489,.T.);
#15921=ORIENTED_EDGE('',*,*,#10760,.F.);
#15922=ORIENTED_EDGE('',*,*,#10277,.F.);
#15923=ORIENTED_EDGE('',*,*,#10868,.T.);
#15924=ORIENTED_EDGE('',*,*,#10493,.T.);
#15925=ORIENTED_EDGE('',*,*,#10869,.F.);
#15926=ORIENTED_EDGE('',*,*,#10273,.F.);
#15927=ORIENTED_EDGE('',*,*,#10757,.T.);
#15928=ORIENTED_EDGE('',*,*,#10492,.T.);
#15929=ORIENTED_EDGE('',*,*,#10758,.F.);
#15930=ORIENTED_EDGE('',*,*,#10274,.F.);
#15931=ORIENTED_EDGE('',*,*,#10869,.T.);
#15932=ORIENTED_EDGE('',*,*,#10496,.T.);
#15933=ORIENTED_EDGE('',*,*,#10870,.F.);
#15934=ORIENTED_EDGE('',*,*,#10270,.F.);
#15935=ORIENTED_EDGE('',*,*,#10755,.T.);
#15936=ORIENTED_EDGE('',*,*,#10495,.T.);
#15937=ORIENTED_EDGE('',*,*,#10756,.F.);
#15938=ORIENTED_EDGE('',*,*,#10271,.F.);
#15939=ORIENTED_EDGE('',*,*,#10870,.T.);
#15940=ORIENTED_EDGE('',*,*,#10499,.T.);
#15941=ORIENTED_EDGE('',*,*,#10871,.F.);
#15942=ORIENTED_EDGE('',*,*,#10267,.F.);
#15943=ORIENTED_EDGE('',*,*,#10753,.T.);
#15944=ORIENTED_EDGE('',*,*,#10498,.T.);
#15945=ORIENTED_EDGE('',*,*,#10754,.F.);
#15946=ORIENTED_EDGE('',*,*,#10268,.F.);
#15947=ORIENTED_EDGE('',*,*,#10871,.T.);
#15948=ORIENTED_EDGE('',*,*,#10502,.T.);
#15949=ORIENTED_EDGE('',*,*,#10872,.F.);
#15950=ORIENTED_EDGE('',*,*,#10264,.F.);
#15951=ORIENTED_EDGE('',*,*,#10751,.T.);
#15952=ORIENTED_EDGE('',*,*,#10501,.T.);
#15953=ORIENTED_EDGE('',*,*,#10752,.F.);
#15954=ORIENTED_EDGE('',*,*,#10265,.F.);
#15955=ORIENTED_EDGE('',*,*,#10872,.T.);
#15956=ORIENTED_EDGE('',*,*,#10505,.T.);
#15957=ORIENTED_EDGE('',*,*,#10873,.F.);
#15958=ORIENTED_EDGE('',*,*,#10261,.F.);
#15959=ORIENTED_EDGE('',*,*,#10749,.T.);
#15960=ORIENTED_EDGE('',*,*,#10504,.T.);
#15961=ORIENTED_EDGE('',*,*,#10750,.F.);
#15962=ORIENTED_EDGE('',*,*,#10262,.F.);
#15963=ORIENTED_EDGE('',*,*,#10873,.T.);
#15964=ORIENTED_EDGE('',*,*,#10508,.T.);
#15965=ORIENTED_EDGE('',*,*,#10874,.F.);
#15966=ORIENTED_EDGE('',*,*,#10258,.F.);
#15967=ORIENTED_EDGE('',*,*,#10747,.T.);
#15968=ORIENTED_EDGE('',*,*,#10507,.T.);
#15969=ORIENTED_EDGE('',*,*,#10748,.F.);
#15970=ORIENTED_EDGE('',*,*,#10259,.F.);
#15971=ORIENTED_EDGE('',*,*,#10874,.T.);
#15972=ORIENTED_EDGE('',*,*,#10511,.T.);
#15973=ORIENTED_EDGE('',*,*,#10875,.F.);
#15974=ORIENTED_EDGE('',*,*,#10255,.F.);
#15975=ORIENTED_EDGE('',*,*,#10745,.T.);
#15976=ORIENTED_EDGE('',*,*,#10510,.T.);
#15977=ORIENTED_EDGE('',*,*,#10746,.F.);
#15978=ORIENTED_EDGE('',*,*,#10256,.F.);
#15979=ORIENTED_EDGE('',*,*,#10875,.T.);
#15980=ORIENTED_EDGE('',*,*,#10514,.T.);
#15981=ORIENTED_EDGE('',*,*,#10876,.F.);
#15982=ORIENTED_EDGE('',*,*,#10252,.F.);
#15983=ORIENTED_EDGE('',*,*,#10743,.T.);
#15984=ORIENTED_EDGE('',*,*,#10513,.T.);
#15985=ORIENTED_EDGE('',*,*,#10744,.F.);
#15986=ORIENTED_EDGE('',*,*,#10253,.F.);
#15987=ORIENTED_EDGE('',*,*,#10876,.T.);
#15988=ORIENTED_EDGE('',*,*,#10517,.T.);
#15989=ORIENTED_EDGE('',*,*,#10877,.F.);
#15990=ORIENTED_EDGE('',*,*,#10249,.F.);
#15991=ORIENTED_EDGE('',*,*,#10741,.T.);
#15992=ORIENTED_EDGE('',*,*,#10516,.T.);
#15993=ORIENTED_EDGE('',*,*,#10742,.F.);
#15994=ORIENTED_EDGE('',*,*,#10250,.F.);
#15995=ORIENTED_EDGE('',*,*,#10877,.T.);
#15996=ORIENTED_EDGE('',*,*,#10520,.T.);
#15997=ORIENTED_EDGE('',*,*,#10878,.F.);
#15998=ORIENTED_EDGE('',*,*,#10246,.F.);
#15999=ORIENTED_EDGE('',*,*,#10739,.T.);
#16000=ORIENTED_EDGE('',*,*,#10519,.T.);
#16001=ORIENTED_EDGE('',*,*,#10740,.F.);
#16002=ORIENTED_EDGE('',*,*,#10247,.F.);
#16003=ORIENTED_EDGE('',*,*,#10878,.T.);
#16004=ORIENTED_EDGE('',*,*,#10523,.T.);
#16005=ORIENTED_EDGE('',*,*,#10879,.F.);
#16006=ORIENTED_EDGE('',*,*,#10243,.F.);
#16007=ORIENTED_EDGE('',*,*,#10737,.T.);
#16008=ORIENTED_EDGE('',*,*,#10522,.T.);
#16009=ORIENTED_EDGE('',*,*,#10738,.F.);
#16010=ORIENTED_EDGE('',*,*,#10244,.F.);
#16011=ORIENTED_EDGE('',*,*,#10879,.T.);
#16012=ORIENTED_EDGE('',*,*,#10526,.T.);
#16013=ORIENTED_EDGE('',*,*,#10880,.F.);
#16014=ORIENTED_EDGE('',*,*,#10240,.F.);
#16015=ORIENTED_EDGE('',*,*,#10735,.T.);
#16016=ORIENTED_EDGE('',*,*,#10525,.T.);
#16017=ORIENTED_EDGE('',*,*,#10736,.F.);
#16018=ORIENTED_EDGE('',*,*,#10241,.F.);
#16019=ORIENTED_EDGE('',*,*,#10880,.T.);
#16020=ORIENTED_EDGE('',*,*,#10529,.T.);
#16021=ORIENTED_EDGE('',*,*,#10881,.F.);
#16022=ORIENTED_EDGE('',*,*,#10237,.F.);
#16023=ORIENTED_EDGE('',*,*,#10733,.T.);
#16024=ORIENTED_EDGE('',*,*,#10528,.T.);
#16025=ORIENTED_EDGE('',*,*,#10734,.F.);
#16026=ORIENTED_EDGE('',*,*,#10238,.F.);
#16027=ORIENTED_EDGE('',*,*,#10881,.T.);
#16028=ORIENTED_EDGE('',*,*,#10532,.T.);
#16029=ORIENTED_EDGE('',*,*,#10882,.F.);
#16030=ORIENTED_EDGE('',*,*,#10234,.F.);
#16031=ORIENTED_EDGE('',*,*,#10731,.T.);
#16032=ORIENTED_EDGE('',*,*,#10531,.T.);
#16033=ORIENTED_EDGE('',*,*,#10732,.F.);
#16034=ORIENTED_EDGE('',*,*,#10235,.F.);
#16035=ORIENTED_EDGE('',*,*,#10882,.T.);
#16036=ORIENTED_EDGE('',*,*,#10535,.T.);
#16037=ORIENTED_EDGE('',*,*,#10883,.F.);
#16038=ORIENTED_EDGE('',*,*,#10231,.F.);
#16039=ORIENTED_EDGE('',*,*,#10729,.T.);
#16040=ORIENTED_EDGE('',*,*,#10534,.T.);
#16041=ORIENTED_EDGE('',*,*,#10730,.F.);
#16042=ORIENTED_EDGE('',*,*,#10232,.F.);
#16043=ORIENTED_EDGE('',*,*,#10883,.T.);
#16044=ORIENTED_EDGE('',*,*,#10538,.T.);
#16045=ORIENTED_EDGE('',*,*,#10884,.F.);
#16046=ORIENTED_EDGE('',*,*,#10228,.F.);
#16047=ORIENTED_EDGE('',*,*,#10727,.T.);
#16048=ORIENTED_EDGE('',*,*,#10537,.T.);
#16049=ORIENTED_EDGE('',*,*,#10728,.F.);
#16050=ORIENTED_EDGE('',*,*,#10229,.F.);
#16051=ORIENTED_EDGE('',*,*,#10884,.T.);
#16052=ORIENTED_EDGE('',*,*,#10541,.T.);
#16053=ORIENTED_EDGE('',*,*,#10885,.F.);
#16054=ORIENTED_EDGE('',*,*,#10225,.F.);
#16055=ORIENTED_EDGE('',*,*,#10725,.T.);
#16056=ORIENTED_EDGE('',*,*,#10540,.T.);
#16057=ORIENTED_EDGE('',*,*,#10726,.F.);
#16058=ORIENTED_EDGE('',*,*,#10226,.F.);
#16059=ORIENTED_EDGE('',*,*,#10885,.T.);
#16060=ORIENTED_EDGE('',*,*,#10544,.T.);
#16061=ORIENTED_EDGE('',*,*,#10886,.F.);
#16062=ORIENTED_EDGE('',*,*,#10222,.F.);
#16063=ORIENTED_EDGE('',*,*,#10723,.T.);
#16064=ORIENTED_EDGE('',*,*,#10543,.T.);
#16065=ORIENTED_EDGE('',*,*,#10724,.F.);
#16066=ORIENTED_EDGE('',*,*,#10223,.F.);
#16067=ORIENTED_EDGE('',*,*,#10886,.T.);
#16068=ORIENTED_EDGE('',*,*,#10547,.T.);
#16069=ORIENTED_EDGE('',*,*,#10887,.F.);
#16070=ORIENTED_EDGE('',*,*,#10219,.F.);
#16071=ORIENTED_EDGE('',*,*,#10721,.T.);
#16072=ORIENTED_EDGE('',*,*,#10546,.T.);
#16073=ORIENTED_EDGE('',*,*,#10722,.F.);
#16074=ORIENTED_EDGE('',*,*,#10220,.F.);
#16075=ORIENTED_EDGE('',*,*,#10887,.T.);
#16076=ORIENTED_EDGE('',*,*,#10550,.T.);
#16077=ORIENTED_EDGE('',*,*,#10888,.F.);
#16078=ORIENTED_EDGE('',*,*,#10216,.F.);
#16079=ORIENTED_EDGE('',*,*,#10719,.T.);
#16080=ORIENTED_EDGE('',*,*,#10549,.T.);
#16081=ORIENTED_EDGE('',*,*,#10720,.F.);
#16082=ORIENTED_EDGE('',*,*,#10217,.F.);
#16083=ORIENTED_EDGE('',*,*,#10888,.T.);
#16084=ORIENTED_EDGE('',*,*,#10553,.T.);
#16085=ORIENTED_EDGE('',*,*,#10889,.F.);
#16086=ORIENTED_EDGE('',*,*,#10213,.F.);
#16087=ORIENTED_EDGE('',*,*,#10717,.T.);
#16088=ORIENTED_EDGE('',*,*,#10552,.T.);
#16089=ORIENTED_EDGE('',*,*,#10718,.F.);
#16090=ORIENTED_EDGE('',*,*,#10214,.F.);
#16091=ORIENTED_EDGE('',*,*,#10889,.T.);
#16092=ORIENTED_EDGE('',*,*,#10556,.T.);
#16093=ORIENTED_EDGE('',*,*,#10890,.F.);
#16094=ORIENTED_EDGE('',*,*,#10210,.F.);
#16095=ORIENTED_EDGE('',*,*,#10715,.T.);
#16096=ORIENTED_EDGE('',*,*,#10555,.T.);
#16097=ORIENTED_EDGE('',*,*,#10716,.F.);
#16098=ORIENTED_EDGE('',*,*,#10211,.F.);
#16099=ORIENTED_EDGE('',*,*,#10890,.T.);
#16100=ORIENTED_EDGE('',*,*,#10562,.T.);
#16101=ORIENTED_EDGE('',*,*,#10891,.F.);
#16102=ORIENTED_EDGE('',*,*,#10441,.F.);
#16103=ORIENTED_EDGE('',*,*,#10713,.T.);
#16104=ORIENTED_EDGE('',*,*,#10561,.T.);
#16105=ORIENTED_EDGE('',*,*,#10558,.T.);
#16106=ORIENTED_EDGE('',*,*,#10714,.F.);
#16107=ORIENTED_EDGE('',*,*,#10208,.F.);
#16108=ORIENTED_EDGE('',*,*,#10891,.T.);
#16109=ORIENTED_EDGE('',*,*,#10565,.T.);
#16110=ORIENTED_EDGE('',*,*,#10892,.F.);
#16111=ORIENTED_EDGE('',*,*,#10438,.F.);
#16112=ORIENTED_EDGE('',*,*,#10711,.T.);
#16113=ORIENTED_EDGE('',*,*,#10564,.T.);
#16114=ORIENTED_EDGE('',*,*,#10712,.F.);
#16115=ORIENTED_EDGE('',*,*,#10439,.F.);
#16116=ORIENTED_EDGE('',*,*,#10892,.T.);
#16117=ORIENTED_EDGE('',*,*,#10568,.T.);
#16118=ORIENTED_EDGE('',*,*,#10893,.F.);
#16119=ORIENTED_EDGE('',*,*,#10435,.F.);
#16120=ORIENTED_EDGE('',*,*,#10709,.T.);
#16121=ORIENTED_EDGE('',*,*,#10567,.T.);
#16122=ORIENTED_EDGE('',*,*,#10710,.F.);
#16123=ORIENTED_EDGE('',*,*,#10436,.F.);
#16124=ORIENTED_EDGE('',*,*,#10893,.T.);
#16125=ORIENTED_EDGE('',*,*,#10571,.T.);
#16126=ORIENTED_EDGE('',*,*,#10894,.F.);
#16127=ORIENTED_EDGE('',*,*,#10432,.F.);
#16128=ORIENTED_EDGE('',*,*,#10707,.T.);
#16129=ORIENTED_EDGE('',*,*,#10570,.T.);
#16130=ORIENTED_EDGE('',*,*,#10708,.F.);
#16131=ORIENTED_EDGE('',*,*,#10433,.F.);
#16132=ORIENTED_EDGE('',*,*,#10894,.T.);
#16133=ORIENTED_EDGE('',*,*,#10574,.T.);
#16134=ORIENTED_EDGE('',*,*,#10895,.F.);
#16135=ORIENTED_EDGE('',*,*,#10429,.F.);
#16136=ORIENTED_EDGE('',*,*,#10705,.T.);
#16137=ORIENTED_EDGE('',*,*,#10573,.T.);
#16138=ORIENTED_EDGE('',*,*,#10706,.F.);
#16139=ORIENTED_EDGE('',*,*,#10430,.F.);
#16140=ORIENTED_EDGE('',*,*,#10895,.T.);
#16141=ORIENTED_EDGE('',*,*,#10577,.T.);
#16142=ORIENTED_EDGE('',*,*,#10896,.F.);
#16143=ORIENTED_EDGE('',*,*,#10426,.F.);
#16144=ORIENTED_EDGE('',*,*,#10703,.T.);
#16145=ORIENTED_EDGE('',*,*,#10576,.T.);
#16146=ORIENTED_EDGE('',*,*,#10704,.F.);
#16147=ORIENTED_EDGE('',*,*,#10427,.F.);
#16148=ORIENTED_EDGE('',*,*,#10896,.T.);
#16149=ORIENTED_EDGE('',*,*,#10580,.T.);
#16150=ORIENTED_EDGE('',*,*,#10897,.F.);
#16151=ORIENTED_EDGE('',*,*,#10423,.F.);
#16152=ORIENTED_EDGE('',*,*,#10701,.T.);
#16153=ORIENTED_EDGE('',*,*,#10579,.T.);
#16154=ORIENTED_EDGE('',*,*,#10702,.F.);
#16155=ORIENTED_EDGE('',*,*,#10424,.F.);
#16156=ORIENTED_EDGE('',*,*,#10897,.T.);
#16157=ORIENTED_EDGE('',*,*,#10583,.T.);
#16158=ORIENTED_EDGE('',*,*,#10898,.F.);
#16159=ORIENTED_EDGE('',*,*,#10420,.F.);
#16160=ORIENTED_EDGE('',*,*,#10699,.T.);
#16161=ORIENTED_EDGE('',*,*,#10582,.T.);
#16162=ORIENTED_EDGE('',*,*,#10700,.F.);
#16163=ORIENTED_EDGE('',*,*,#10421,.F.);
#16164=ORIENTED_EDGE('',*,*,#10898,.T.);
#16165=ORIENTED_EDGE('',*,*,#10586,.T.);
#16166=ORIENTED_EDGE('',*,*,#10899,.F.);
#16167=ORIENTED_EDGE('',*,*,#10417,.F.);
#16168=ORIENTED_EDGE('',*,*,#10697,.T.);
#16169=ORIENTED_EDGE('',*,*,#10585,.T.);
#16170=ORIENTED_EDGE('',*,*,#10698,.F.);
#16171=ORIENTED_EDGE('',*,*,#10418,.F.);
#16172=ORIENTED_EDGE('',*,*,#10899,.T.);
#16173=ORIENTED_EDGE('',*,*,#10589,.T.);
#16174=ORIENTED_EDGE('',*,*,#10900,.F.);
#16175=ORIENTED_EDGE('',*,*,#10414,.F.);
#16176=ORIENTED_EDGE('',*,*,#10695,.T.);
#16177=ORIENTED_EDGE('',*,*,#10588,.T.);
#16178=ORIENTED_EDGE('',*,*,#10696,.F.);
#16179=ORIENTED_EDGE('',*,*,#10415,.F.);
#16180=ORIENTED_EDGE('',*,*,#10900,.T.);
#16181=ORIENTED_EDGE('',*,*,#10592,.T.);
#16182=ORIENTED_EDGE('',*,*,#10901,.F.);
#16183=ORIENTED_EDGE('',*,*,#10411,.F.);
#16184=ORIENTED_EDGE('',*,*,#10693,.T.);
#16185=ORIENTED_EDGE('',*,*,#10591,.T.);
#16186=ORIENTED_EDGE('',*,*,#10694,.F.);
#16187=ORIENTED_EDGE('',*,*,#10412,.F.);
#16188=ORIENTED_EDGE('',*,*,#10901,.T.);
#16189=ORIENTED_EDGE('',*,*,#10595,.T.);
#16190=ORIENTED_EDGE('',*,*,#10902,.F.);
#16191=ORIENTED_EDGE('',*,*,#10408,.F.);
#16192=ORIENTED_EDGE('',*,*,#10691,.T.);
#16193=ORIENTED_EDGE('',*,*,#10594,.T.);
#16194=ORIENTED_EDGE('',*,*,#10692,.F.);
#16195=ORIENTED_EDGE('',*,*,#10409,.F.);
#16196=ORIENTED_EDGE('',*,*,#10902,.T.);
#16197=ORIENTED_EDGE('',*,*,#10598,.T.);
#16198=ORIENTED_EDGE('',*,*,#10903,.F.);
#16199=ORIENTED_EDGE('',*,*,#10405,.F.);
#16200=ORIENTED_EDGE('',*,*,#10689,.T.);
#16201=ORIENTED_EDGE('',*,*,#10597,.T.);
#16202=ORIENTED_EDGE('',*,*,#10690,.F.);
#16203=ORIENTED_EDGE('',*,*,#10406,.F.);
#16204=ORIENTED_EDGE('',*,*,#10903,.T.);
#16205=ORIENTED_EDGE('',*,*,#10601,.T.);
#16206=ORIENTED_EDGE('',*,*,#10904,.F.);
#16207=ORIENTED_EDGE('',*,*,#10402,.F.);
#16208=ORIENTED_EDGE('',*,*,#10687,.T.);
#16209=ORIENTED_EDGE('',*,*,#10600,.T.);
#16210=ORIENTED_EDGE('',*,*,#10688,.F.);
#16211=ORIENTED_EDGE('',*,*,#10403,.F.);
#16212=ORIENTED_EDGE('',*,*,#10904,.T.);
#16213=ORIENTED_EDGE('',*,*,#10604,.T.);
#16214=ORIENTED_EDGE('',*,*,#10905,.F.);
#16215=ORIENTED_EDGE('',*,*,#10399,.F.);
#16216=ORIENTED_EDGE('',*,*,#10685,.T.);
#16217=ORIENTED_EDGE('',*,*,#10603,.T.);
#16218=ORIENTED_EDGE('',*,*,#10686,.F.);
#16219=ORIENTED_EDGE('',*,*,#10400,.F.);
#16220=ORIENTED_EDGE('',*,*,#10905,.T.);
#16221=ORIENTED_EDGE('',*,*,#10607,.T.);
#16222=ORIENTED_EDGE('',*,*,#10906,.F.);
#16223=ORIENTED_EDGE('',*,*,#10396,.F.);
#16224=ORIENTED_EDGE('',*,*,#10683,.T.);
#16225=ORIENTED_EDGE('',*,*,#10606,.T.);
#16226=ORIENTED_EDGE('',*,*,#10684,.F.);
#16227=ORIENTED_EDGE('',*,*,#10397,.F.);
#16228=ORIENTED_EDGE('',*,*,#10906,.T.);
#16229=ORIENTED_EDGE('',*,*,#10610,.T.);
#16230=ORIENTED_EDGE('',*,*,#10907,.F.);
#16231=ORIENTED_EDGE('',*,*,#10393,.F.);
#16232=ORIENTED_EDGE('',*,*,#10681,.T.);
#16233=ORIENTED_EDGE('',*,*,#10609,.T.);
#16234=ORIENTED_EDGE('',*,*,#10682,.F.);
#16235=ORIENTED_EDGE('',*,*,#10394,.F.);
#16236=ORIENTED_EDGE('',*,*,#10907,.T.);
#16237=ORIENTED_EDGE('',*,*,#10613,.T.);
#16238=ORIENTED_EDGE('',*,*,#10908,.F.);
#16239=ORIENTED_EDGE('',*,*,#10390,.F.);
#16240=ORIENTED_EDGE('',*,*,#10678,.T.);
#16241=ORIENTED_EDGE('',*,*,#10612,.T.);
#16242=ORIENTED_EDGE('',*,*,#10680,.F.);
#16243=ORIENTED_EDGE('',*,*,#10391,.F.);
#16244=ORIENTED_EDGE('',*,*,#10908,.T.);
#16375=CYLINDRICAL_SURFACE('',#18482,2.);
#16376=CYLINDRICAL_SURFACE('',#18485,2.);
#16377=CYLINDRICAL_SURFACE('',#18487,1.2);
#16378=CYLINDRICAL_SURFACE('',#18488,3.2);
#16379=CYLINDRICAL_SURFACE('',#18489,2.);
#16380=CYLINDRICAL_SURFACE('',#18490,1.5);
#16381=CYLINDRICAL_SURFACE('',#18506,4.);
#16382=CYLINDRICAL_SURFACE('',#18511,4.);
#16383=CYLINDRICAL_SURFACE('',#18525,3.);
#16384=CYLINDRICAL_SURFACE('',#18530,3.);
#16385=CYLINDRICAL_SURFACE('',#18532,0.300000000000002);
#16386=CYLINDRICAL_SURFACE('',#18535,0.3);
#16387=CYLINDRICAL_SURFACE('',#18537,0.300000000000002);
#16388=CYLINDRICAL_SURFACE('',#18540,0.300000000000002);
#16389=CYLINDRICAL_SURFACE('',#18542,0.300000000000002);
#16390=CYLINDRICAL_SURFACE('',#18550,0.3);
#16391=CYLINDRICAL_SURFACE('',#18552,0.300000000000002);
#16392=CYLINDRICAL_SURFACE('',#18555,0.300000000000002);
#16393=CYLINDRICAL_SURFACE('',#18557,0.300000000000002);
#16394=CYLINDRICAL_SURFACE('',#18559,0.300000000000002);
#16395=CYLINDRICAL_SURFACE('',#18561,0.300000000000002);
#16396=CYLINDRICAL_SURFACE('',#18569,0.300000000000002);
#16397=CYLINDRICAL_SURFACE('',#18571,0.300000000000002);
#16398=CYLINDRICAL_SURFACE('',#18573,0.300000000000002);
#16399=CYLINDRICAL_SURFACE('',#18575,0.300000000000002);
#16400=CYLINDRICAL_SURFACE('',#18579,0.300000000000002);
#16401=CYLINDRICAL_SURFACE('',#18582,0.300000000000002);
#16402=CYLINDRICAL_SURFACE('',#18584,0.300000000000002);
#16403=CYLINDRICAL_SURFACE('',#18586,0.300000000000002);
#16404=CYLINDRICAL_SURFACE('',#18588,0.300000000000002);
#16405=CYLINDRICAL_SURFACE('',#18590,0.300000000000002);
#16406=CYLINDRICAL_SURFACE('',#18607,1.2);
#16407=CYLINDRICAL_SURFACE('',#18610,2.5);
#16408=CYLINDRICAL_SURFACE('',#18613,3.);
#16409=CYLINDRICAL_SURFACE('',#18618,4.25);
#16410=CYLINDRICAL_SURFACE('',#18621,1.2);
#16411=CYLINDRICAL_SURFACE('',#18624,1.2);
#16412=CYLINDRICAL_SURFACE('',#18627,2.);
#16413=CYLINDRICAL_SURFACE('',#18631,1.5);
#16414=CYLINDRICAL_SURFACE('',#18640,1.5);
#16415=CYLINDRICAL_SURFACE('',#18650,2.5);
#16416=CYLINDRICAL_SURFACE('',#18670,2.);
#16417=CYLINDRICAL_SURFACE('',#18679,2.);
#16418=CYLINDRICAL_SURFACE('',#18688,2.);
#16419=CYLINDRICAL_SURFACE('',#18697,2.);
#16420=CYLINDRICAL_SURFACE('',#18706,2.);
#16421=CYLINDRICAL_SURFACE('',#18715,2.);
#16422=CYLINDRICAL_SURFACE('',#18724,2.);
#16423=CYLINDRICAL_SURFACE('',#18733,2.);
#16424=CYLINDRICAL_SURFACE('',#18742,2.);
#16425=CYLINDRICAL_SURFACE('',#18751,2.);
#16426=CYLINDRICAL_SURFACE('',#18760,2.);
#16427=CYLINDRICAL_SURFACE('',#18769,2.);
#16428=CYLINDRICAL_SURFACE('',#18778,2.);
#16429=CYLINDRICAL_SURFACE('',#18787,2.);
#16430=CYLINDRICAL_SURFACE('',#18954,2.);
#16431=CYLINDRICAL_SURFACE('',#18955,8.175);
#16432=CYLINDRICAL_SURFACE('',#18956,8.175);
#16433=CYLINDRICAL_SURFACE('',#18957,8.175);
#16434=CYLINDRICAL_SURFACE('',#18958,8.175);
#16435=CYLINDRICAL_SURFACE('',#18959,8.175);
#16436=CYLINDRICAL_SURFACE('',#18960,8.175);
#16437=CYLINDRICAL_SURFACE('',#18961,8.175);
#16438=CYLINDRICAL_SURFACE('',#18962,8.175);
#16439=CYLINDRICAL_SURFACE('',#18963,8.175);
#16440=CYLINDRICAL_SURFACE('',#18964,8.175);
#16441=CYLINDRICAL_SURFACE('',#18965,8.175);
#16442=CYLINDRICAL_SURFACE('',#18966,8.175);
#16443=CYLINDRICAL_SURFACE('',#18967,8.175);
#16444=CYLINDRICAL_SURFACE('',#18968,8.175);
#16445=CYLINDRICAL_SURFACE('',#18969,8.175);
#16446=CYLINDRICAL_SURFACE('',#18970,8.175);
#16447=CYLINDRICAL_SURFACE('',#18971,8.175);
#16448=CYLINDRICAL_SURFACE('',#18972,8.175);
#16449=CYLINDRICAL_SURFACE('',#18973,8.175);
#16450=CYLINDRICAL_SURFACE('',#18974,8.175);
#16451=CYLINDRICAL_SURFACE('',#18975,8.175);
#16452=CYLINDRICAL_SURFACE('',#18976,8.175);
#16453=CYLINDRICAL_SURFACE('',#18977,8.175);
#16454=CYLINDRICAL_SURFACE('',#18978,8.175);
#16455=CYLINDRICAL_SURFACE('',#18979,8.175);
#16456=CYLINDRICAL_SURFACE('',#18980,8.175);
#16457=CYLINDRICAL_SURFACE('',#18981,8.175);
#16458=CYLINDRICAL_SURFACE('',#18982,8.175);
#16459=CYLINDRICAL_SURFACE('',#18983,8.175);
#16460=CYLINDRICAL_SURFACE('',#18984,8.175);
#16461=CYLINDRICAL_SURFACE('',#18985,8.175);
#16462=CYLINDRICAL_SURFACE('',#18986,8.175);
#16463=CYLINDRICAL_SURFACE('',#18987,8.175);
#16464=CYLINDRICAL_SURFACE('',#18988,8.175);
#16465=CYLINDRICAL_SURFACE('',#18989,8.175);
#16466=CYLINDRICAL_SURFACE('',#18990,8.175);
#16467=CYLINDRICAL_SURFACE('',#18991,8.175);
#16468=CYLINDRICAL_SURFACE('',#18992,8.175);
#16469=CYLINDRICAL_SURFACE('',#18993,8.175);
#16470=CYLINDRICAL_SURFACE('',#18994,8.175);
#16471=CYLINDRICAL_SURFACE('',#18995,8.175);
#16472=CYLINDRICAL_SURFACE('',#18996,8.175);
#16473=CYLINDRICAL_SURFACE('',#18997,8.175);
#16474=CYLINDRICAL_SURFACE('',#18998,8.175);
#16475=CYLINDRICAL_SURFACE('',#18999,8.175);
#16476=CYLINDRICAL_SURFACE('',#19000,8.175);
#16477=CYLINDRICAL_SURFACE('',#19001,8.175);
#16478=CYLINDRICAL_SURFACE('',#19002,8.175);
#16479=CYLINDRICAL_SURFACE('',#19003,8.175);
#16480=CYLINDRICAL_SURFACE('',#19004,8.175);
#16481=CYLINDRICAL_SURFACE('',#19005,8.175);
#16482=CYLINDRICAL_SURFACE('',#19006,8.175);
#16483=CYLINDRICAL_SURFACE('',#19007,8.175);
#16484=CYLINDRICAL_SURFACE('',#19008,8.175);
#16485=CYLINDRICAL_SURFACE('',#19009,8.175);
#16486=CYLINDRICAL_SURFACE('',#19010,8.175);
#16487=CYLINDRICAL_SURFACE('',#19011,8.175);
#16488=CYLINDRICAL_SURFACE('',#19012,8.175);
#16489=CYLINDRICAL_SURFACE('',#19013,8.175);
#16490=CYLINDRICAL_SURFACE('',#19014,8.175);
#16491=CYLINDRICAL_SURFACE('',#19015,8.175);
#16492=CYLINDRICAL_SURFACE('',#19016,8.175);
#16493=CYLINDRICAL_SURFACE('',#19017,8.175);
#16494=CYLINDRICAL_SURFACE('',#19018,8.175);
#16495=CYLINDRICAL_SURFACE('',#19019,8.175);
#16496=CYLINDRICAL_SURFACE('',#19020,8.175);
#16497=CYLINDRICAL_SURFACE('',#19021,8.175);
#16498=CYLINDRICAL_SURFACE('',#19022,8.175);
#16499=CYLINDRICAL_SURFACE('',#19023,8.175);
#16500=CYLINDRICAL_SURFACE('',#19024,8.175);
#16501=CYLINDRICAL_SURFACE('',#19025,8.175);
#16502=CYLINDRICAL_SURFACE('',#19026,8.175);
#16503=CYLINDRICAL_SURFACE('',#19027,8.175);
#16504=CYLINDRICAL_SURFACE('',#19028,8.175);
#16505=CYLINDRICAL_SURFACE('',#19029,8.175);
#16506=CYLINDRICAL_SURFACE('',#19030,8.175);
#16507=CYLINDRICAL_SURFACE('',#19032,8.175);
#16508=CYLINDRICAL_SURFACE('',#19200,1.5);
#16509=CYLINDRICAL_SURFACE('',#19224,2.);
#16510=CYLINDRICAL_SURFACE('',#19233,2.);
#16511=CYLINDRICAL_SURFACE('',#19242,2.);
#16512=CYLINDRICAL_SURFACE('',#19251,2.);
#16513=CYLINDRICAL_SURFACE('',#19260,2.);
#16514=CYLINDRICAL_SURFACE('',#19269,2.);
#16515=CYLINDRICAL_SURFACE('',#19278,2.);
#16516=CYLINDRICAL_SURFACE('',#19287,2.);
#16517=CYLINDRICAL_SURFACE('',#19296,2.);
#16518=CYLINDRICAL_SURFACE('',#19305,2.);
#16519=CYLINDRICAL_SURFACE('',#19314,2.);
#16520=CYLINDRICAL_SURFACE('',#19323,2.);
#16521=CYLINDRICAL_SURFACE('',#19332,4.);
#16522=CYLINDRICAL_SURFACE('',#19492,2.);
#16523=CYLINDRICAL_SURFACE('',#19494,8.175);
#16524=CYLINDRICAL_SURFACE('',#19495,8.175);
#16525=CYLINDRICAL_SURFACE('',#19496,8.175);
#16526=CYLINDRICAL_SURFACE('',#19497,8.175);
#16527=CYLINDRICAL_SURFACE('',#19498,8.175);
#16528=CYLINDRICAL_SURFACE('',#19499,8.175);
#16529=CYLINDRICAL_SURFACE('',#19500,8.175);
#16530=CYLINDRICAL_SURFACE('',#19501,8.175);
#16531=CYLINDRICAL_SURFACE('',#19502,8.175);
#16532=CYLINDRICAL_SURFACE('',#19503,8.175);
#16533=CYLINDRICAL_SURFACE('',#19504,8.175);
#16534=CYLINDRICAL_SURFACE('',#19505,8.175);
#16535=CYLINDRICAL_SURFACE('',#19506,8.175);
#16536=CYLINDRICAL_SURFACE('',#19507,8.175);
#16537=CYLINDRICAL_SURFACE('',#19508,8.175);
#16538=CYLINDRICAL_SURFACE('',#19509,8.175);
#16539=CYLINDRICAL_SURFACE('',#19510,8.175);
#16540=CYLINDRICAL_SURFACE('',#19511,8.175);
#16541=CYLINDRICAL_SURFACE('',#19512,8.175);
#16542=CYLINDRICAL_SURFACE('',#19513,8.175);
#16543=CYLINDRICAL_SURFACE('',#19514,8.175);
#16544=CYLINDRICAL_SURFACE('',#19515,8.175);
#16545=CYLINDRICAL_SURFACE('',#19516,8.175);
#16546=CYLINDRICAL_SURFACE('',#19517,8.175);
#16547=CYLINDRICAL_SURFACE('',#19518,8.175);
#16548=CYLINDRICAL_SURFACE('',#19519,8.175);
#16549=CYLINDRICAL_SURFACE('',#19520,8.175);
#16550=CYLINDRICAL_SURFACE('',#19521,8.175);
#16551=CYLINDRICAL_SURFACE('',#19522,8.175);
#16552=CYLINDRICAL_SURFACE('',#19523,8.175);
#16553=CYLINDRICAL_SURFACE('',#19524,8.175);
#16554=CYLINDRICAL_SURFACE('',#19525,8.175);
#16555=CYLINDRICAL_SURFACE('',#19526,8.175);
#16556=CYLINDRICAL_SURFACE('',#19527,8.175);
#16557=CYLINDRICAL_SURFACE('',#19528,8.175);
#16558=CYLINDRICAL_SURFACE('',#19529,8.175);
#16559=CYLINDRICAL_SURFACE('',#19530,8.175);
#16560=CYLINDRICAL_SURFACE('',#19531,8.175);
#16561=CYLINDRICAL_SURFACE('',#19532,8.175);
#16562=CYLINDRICAL_SURFACE('',#19533,8.175);
#16563=CYLINDRICAL_SURFACE('',#19534,8.175);
#16564=CYLINDRICAL_SURFACE('',#19535,8.175);
#16565=CYLINDRICAL_SURFACE('',#19536,8.175);
#16566=CYLINDRICAL_SURFACE('',#19537,8.175);
#16567=CYLINDRICAL_SURFACE('',#19538,8.175);
#16568=CYLINDRICAL_SURFACE('',#19539,8.175);
#16569=CYLINDRICAL_SURFACE('',#19540,8.175);
#16570=CYLINDRICAL_SURFACE('',#19541,8.175);
#16571=CYLINDRICAL_SURFACE('',#19542,8.175);
#16572=CYLINDRICAL_SURFACE('',#19543,8.175);
#16573=CYLINDRICAL_SURFACE('',#19544,8.175);
#16574=CYLINDRICAL_SURFACE('',#19545,8.175);
#16575=CYLINDRICAL_SURFACE('',#19546,8.175);
#16576=CYLINDRICAL_SURFACE('',#19547,8.175);
#16577=CYLINDRICAL_SURFACE('',#19548,8.175);
#16578=CYLINDRICAL_SURFACE('',#19549,8.175);
#16579=CYLINDRICAL_SURFACE('',#19550,8.175);
#16580=CYLINDRICAL_SURFACE('',#19551,8.175);
#16581=CYLINDRICAL_SURFACE('',#19552,8.175);
#16582=CYLINDRICAL_SURFACE('',#19553,8.175);
#16583=CYLINDRICAL_SURFACE('',#19554,8.175);
#16584=CYLINDRICAL_SURFACE('',#19555,8.175);
#16585=CYLINDRICAL_SURFACE('',#19556,8.175);
#16586=CYLINDRICAL_SURFACE('',#19557,8.175);
#16587=CYLINDRICAL_SURFACE('',#19558,8.175);
#16588=CYLINDRICAL_SURFACE('',#19559,8.175);
#16589=CYLINDRICAL_SURFACE('',#19560,8.175);
#16590=CYLINDRICAL_SURFACE('',#19561,8.175);
#16591=CYLINDRICAL_SURFACE('',#19562,8.175);
#16592=CYLINDRICAL_SURFACE('',#19563,8.175);
#16593=CYLINDRICAL_SURFACE('',#19564,8.175);
#16594=CYLINDRICAL_SURFACE('',#19565,8.175);
#16595=CYLINDRICAL_SURFACE('',#19566,8.175);
#16596=CYLINDRICAL_SURFACE('',#19567,8.175);
#16597=CYLINDRICAL_SURFACE('',#19568,8.175);
#16598=CYLINDRICAL_SURFACE('',#19569,8.175);
#16599=CYLINDRICAL_SURFACE('',#19571,8.175);
#16928=ADVANCED_FACE('',(#1969),#1035,.F.);
#16929=ADVANCED_FACE('',(#1970),#1036,.F.);
#16930=ADVANCED_FACE('',(#1971),#1037,.F.);
#16931=ADVANCED_FACE('',(#1972),#1038,.F.);
#16932=ADVANCED_FACE('',(#1973),#1039,.F.);
#16933=ADVANCED_FACE('',(#1974),#1040,.F.);
#16934=ADVANCED_FACE('',(#1975),#1041,.F.);
#16935=ADVANCED_FACE('',(#1976),#1042,.F.);
#16936=ADVANCED_FACE('',(#1977),#1043,.F.);
#16937=ADVANCED_FACE('',(#1978),#1044,.F.);
#16938=ADVANCED_FACE('',(#1979),#16375,.F.);
#16939=ADVANCED_FACE('',(#1980),#16376,.F.);
#16940=ADVANCED_FACE('',(#1981),#16377,.F.);
#16941=ADVANCED_FACE('',(#1982),#16378,.F.);
#16942=ADVANCED_FACE('',(#1983),#16379,.F.);
#16943=ADVANCED_FACE('',(#1984),#16380,.F.);
#16944=ADVANCED_FACE('',(#1985),#1279,.F.);
#16945=ADVANCED_FACE('',(#1986),#1280,.F.);
#16946=ADVANCED_FACE('',(#1987,#885,#886),#1281,.F.);
#16947=ADVANCED_FACE('',(#1988),#1282,.F.);
#16948=ADVANCED_FACE('',(#1989),#1283,.F.);
#16949=ADVANCED_FACE('',(#1990),#1284,.F.);
#16950=ADVANCED_FACE('',(#1991,#887,#888),#1285,.F.);
#16951=ADVANCED_FACE('',(#1992,#889),#1286,.F.);
#16952=ADVANCED_FACE('',(#1993,#890),#1287,.T.);
#16953=ADVANCED_FACE('',(#1994),#16381,.F.);
#16954=ADVANCED_FACE('',(#1995),#1288,.F.);
#16955=ADVANCED_FACE('',(#1996,#891),#1289,.F.);
#16956=ADVANCED_FACE('',(#1997),#16382,.F.);
#16957=ADVANCED_FACE('',(#1998),#1290,.F.);
#16958=ADVANCED_FACE('',(#1999),#1291,.F.);
#16959=ADVANCED_FACE('',(#2000),#1292,.F.);
#16960=ADVANCED_FACE('',(#2001),#1293,.F.);
#16961=ADVANCED_FACE('',(#2002),#1294,.F.);
#16962=ADVANCED_FACE('',(#2003),#1295,.F.);
#16963=ADVANCED_FACE('',(#2004,#892),#1296,.F.);
#16964=ADVANCED_FACE('',(#2005),#1297,.F.);
#16965=ADVANCED_FACE('',(#2006),#1298,.F.);
#16966=ADVANCED_FACE('',(#2007),#1299,.F.);
#16967=ADVANCED_FACE('',(#2008),#16383,.F.);
#16968=ADVANCED_FACE('',(#2009,#893),#1300,.F.);
#16969=ADVANCED_FACE('',(#2010),#1301,.F.);
#16970=ADVANCED_FACE('',(#2011),#16384,.F.);
#16971=ADVANCED_FACE('',(#2012),#16385,.T.);
#16972=ADVANCED_FACE('',(#2013),#16386,.T.);
#16973=ADVANCED_FACE('',(#2014),#16387,.T.);
#16974=ADVANCED_FACE('',(#2015),#16388,.T.);
#16975=ADVANCED_FACE('',(#2016),#16389,.T.);
#16976=ADVANCED_FACE('',(#2017),#179,.T.);
#16977=ADVANCED_FACE('',(#2018),#117,.T.);
#16978=ADVANCED_FACE('',(#2019),#16390,.T.);
#16979=ADVANCED_FACE('',(#2020),#16391,.T.);
#16980=ADVANCED_FACE('',(#2021),#16392,.T.);
#16981=ADVANCED_FACE('',(#2022),#16393,.T.);
#16982=ADVANCED_FACE('',(#2023),#16394,.T.);
#16983=ADVANCED_FACE('',(#2024),#16395,.T.);
#16984=ADVANCED_FACE('',(#2025),#180,.T.);
#16985=ADVANCED_FACE('',(#2026),#118,.T.);
#16986=ADVANCED_FACE('',(#2027),#119,.T.);
#16987=ADVANCED_FACE('',(#2028),#16396,.T.);
#16988=ADVANCED_FACE('',(#2029),#16397,.T.);
#16989=ADVANCED_FACE('',(#2030),#16398,.T.);
#16990=ADVANCED_FACE('',(#2031),#16399,.T.);
#16991=ADVANCED_FACE('',(#2032),#120,.T.);
#16992=ADVANCED_FACE('',(#2033),#16400,.T.);
#16993=ADVANCED_FACE('',(#2034),#121,.T.);
#16994=ADVANCED_FACE('',(#2035),#16401,.T.);
#16995=ADVANCED_FACE('',(#2036),#16402,.T.);
#16996=ADVANCED_FACE('',(#2037),#16403,.T.);
#16997=ADVANCED_FACE('',(#2038),#16404,.T.);
#16998=ADVANCED_FACE('',(#2039),#16405,.T.);
#16999=ADVANCED_FACE('',(#2040),#122,.T.);
#17000=ADVANCED_FACE('',(#2041),#1045,.F.);
#17001=ADVANCED_FACE('',(#2042),#1046,.F.);
#17002=ADVANCED_FACE('',(#2043),#1047,.F.);
#17003=ADVANCED_FACE('',(#2044),#1048,.F.);
#17004=ADVANCED_FACE('',(#2045),#181,.T.);
#17005=ADVANCED_FACE('',(#2046),#182,.T.);
#17006=ADVANCED_FACE('',(#2047),#16406,.T.);
#17007=ADVANCED_FACE('',(#2048),#1302,.T.);
#17008=ADVANCED_FACE('',(#2049),#1303,.F.);
#17009=ADVANCED_FACE('',(#2050),#16407,.T.);
#17010=ADVANCED_FACE('',(#2051),#16408,.T.);
#17011=ADVANCED_FACE('',(#2052),#16409,.F.);
#17012=ADVANCED_FACE('',(#2053),#16410,.F.);
#17013=ADVANCED_FACE('',(#2054),#16411,.F.);
#17014=ADVANCED_FACE('',(#2055),#16412,.F.);
#17015=ADVANCED_FACE('',(#2056),#1304,.F.);
#17016=ADVANCED_FACE('',(#2057),#16413,.T.);
#17017=ADVANCED_FACE('',(#2058),#1305,.F.);
#17018=ADVANCED_FACE('',(#2059,#894),#1306,.F.);
#17019=ADVANCED_FACE('',(#2060,#895),#1307,.T.);
#17020=ADVANCED_FACE('',(#2061),#1308,.F.);
#17021=ADVANCED_FACE('',(#2062,#896),#1309,.F.);
#17022=ADVANCED_FACE('',(#2063),#16414,.T.);
#17023=ADVANCED_FACE('',(#2064),#1310,.F.);
#17024=ADVANCED_FACE('',(#2065,#897),#1311,.F.);
#17025=ADVANCED_FACE('',(#2066,#898),#1312,.F.);
#17026=ADVANCED_FACE('',(#2067,#899),#1313,.F.);
#17027=ADVANCED_FACE('',(#2068),#1314,.F.);
#17028=ADVANCED_FACE('',(#2069,#900),#1315,.T.);
#17029=ADVANCED_FACE('',(#2070,#901),#1316,.T.);
#17030=ADVANCED_FACE('',(#2071),#1317,.T.);
#17031=ADVANCED_FACE('',(#2072),#16415,.F.);
#17032=ADVANCED_FACE('',(#2073,#902),#123,.T.);
#17033=ADVANCED_FACE('',(#2074),#1318,.T.);
#17034=ADVANCED_FACE('',(#2075),#183,.F.);
#17035=ADVANCED_FACE('',(#2076),#1049,.T.);
#17036=ADVANCED_FACE('',(#2077),#1050,.T.);
#17037=ADVANCED_FACE('',(#2078),#1051,.T.);
#17038=ADVANCED_FACE('',(#2079),#16416,.T.);
#17039=ADVANCED_FACE('',(#2080),#1052,.T.);
#17040=ADVANCED_FACE('',(#2081),#1053,.T.);
#17041=ADVANCED_FACE('',(#2082),#16417,.T.);
#17042=ADVANCED_FACE('',(#2083),#1054,.T.);
#17043=ADVANCED_FACE('',(#2084),#1055,.T.);
#17044=ADVANCED_FACE('',(#2085),#16418,.T.);
#17045=ADVANCED_FACE('',(#2086),#1056,.T.);
#17046=ADVANCED_FACE('',(#2087),#1057,.T.);
#17047=ADVANCED_FACE('',(#2088),#16419,.T.);
#17048=ADVANCED_FACE('',(#2089),#1058,.T.);
#17049=ADVANCED_FACE('',(#2090),#1059,.T.);
#17050=ADVANCED_FACE('',(#2091),#16420,.T.);
#17051=ADVANCED_FACE('',(#2092),#1060,.T.);
#17052=ADVANCED_FACE('',(#2093),#1061,.T.);
#17053=ADVANCED_FACE('',(#2094),#16421,.T.);
#17054=ADVANCED_FACE('',(#2095),#1062,.T.);
#17055=ADVANCED_FACE('',(#2096),#1063,.T.);
#17056=ADVANCED_FACE('',(#2097),#16422,.T.);
#17057=ADVANCED_FACE('',(#2098),#1064,.T.);
#17058=ADVANCED_FACE('',(#2099),#1065,.T.);
#17059=ADVANCED_FACE('',(#2100),#16423,.T.);
#17060=ADVANCED_FACE('',(#2101),#1066,.T.);
#17061=ADVANCED_FACE('',(#2102),#1067,.T.);
#17062=ADVANCED_FACE('',(#2103),#16424,.T.);
#17063=ADVANCED_FACE('',(#2104),#1068,.T.);
#17064=ADVANCED_FACE('',(#2105),#1069,.T.);
#17065=ADVANCED_FACE('',(#2106),#16425,.T.);
#17066=ADVANCED_FACE('',(#2107),#1070,.T.);
#17067=ADVANCED_FACE('',(#2108),#1071,.T.);
#17068=ADVANCED_FACE('',(#2109),#16426,.T.);
#17069=ADVANCED_FACE('',(#2110),#1072,.T.);
#17070=ADVANCED_FACE('',(#2111),#1073,.T.);
#17071=ADVANCED_FACE('',(#2112),#16427,.T.);
#17072=ADVANCED_FACE('',(#2113),#1074,.T.);
#17073=ADVANCED_FACE('',(#2114),#1075,.T.);
#17074=ADVANCED_FACE('',(#2115),#16428,.T.);
#17075=ADVANCED_FACE('',(#2116),#1076,.T.);
#17076=ADVANCED_FACE('',(#2117),#1077,.T.);
#17077=ADVANCED_FACE('',(#2118),#16429,.T.);
#17078=ADVANCED_FACE('',(#2119),#1078,.T.);
#17079=ADVANCED_FACE('',(#2120),#1079,.T.);
#17080=ADVANCED_FACE('',(#2121),#1080,.T.);
#17081=ADVANCED_FACE('',(#2122),#1081,.T.);
#17082=ADVANCED_FACE('',(#2123),#16430,.T.);
#17083=ADVANCED_FACE('',(#2124),#16431,.T.);
#17084=ADVANCED_FACE('',(#2125),#16432,.T.);
#17085=ADVANCED_FACE('',(#2126),#16433,.T.);
#17086=ADVANCED_FACE('',(#2127),#16434,.T.);
#17087=ADVANCED_FACE('',(#2128),#16435,.T.);
#17088=ADVANCED_FACE('',(#2129),#16436,.T.);
#17089=ADVANCED_FACE('',(#2130),#16437,.T.);
#17090=ADVANCED_FACE('',(#2131),#16438,.T.);
#17091=ADVANCED_FACE('',(#2132),#16439,.T.);
#17092=ADVANCED_FACE('',(#2133),#16440,.T.);
#17093=ADVANCED_FACE('',(#2134),#16441,.T.);
#17094=ADVANCED_FACE('',(#2135),#16442,.T.);
#17095=ADVANCED_FACE('',(#2136),#16443,.T.);
#17096=ADVANCED_FACE('',(#2137),#16444,.T.);
#17097=ADVANCED_FACE('',(#2138),#16445,.T.);
#17098=ADVANCED_FACE('',(#2139),#16446,.T.);
#17099=ADVANCED_FACE('',(#2140),#16447,.T.);
#17100=ADVANCED_FACE('',(#2141),#16448,.T.);
#17101=ADVANCED_FACE('',(#2142),#16449,.T.);
#17102=ADVANCED_FACE('',(#2143),#16450,.T.);
#17103=ADVANCED_FACE('',(#2144),#16451,.T.);
#17104=ADVANCED_FACE('',(#2145),#16452,.T.);
#17105=ADVANCED_FACE('',(#2146),#16453,.T.);
#17106=ADVANCED_FACE('',(#2147),#16454,.T.);
#17107=ADVANCED_FACE('',(#2148),#16455,.T.);
#17108=ADVANCED_FACE('',(#2149),#16456,.T.);
#17109=ADVANCED_FACE('',(#2150),#16457,.T.);
#17110=ADVANCED_FACE('',(#2151),#16458,.T.);
#17111=ADVANCED_FACE('',(#2152),#16459,.T.);
#17112=ADVANCED_FACE('',(#2153),#16460,.T.);
#17113=ADVANCED_FACE('',(#2154),#16461,.T.);
#17114=ADVANCED_FACE('',(#2155),#16462,.T.);
#17115=ADVANCED_FACE('',(#2156),#16463,.T.);
#17116=ADVANCED_FACE('',(#2157),#16464,.T.);
#17117=ADVANCED_FACE('',(#2158),#16465,.T.);
#17118=ADVANCED_FACE('',(#2159),#16466,.T.);
#17119=ADVANCED_FACE('',(#2160),#16467,.T.);
#17120=ADVANCED_FACE('',(#2161),#16468,.T.);
#17121=ADVANCED_FACE('',(#2162),#16469,.T.);
#17122=ADVANCED_FACE('',(#2163),#16470,.T.);
#17123=ADVANCED_FACE('',(#2164),#16471,.T.);
#17124=ADVANCED_FACE('',(#2165),#16472,.T.);
#17125=ADVANCED_FACE('',(#2166),#16473,.T.);
#17126=ADVANCED_FACE('',(#2167),#16474,.T.);
#17127=ADVANCED_FACE('',(#2168),#16475,.T.);
#17128=ADVANCED_FACE('',(#2169),#16476,.T.);
#17129=ADVANCED_FACE('',(#2170),#16477,.T.);
#17130=ADVANCED_FACE('',(#2171),#16478,.T.);
#17131=ADVANCED_FACE('',(#2172),#16479,.T.);
#17132=ADVANCED_FACE('',(#2173),#16480,.T.);
#17133=ADVANCED_FACE('',(#2174),#16481,.T.);
#17134=ADVANCED_FACE('',(#2175),#16482,.T.);
#17135=ADVANCED_FACE('',(#2176),#16483,.T.);
#17136=ADVANCED_FACE('',(#2177),#16484,.T.);
#17137=ADVANCED_FACE('',(#2178),#16485,.T.);
#17138=ADVANCED_FACE('',(#2179),#16486,.T.);
#17139=ADVANCED_FACE('',(#2180),#16487,.T.);
#17140=ADVANCED_FACE('',(#2181),#16488,.T.);
#17141=ADVANCED_FACE('',(#2182),#16489,.T.);
#17142=ADVANCED_FACE('',(#2183),#16490,.T.);
#17143=ADVANCED_FACE('',(#2184),#16491,.T.);
#17144=ADVANCED_FACE('',(#2185),#16492,.T.);
#17145=ADVANCED_FACE('',(#2186),#16493,.T.);
#17146=ADVANCED_FACE('',(#2187),#16494,.T.);
#17147=ADVANCED_FACE('',(#2188),#16495,.T.);
#17148=ADVANCED_FACE('',(#2189),#16496,.T.);
#17149=ADVANCED_FACE('',(#2190),#16497,.T.);
#17150=ADVANCED_FACE('',(#2191),#16498,.T.);
#17151=ADVANCED_FACE('',(#2192),#16499,.T.);
#17152=ADVANCED_FACE('',(#2193),#16500,.T.);
#17153=ADVANCED_FACE('',(#2194),#16501,.T.);
#17154=ADVANCED_FACE('',(#2195),#16502,.T.);
#17155=ADVANCED_FACE('',(#2196),#16503,.T.);
#17156=ADVANCED_FACE('',(#2197),#16504,.T.);
#17157=ADVANCED_FACE('',(#2198),#16505,.T.);
#17158=ADVANCED_FACE('',(#2199),#16506,.T.);
#17159=ADVANCED_FACE('',(#2200,#903),#1319,.F.);
#17160=ADVANCED_FACE('',(#2201),#16507,.T.);
#17161=ADVANCED_FACE('',(#2202),#1320,.T.);
#17162=ADVANCED_FACE('',(#2203),#1321,.T.);
#17163=ADVANCED_FACE('',(#2204),#1322,.F.);
#17164=ADVANCED_FACE('',(#2205),#1323,.F.);
#17165=ADVANCED_FACE('',(#2206),#1324,.F.);
#17166=ADVANCED_FACE('',(#2207),#1325,.F.);
#17167=ADVANCED_FACE('',(#2208),#1326,.F.);
#17168=ADVANCED_FACE('',(#2209),#1327,.F.);
#17169=ADVANCED_FACE('',(#2210),#1328,.F.);
#17170=ADVANCED_FACE('',(#2211),#1329,.F.);
#17171=ADVANCED_FACE('',(#2212),#1330,.F.);
#17172=ADVANCED_FACE('',(#2213),#1331,.F.);
#17173=ADVANCED_FACE('',(#2214),#1332,.F.);
#17174=ADVANCED_FACE('',(#2215),#1333,.F.);
#17175=ADVANCED_FACE('',(#2216),#1334,.F.);
#17176=ADVANCED_FACE('',(#2217),#1335,.F.);
#17177=ADVANCED_FACE('',(#2218),#1336,.F.);
#17178=ADVANCED_FACE('',(#2219),#1337,.F.);
#17179=ADVANCED_FACE('',(#2220),#1338,.F.);
#17180=ADVANCED_FACE('',(#2221),#1339,.F.);
#17181=ADVANCED_FACE('',(#2222),#1340,.F.);
#17182=ADVANCED_FACE('',(#2223),#1341,.F.);
#17183=ADVANCED_FACE('',(#2224),#1342,.F.);
#17184=ADVANCED_FACE('',(#2225),#1343,.F.);
#17185=ADVANCED_FACE('',(#2226),#1344,.F.);
#17186=ADVANCED_FACE('',(#2227),#1345,.F.);
#17187=ADVANCED_FACE('',(#2228),#1346,.F.);
#17188=ADVANCED_FACE('',(#2229),#1347,.F.);
#17189=ADVANCED_FACE('',(#2230),#1348,.F.);
#17190=ADVANCED_FACE('',(#2231),#1349,.F.);
#17191=ADVANCED_FACE('',(#2232),#1350,.F.);
#17192=ADVANCED_FACE('',(#2233),#1351,.F.);
#17193=ADVANCED_FACE('',(#2234),#1352,.F.);
#17194=ADVANCED_FACE('',(#2235),#1353,.F.);
#17195=ADVANCED_FACE('',(#2236),#1354,.F.);
#17196=ADVANCED_FACE('',(#2237),#1355,.F.);
#17197=ADVANCED_FACE('',(#2238),#1356,.F.);
#17198=ADVANCED_FACE('',(#2239),#1357,.F.);
#17199=ADVANCED_FACE('',(#2240),#1358,.F.);
#17200=ADVANCED_FACE('',(#2241),#1359,.F.);
#17201=ADVANCED_FACE('',(#2242),#1360,.F.);
#17202=ADVANCED_FACE('',(#2243),#1361,.F.);
#17203=ADVANCED_FACE('',(#2244),#1362,.F.);
#17204=ADVANCED_FACE('',(#2245),#1363,.F.);
#17205=ADVANCED_FACE('',(#2246),#1364,.F.);
#17206=ADVANCED_FACE('',(#2247),#1365,.F.);
#17207=ADVANCED_FACE('',(#2248),#1366,.F.);
#17208=ADVANCED_FACE('',(#2249),#1367,.F.);
#17209=ADVANCED_FACE('',(#2250),#1368,.F.);
#17210=ADVANCED_FACE('',(#2251),#1369,.F.);
#17211=ADVANCED_FACE('',(#2252),#1370,.F.);
#17212=ADVANCED_FACE('',(#2253),#1371,.F.);
#17213=ADVANCED_FACE('',(#2254),#1372,.F.);
#17214=ADVANCED_FACE('',(#2255),#1373,.F.);
#17215=ADVANCED_FACE('',(#2256),#1374,.F.);
#17216=ADVANCED_FACE('',(#2257),#1375,.F.);
#17217=ADVANCED_FACE('',(#2258),#1376,.F.);
#17218=ADVANCED_FACE('',(#2259),#1377,.F.);
#17219=ADVANCED_FACE('',(#2260),#1378,.F.);
#17220=ADVANCED_FACE('',(#2261),#1379,.F.);
#17221=ADVANCED_FACE('',(#2262),#1380,.F.);
#17222=ADVANCED_FACE('',(#2263),#1381,.F.);
#17223=ADVANCED_FACE('',(#2264),#1382,.F.);
#17224=ADVANCED_FACE('',(#2265),#1383,.F.);
#17225=ADVANCED_FACE('',(#2266),#1384,.F.);
#17226=ADVANCED_FACE('',(#2267),#1385,.F.);
#17227=ADVANCED_FACE('',(#2268),#1386,.F.);
#17228=ADVANCED_FACE('',(#2269),#1387,.F.);
#17229=ADVANCED_FACE('',(#2270),#1388,.F.);
#17230=ADVANCED_FACE('',(#2271),#1389,.F.);
#17231=ADVANCED_FACE('',(#2272),#1390,.F.);
#17232=ADVANCED_FACE('',(#2273),#1391,.F.);
#17233=ADVANCED_FACE('',(#2274),#1392,.F.);
#17234=ADVANCED_FACE('',(#2275),#1393,.F.);
#17235=ADVANCED_FACE('',(#2276),#1394,.F.);
#17236=ADVANCED_FACE('',(#2277),#1395,.F.);
#17237=ADVANCED_FACE('',(#2278),#1396,.F.);
#17238=ADVANCED_FACE('',(#2279),#1397,.F.);
#17239=ADVANCED_FACE('',(#2280),#1398,.F.);
#17240=ADVANCED_FACE('',(#2281),#1399,.F.);
#17241=ADVANCED_FACE('',(#2282),#1400,.F.);
#17242=ADVANCED_FACE('',(#2283),#1401,.F.);
#17243=ADVANCED_FACE('',(#2284),#1402,.F.);
#17244=ADVANCED_FACE('',(#2285),#1403,.F.);
#17245=ADVANCED_FACE('',(#2286),#1404,.F.);
#17246=ADVANCED_FACE('',(#2287),#1405,.F.);
#17247=ADVANCED_FACE('',(#2288),#1406,.F.);
#17248=ADVANCED_FACE('',(#2289),#1407,.F.);
#17249=ADVANCED_FACE('',(#2290),#1408,.F.);
#17250=ADVANCED_FACE('',(#2291),#1409,.F.);
#17251=ADVANCED_FACE('',(#2292),#1410,.F.);
#17252=ADVANCED_FACE('',(#2293),#1411,.F.);
#17253=ADVANCED_FACE('',(#2294),#1412,.F.);
#17254=ADVANCED_FACE('',(#2295),#1413,.F.);
#17255=ADVANCED_FACE('',(#2296),#1414,.F.);
#17256=ADVANCED_FACE('',(#2297),#1415,.F.);
#17257=ADVANCED_FACE('',(#2298),#1416,.F.);
#17258=ADVANCED_FACE('',(#2299),#1417,.F.);
#17259=ADVANCED_FACE('',(#2300),#1418,.F.);
#17260=ADVANCED_FACE('',(#2301),#1419,.F.);
#17261=ADVANCED_FACE('',(#2302),#1420,.F.);
#17262=ADVANCED_FACE('',(#2303),#1421,.F.);
#17263=ADVANCED_FACE('',(#2304),#1422,.F.);
#17264=ADVANCED_FACE('',(#2305),#1423,.F.);
#17265=ADVANCED_FACE('',(#2306),#1424,.F.);
#17266=ADVANCED_FACE('',(#2307),#1425,.F.);
#17267=ADVANCED_FACE('',(#2308),#1426,.F.);
#17268=ADVANCED_FACE('',(#2309),#1427,.F.);
#17269=ADVANCED_FACE('',(#2310),#1428,.F.);
#17270=ADVANCED_FACE('',(#2311),#1429,.F.);
#17271=ADVANCED_FACE('',(#2312),#1430,.F.);
#17272=ADVANCED_FACE('',(#2313),#1431,.F.);
#17273=ADVANCED_FACE('',(#2314),#1432,.F.);
#17274=ADVANCED_FACE('',(#2315),#1433,.F.);
#17275=ADVANCED_FACE('',(#2316),#1434,.F.);
#17276=ADVANCED_FACE('',(#2317),#1435,.F.);
#17277=ADVANCED_FACE('',(#2318),#1436,.F.);
#17278=ADVANCED_FACE('',(#2319),#1437,.F.);
#17279=ADVANCED_FACE('',(#2320),#1438,.F.);
#17280=ADVANCED_FACE('',(#2321),#1439,.F.);
#17281=ADVANCED_FACE('',(#2322),#1440,.F.);
#17282=ADVANCED_FACE('',(#2323),#1441,.F.);
#17283=ADVANCED_FACE('',(#2324),#1442,.F.);
#17284=ADVANCED_FACE('',(#2325),#1443,.F.);
#17285=ADVANCED_FACE('',(#2326),#1444,.F.);
#17286=ADVANCED_FACE('',(#2327),#1445,.F.);
#17287=ADVANCED_FACE('',(#2328),#1446,.F.);
#17288=ADVANCED_FACE('',(#2329),#1447,.F.);
#17289=ADVANCED_FACE('',(#2330),#1448,.F.);
#17290=ADVANCED_FACE('',(#2331),#1449,.F.);
#17291=ADVANCED_FACE('',(#2332),#1450,.F.);
#17292=ADVANCED_FACE('',(#2333),#1451,.F.);
#17293=ADVANCED_FACE('',(#2334),#1452,.F.);
#17294=ADVANCED_FACE('',(#2335),#1453,.F.);
#17295=ADVANCED_FACE('',(#2336),#1454,.F.);
#17296=ADVANCED_FACE('',(#2337),#1455,.F.);
#17297=ADVANCED_FACE('',(#2338),#1456,.F.);
#17298=ADVANCED_FACE('',(#2339),#1457,.F.);
#17299=ADVANCED_FACE('',(#2340),#1458,.F.);
#17300=ADVANCED_FACE('',(#2341),#1459,.F.);
#17301=ADVANCED_FACE('',(#2342),#1460,.F.);
#17302=ADVANCED_FACE('',(#2343),#1461,.F.);
#17303=ADVANCED_FACE('',(#2344),#1462,.F.);
#17304=ADVANCED_FACE('',(#2345),#1463,.F.);
#17305=ADVANCED_FACE('',(#2346),#1464,.F.);
#17306=ADVANCED_FACE('',(#2347),#1465,.F.);
#17307=ADVANCED_FACE('',(#2348),#1466,.F.);
#17308=ADVANCED_FACE('',(#2349),#1467,.F.);
#17309=ADVANCED_FACE('',(#2350),#1468,.F.);
#17310=ADVANCED_FACE('',(#2351),#1469,.F.);
#17311=ADVANCED_FACE('',(#2352),#1470,.F.);
#17312=ADVANCED_FACE('',(#2353),#1471,.F.);
#17313=ADVANCED_FACE('',(#2354),#1472,.F.);
#17314=ADVANCED_FACE('',(#2355),#1473,.F.);
#17315=ADVANCED_FACE('',(#2356),#1474,.F.);
#17316=ADVANCED_FACE('',(#2357),#1475,.F.);
#17317=ADVANCED_FACE('',(#2358),#184,.T.);
#17318=ADVANCED_FACE('',(#2359),#1082,.T.);
#17319=ADVANCED_FACE('',(#2360),#16508,.T.);
#17320=ADVANCED_FACE('',(#2361),#1476,.T.);
#17321=ADVANCED_FACE('',(#2362),#1477,.T.);
#17322=ADVANCED_FACE('',(#2363),#1478,.T.);
#17323=ADVANCED_FACE('',(#2364,#904),#1479,.F.);
#17324=ADVANCED_FACE('',(#2365),#1480,.F.);
#17325=ADVANCED_FACE('',(#2366),#1481,.F.);
#17326=ADVANCED_FACE('',(#2367),#1482,.T.);
#17327=ADVANCED_FACE('',(#2368),#185,.F.);
#17328=ADVANCED_FACE('',(#2369),#1083,.T.);
#17329=ADVANCED_FACE('',(#2370),#1084,.T.);
#17330=ADVANCED_FACE('',(#2371),#1085,.T.);
#17331=ADVANCED_FACE('',(#2372),#16509,.T.);
#17332=ADVANCED_FACE('',(#2373),#1086,.T.);
#17333=ADVANCED_FACE('',(#2374),#1087,.T.);
#17334=ADVANCED_FACE('',(#2375),#16510,.T.);
#17335=ADVANCED_FACE('',(#2376),#1088,.T.);
#17336=ADVANCED_FACE('',(#2377),#1089,.T.);
#17337=ADVANCED_FACE('',(#2378),#16511,.T.);
#17338=ADVANCED_FACE('',(#2379),#1090,.T.);
#17339=ADVANCED_FACE('',(#2380),#1091,.T.);
#17340=ADVANCED_FACE('',(#2381),#16512,.T.);
#17341=ADVANCED_FACE('',(#2382),#1092,.T.);
#17342=ADVANCED_FACE('',(#2383),#1093,.T.);
#17343=ADVANCED_FACE('',(#2384),#16513,.T.);
#17344=ADVANCED_FACE('',(#2385),#1094,.T.);
#17345=ADVANCED_FACE('',(#2386),#1095,.T.);
#17346=ADVANCED_FACE('',(#2387),#16514,.T.);
#17347=ADVANCED_FACE('',(#2388),#1096,.T.);
#17348=ADVANCED_FACE('',(#2389),#1097,.T.);
#17349=ADVANCED_FACE('',(#2390),#16515,.T.);
#17350=ADVANCED_FACE('',(#2391),#1098,.T.);
#17351=ADVANCED_FACE('',(#2392),#1099,.T.);
#17352=ADVANCED_FACE('',(#2393),#16516,.T.);
#17353=ADVANCED_FACE('',(#2394),#1100,.T.);
#17354=ADVANCED_FACE('',(#2395),#1101,.T.);
#17355=ADVANCED_FACE('',(#2396),#16517,.T.);
#17356=ADVANCED_FACE('',(#2397),#1102,.T.);
#17357=ADVANCED_FACE('',(#2398),#1103,.T.);
#17358=ADVANCED_FACE('',(#2399),#16518,.T.);
#17359=ADVANCED_FACE('',(#2400),#1104,.T.);
#17360=ADVANCED_FACE('',(#2401),#1105,.T.);
#17361=ADVANCED_FACE('',(#2402),#16519,.T.);
#17362=ADVANCED_FACE('',(#2403),#1106,.T.);
#17363=ADVANCED_FACE('',(#2404),#1107,.T.);
#17364=ADVANCED_FACE('',(#2405),#16520,.T.);
#17365=ADVANCED_FACE('',(#2406),#1108,.T.);
#17366=ADVANCED_FACE('',(#2407),#1109,.T.);
#17367=ADVANCED_FACE('',(#2408),#16521,.T.);
#17368=ADVANCED_FACE('',(#2409),#1110,.T.);
#17369=ADVANCED_FACE('',(#2410),#1111,.T.);
#17370=ADVANCED_FACE('',(#2411),#16522,.T.);
#17371=ADVANCED_FACE('',(#2412),#16523,.T.);
#17372=ADVANCED_FACE('',(#2413),#16524,.T.);
#17373=ADVANCED_FACE('',(#2414),#16525,.T.);
#17374=ADVANCED_FACE('',(#2415),#16526,.T.);
#17375=ADVANCED_FACE('',(#2416),#16527,.T.);
#17376=ADVANCED_FACE('',(#2417),#16528,.T.);
#17377=ADVANCED_FACE('',(#2418),#16529,.T.);
#17378=ADVANCED_FACE('',(#2419),#16530,.T.);
#17379=ADVANCED_FACE('',(#2420),#16531,.T.);
#17380=ADVANCED_FACE('',(#2421),#16532,.T.);
#17381=ADVANCED_FACE('',(#2422),#16533,.T.);
#17382=ADVANCED_FACE('',(#2423),#16534,.T.);
#17383=ADVANCED_FACE('',(#2424),#16535,.T.);
#17384=ADVANCED_FACE('',(#2425),#16536,.T.);
#17385=ADVANCED_FACE('',(#2426),#16537,.T.);
#17386=ADVANCED_FACE('',(#2427),#16538,.T.);
#17387=ADVANCED_FACE('',(#2428),#16539,.T.);
#17388=ADVANCED_FACE('',(#2429),#16540,.T.);
#17389=ADVANCED_FACE('',(#2430),#16541,.T.);
#17390=ADVANCED_FACE('',(#2431),#16542,.T.);
#17391=ADVANCED_FACE('',(#2432),#16543,.T.);
#17392=ADVANCED_FACE('',(#2433),#16544,.T.);
#17393=ADVANCED_FACE('',(#2434),#16545,.T.);
#17394=ADVANCED_FACE('',(#2435),#16546,.T.);
#17395=ADVANCED_FACE('',(#2436),#16547,.T.);
#17396=ADVANCED_FACE('',(#2437),#16548,.T.);
#17397=ADVANCED_FACE('',(#2438),#16549,.T.);
#17398=ADVANCED_FACE('',(#2439),#16550,.T.);
#17399=ADVANCED_FACE('',(#2440),#16551,.T.);
#17400=ADVANCED_FACE('',(#2441),#16552,.T.);
#17401=ADVANCED_FACE('',(#2442),#16553,.T.);
#17402=ADVANCED_FACE('',(#2443),#16554,.T.);
#17403=ADVANCED_FACE('',(#2444),#16555,.T.);
#17404=ADVANCED_FACE('',(#2445),#16556,.T.);
#17405=ADVANCED_FACE('',(#2446),#16557,.T.);
#17406=ADVANCED_FACE('',(#2447),#16558,.T.);
#17407=ADVANCED_FACE('',(#2448),#16559,.T.);
#17408=ADVANCED_FACE('',(#2449),#16560,.T.);
#17409=ADVANCED_FACE('',(#2450),#16561,.T.);
#17410=ADVANCED_FACE('',(#2451),#16562,.T.);
#17411=ADVANCED_FACE('',(#2452),#16563,.T.);
#17412=ADVANCED_FACE('',(#2453),#16564,.T.);
#17413=ADVANCED_FACE('',(#2454),#16565,.T.);
#17414=ADVANCED_FACE('',(#2455),#16566,.T.);
#17415=ADVANCED_FACE('',(#2456),#16567,.T.);
#17416=ADVANCED_FACE('',(#2457),#16568,.T.);
#17417=ADVANCED_FACE('',(#2458),#16569,.T.);
#17418=ADVANCED_FACE('',(#2459),#16570,.T.);
#17419=ADVANCED_FACE('',(#2460),#16571,.T.);
#17420=ADVANCED_FACE('',(#2461),#16572,.T.);
#17421=ADVANCED_FACE('',(#2462),#16573,.T.);
#17422=ADVANCED_FACE('',(#2463),#16574,.T.);
#17423=ADVANCED_FACE('',(#2464),#16575,.T.);
#17424=ADVANCED_FACE('',(#2465),#16576,.T.);
#17425=ADVANCED_FACE('',(#2466),#16577,.T.);
#17426=ADVANCED_FACE('',(#2467),#16578,.T.);
#17427=ADVANCED_FACE('',(#2468),#16579,.T.);
#17428=ADVANCED_FACE('',(#2469),#16580,.T.);
#17429=ADVANCED_FACE('',(#2470),#16581,.T.);
#17430=ADVANCED_FACE('',(#2471),#16582,.T.);
#17431=ADVANCED_FACE('',(#2472),#16583,.T.);
#17432=ADVANCED_FACE('',(#2473),#16584,.T.);
#17433=ADVANCED_FACE('',(#2474),#16585,.T.);
#17434=ADVANCED_FACE('',(#2475),#16586,.T.);
#17435=ADVANCED_FACE('',(#2476),#16587,.T.);
#17436=ADVANCED_FACE('',(#2477),#16588,.T.);
#17437=ADVANCED_FACE('',(#2478),#16589,.T.);
#17438=ADVANCED_FACE('',(#2479),#16590,.T.);
#17439=ADVANCED_FACE('',(#2480),#16591,.T.);
#17440=ADVANCED_FACE('',(#2481),#16592,.T.);
#17441=ADVANCED_FACE('',(#2482),#16593,.T.);
#17442=ADVANCED_FACE('',(#2483),#16594,.T.);
#17443=ADVANCED_FACE('',(#2484),#16595,.T.);
#17444=ADVANCED_FACE('',(#2485),#16596,.T.);
#17445=ADVANCED_FACE('',(#2486),#16597,.T.);
#17446=ADVANCED_FACE('',(#2487),#16598,.T.);
#17447=ADVANCED_FACE('',(#2488),#1483,.T.);
#17448=ADVANCED_FACE('',(#2489),#16599,.T.);
#17449=ADVANCED_FACE('',(#2490,#905),#1484,.F.);
#17450=ADVANCED_FACE('',(#2491,#906),#1485,.T.);
#17451=ADVANCED_FACE('',(#2492),#1486,.T.);
#17452=ADVANCED_FACE('',(#2493),#1487,.F.);
#17453=ADVANCED_FACE('',(#2494),#1488,.F.);
#17454=ADVANCED_FACE('',(#2495),#1489,.F.);
#17455=ADVANCED_FACE('',(#2496),#1490,.F.);
#17456=ADVANCED_FACE('',(#2497),#1491,.F.);
#17457=ADVANCED_FACE('',(#2498),#1492,.F.);
#17458=ADVANCED_FACE('',(#2499),#1493,.F.);
#17459=ADVANCED_FACE('',(#2500),#1494,.F.);
#17460=ADVANCED_FACE('',(#2501),#1495,.F.);
#17461=ADVANCED_FACE('',(#2502),#1496,.F.);
#17462=ADVANCED_FACE('',(#2503),#1497,.F.);
#17463=ADVANCED_FACE('',(#2504),#1498,.F.);
#17464=ADVANCED_FACE('',(#2505),#1499,.F.);
#17465=ADVANCED_FACE('',(#2506),#1500,.F.);
#17466=ADVANCED_FACE('',(#2507),#1501,.F.);
#17467=ADVANCED_FACE('',(#2508),#1502,.F.);
#17468=ADVANCED_FACE('',(#2509),#1503,.F.);
#17469=ADVANCED_FACE('',(#2510),#1504,.F.);
#17470=ADVANCED_FACE('',(#2511),#1505,.F.);
#17471=ADVANCED_FACE('',(#2512),#1506,.F.);
#17472=ADVANCED_FACE('',(#2513),#1507,.F.);
#17473=ADVANCED_FACE('',(#2514),#1508,.F.);
#17474=ADVANCED_FACE('',(#2515),#1509,.F.);
#17475=ADVANCED_FACE('',(#2516),#1510,.F.);
#17476=ADVANCED_FACE('',(#2517),#1511,.F.);
#17477=ADVANCED_FACE('',(#2518),#1512,.F.);
#17478=ADVANCED_FACE('',(#2519),#1513,.F.);
#17479=ADVANCED_FACE('',(#2520),#1514,.F.);
#17480=ADVANCED_FACE('',(#2521),#1515,.F.);
#17481=ADVANCED_FACE('',(#2522),#1516,.F.);
#17482=ADVANCED_FACE('',(#2523),#1517,.F.);
#17483=ADVANCED_FACE('',(#2524),#1518,.F.);
#17484=ADVANCED_FACE('',(#2525),#1519,.F.);
#17485=ADVANCED_FACE('',(#2526),#1520,.F.);
#17486=ADVANCED_FACE('',(#2527),#1521,.F.);
#17487=ADVANCED_FACE('',(#2528),#1522,.F.);
#17488=ADVANCED_FACE('',(#2529),#1523,.F.);
#17489=ADVANCED_FACE('',(#2530),#1524,.F.);
#17490=ADVANCED_FACE('',(#2531),#1525,.F.);
#17491=ADVANCED_FACE('',(#2532),#1526,.F.);
#17492=ADVANCED_FACE('',(#2533),#1527,.F.);
#17493=ADVANCED_FACE('',(#2534),#1528,.F.);
#17494=ADVANCED_FACE('',(#2535),#1529,.F.);
#17495=ADVANCED_FACE('',(#2536),#1530,.F.);
#17496=ADVANCED_FACE('',(#2537),#1531,.F.);
#17497=ADVANCED_FACE('',(#2538),#1532,.F.);
#17498=ADVANCED_FACE('',(#2539),#1533,.F.);
#17499=ADVANCED_FACE('',(#2540),#1534,.F.);
#17500=ADVANCED_FACE('',(#2541),#1535,.F.);
#17501=ADVANCED_FACE('',(#2542),#1536,.F.);
#17502=ADVANCED_FACE('',(#2543),#1537,.F.);
#17503=ADVANCED_FACE('',(#2544),#1538,.F.);
#17504=ADVANCED_FACE('',(#2545),#1539,.F.);
#17505=ADVANCED_FACE('',(#2546),#1540,.F.);
#17506=ADVANCED_FACE('',(#2547),#1541,.F.);
#17507=ADVANCED_FACE('',(#2548),#1542,.F.);
#17508=ADVANCED_FACE('',(#2549),#1543,.F.);
#17509=ADVANCED_FACE('',(#2550),#1544,.F.);
#17510=ADVANCED_FACE('',(#2551),#1545,.F.);
#17511=ADVANCED_FACE('',(#2552),#1546,.F.);
#17512=ADVANCED_FACE('',(#2553),#1547,.F.);
#17513=ADVANCED_FACE('',(#2554),#1548,.F.);
#17514=ADVANCED_FACE('',(#2555),#1549,.F.);
#17515=ADVANCED_FACE('',(#2556),#1550,.F.);
#17516=ADVANCED_FACE('',(#2557),#1551,.F.);
#17517=ADVANCED_FACE('',(#2558),#1552,.F.);
#17518=ADVANCED_FACE('',(#2559),#1553,.F.);
#17519=ADVANCED_FACE('',(#2560),#1554,.F.);
#17520=ADVANCED_FACE('',(#2561),#1555,.F.);
#17521=ADVANCED_FACE('',(#2562),#1556,.F.);
#17522=ADVANCED_FACE('',(#2563),#1557,.F.);
#17523=ADVANCED_FACE('',(#2564),#1558,.F.);
#17524=ADVANCED_FACE('',(#2565),#1559,.F.);
#17525=ADVANCED_FACE('',(#2566),#1560,.F.);
#17526=ADVANCED_FACE('',(#2567),#1561,.F.);
#17527=ADVANCED_FACE('',(#2568),#1562,.F.);
#17528=ADVANCED_FACE('',(#2569),#1563,.F.);
#17529=ADVANCED_FACE('',(#2570),#1564,.F.);
#17530=ADVANCED_FACE('',(#2571),#1565,.F.);
#17531=ADVANCED_FACE('',(#2572),#1566,.F.);
#17532=ADVANCED_FACE('',(#2573),#1567,.F.);
#17533=ADVANCED_FACE('',(#2574),#1568,.F.);
#17534=ADVANCED_FACE('',(#2575),#1569,.F.);
#17535=ADVANCED_FACE('',(#2576),#1570,.F.);
#17536=ADVANCED_FACE('',(#2577),#1571,.F.);
#17537=ADVANCED_FACE('',(#2578),#1572,.F.);
#17538=ADVANCED_FACE('',(#2579),#1573,.F.);
#17539=ADVANCED_FACE('',(#2580),#1574,.F.);
#17540=ADVANCED_FACE('',(#2581),#1575,.F.);
#17541=ADVANCED_FACE('',(#2582),#1576,.F.);
#17542=ADVANCED_FACE('',(#2583),#1577,.F.);
#17543=ADVANCED_FACE('',(#2584),#1578,.F.);
#17544=ADVANCED_FACE('',(#2585),#1579,.F.);
#17545=ADVANCED_FACE('',(#2586),#1580,.F.);
#17546=ADVANCED_FACE('',(#2587),#1581,.F.);
#17547=ADVANCED_FACE('',(#2588),#1582,.F.);
#17548=ADVANCED_FACE('',(#2589),#1583,.F.);
#17549=ADVANCED_FACE('',(#2590),#1584,.F.);
#17550=ADVANCED_FACE('',(#2591),#1585,.F.);
#17551=ADVANCED_FACE('',(#2592),#1586,.F.);
#17552=ADVANCED_FACE('',(#2593),#1587,.F.);
#17553=ADVANCED_FACE('',(#2594),#1588,.F.);
#17554=ADVANCED_FACE('',(#2595),#1589,.F.);
#17555=ADVANCED_FACE('',(#2596),#1590,.F.);
#17556=ADVANCED_FACE('',(#2597),#1591,.F.);
#17557=ADVANCED_FACE('',(#2598),#1592,.F.);
#17558=ADVANCED_FACE('',(#2599),#1593,.F.);
#17559=ADVANCED_FACE('',(#2600),#1594,.F.);
#17560=ADVANCED_FACE('',(#2601),#1595,.F.);
#17561=ADVANCED_FACE('',(#2602),#1596,.F.);
#17562=ADVANCED_FACE('',(#2603),#1597,.F.);
#17563=ADVANCED_FACE('',(#2604),#1598,.F.);
#17564=ADVANCED_FACE('',(#2605),#1599,.F.);
#17565=ADVANCED_FACE('',(#2606),#1600,.F.);
#17566=ADVANCED_FACE('',(#2607),#1601,.F.);
#17567=ADVANCED_FACE('',(#2608),#1602,.F.);
#17568=ADVANCED_FACE('',(#2609),#1603,.F.);
#17569=ADVANCED_FACE('',(#2610),#1604,.F.);
#17570=ADVANCED_FACE('',(#2611),#1605,.F.);
#17571=ADVANCED_FACE('',(#2612),#1606,.F.);
#17572=ADVANCED_FACE('',(#2613),#1607,.F.);
#17573=ADVANCED_FACE('',(#2614),#1608,.F.);
#17574=ADVANCED_FACE('',(#2615),#1609,.F.);
#17575=ADVANCED_FACE('',(#2616),#1610,.F.);
#17576=ADVANCED_FACE('',(#2617),#1611,.F.);
#17577=ADVANCED_FACE('',(#2618),#1612,.F.);
#17578=ADVANCED_FACE('',(#2619),#1613,.F.);
#17579=ADVANCED_FACE('',(#2620),#1614,.F.);
#17580=ADVANCED_FACE('',(#2621),#1615,.F.);
#17581=ADVANCED_FACE('',(#2622),#1616,.F.);
#17582=ADVANCED_FACE('',(#2623),#1617,.F.);
#17583=ADVANCED_FACE('',(#2624),#1618,.F.);
#17584=ADVANCED_FACE('',(#2625),#1619,.F.);
#17585=ADVANCED_FACE('',(#2626),#1620,.F.);
#17586=ADVANCED_FACE('',(#2627),#1621,.F.);
#17587=ADVANCED_FACE('',(#2628),#1622,.F.);
#17588=ADVANCED_FACE('',(#2629),#1623,.F.);
#17589=ADVANCED_FACE('',(#2630),#1624,.F.);
#17590=ADVANCED_FACE('',(#2631),#1625,.F.);
#17591=ADVANCED_FACE('',(#2632),#1626,.F.);
#17592=ADVANCED_FACE('',(#2633),#1627,.F.);
#17593=ADVANCED_FACE('',(#2634),#1628,.F.);
#17594=ADVANCED_FACE('',(#2635),#1629,.F.);
#17595=ADVANCED_FACE('',(#2636),#1630,.F.);
#17596=ADVANCED_FACE('',(#2637),#1631,.F.);
#17597=ADVANCED_FACE('',(#2638),#1632,.F.);
#17598=ADVANCED_FACE('',(#2639),#1633,.F.);
#17599=ADVANCED_FACE('',(#2640),#1634,.F.);
#17600=ADVANCED_FACE('',(#2641),#1635,.F.);
#17601=ADVANCED_FACE('',(#2642),#1636,.F.);
#17602=ADVANCED_FACE('',(#2643),#1637,.F.);
#17603=ADVANCED_FACE('',(#2644),#1638,.F.);
#17604=ADVANCED_FACE('',(#2645),#1639,.F.);
#17605=ADVANCED_FACE('',(#2646),#1640,.F.);
#17625=CLOSED_SHELL('',(#16928,#16929,#16930,#16931,#16932,#16933,#16934,
#16935,#16936,#16937,#16938,#16939,#16940,#16941,#16942,#16943,#16944,#16945,
#16946,#16947,#16948,#16949,#16950,#16951,#16952,#16953,#16954,#16955,#16956,
#16957,#16958,#16959,#16960,#16961,#16962,#16963,#16964,#16965,#16966,#16967,
#16968,#16969,#16970,#16971,#16972,#16973,#16974,#16975,#16976,#16977,#16978,
#16979,#16980,#16981,#16982,#16983,#16984,#16985,#16986,#16987,#16988,#16989,
#16990,#16991,#16992,#16993,#16994,#16995,#16996,#16997,#16998,#16999,#17000,
#17001,#17002,#17003));
#17626=CLOSED_SHELL('',(#17004,#17005,#17006,#17007,#17008));
#17627=CLOSED_SHELL('',(#17009,#17010,#17011,#17012,#17013,#17014,#17015,
#17016,#17017,#17018,#17019,#17020,#17021,#17022,#17023,#17024,#17025,#17026,
#17027,#17028,#17029,#17030));
#17628=CLOSED_SHELL('',(#17031,#17032,#17033));
#17629=CLOSED_SHELL('',(#17034,#17035,#17036,#17037,#17038,#17039,#17040,
#17041,#17042,#17043,#17044,#17045,#17046,#17047,#17048,#17049,#17050,#17051,
#17052,#17053,#17054,#17055,#17056,#17057,#17058,#17059,#17060,#17061,#17062,
#17063,#17064,#17065,#17066,#17067,#17068,#17069,#17070,#17071,#17072,#17073,
#17074,#17075,#17076,#17077,#17078,#17079,#17080,#17081,#17082,#17083,#17084,
#17085,#17086,#17087,#17088,#17089,#17090,#17091,#17092,#17093,#17094,#17095,
#17096,#17097,#17098,#17099,#17100,#17101,#17102,#17103,#17104,#17105,#17106,
#17107,#17108,#17109,#17110,#17111,#17112,#17113,#17114,#17115,#17116,#17117,
#17118,#17119,#17120,#17121,#17122,#17123,#17124,#17125,#17126,#17127,#17128,
#17129,#17130,#17131,#17132,#17133,#17134,#17135,#17136,#17137,#17138,#17139,
#17140,#17141,#17142,#17143,#17144,#17145,#17146,#17147,#17148,#17149,#17150,
#17151,#17152,#17153,#17154,#17155,#17156,#17157,#17158,#17159,#17160,#17161,
#17162,#17163,#17164,#17165,#17166,#17167,#17168,#17169,#17170,#17171,#17172,
#17173,#17174,#17175,#17176,#17177,#17178,#17179,#17180,#17181,#17182,#17183,
#17184,#17185,#17186,#17187,#17188,#17189,#17190,#17191,#17192,#17193,#17194,
#17195,#17196,#17197,#17198,#17199,#17200,#17201,#17202,#17203,#17204,#17205,
#17206,#17207,#17208,#17209,#17210,#17211,#17212,#17213,#17214,#17215,#17216,
#17217,#17218,#17219,#17220,#17221,#17222,#17223,#17224,#17225,#17226,#17227,
#17228,#17229,#17230,#17231,#17232,#17233,#17234,#17235,#17236,#17237,#17238,
#17239,#17240,#17241,#17242,#17243,#17244,#17245,#17246,#17247,#17248,#17249,
#17250,#17251,#17252,#17253,#17254,#17255,#17256,#17257,#17258,#17259,#17260,
#17261,#17262,#17263,#17264,#17265,#17266,#17267,#17268,#17269,#17270,#17271,
#17272,#17273,#17274,#17275,#17276,#17277,#17278,#17279,#17280,#17281,#17282,
#17283,#17284,#17285,#17286,#17287,#17288,#17289,#17290,#17291,#17292,#17293,
#17294,#17295,#17296,#17297,#17298,#17299,#17300,#17301,#17302,#17303,#17304,
#17305,#17306,#17307,#17308,#17309,#17310,#17311,#17312,#17313,#17314,#17315,
#17316));
#17630=CLOSED_SHELL('',(#17317,#17318,#17319,#17320,#17321,#17322,#17323,
#17324,#17325,#17326));
#17631=CLOSED_SHELL('',(#17327,#17328,#17329,#17330,#17331,#17332,#17333,
#17334,#17335,#17336,#17337,#17338,#17339,#17340,#17341,#17342,#17343,#17344,
#17345,#17346,#17347,#17348,#17349,#17350,#17351,#17352,#17353,#17354,#17355,
#17356,#17357,#17358,#17359,#17360,#17361,#17362,#17363,#17364,#17365,#17366,
#17367,#17368,#17369,#17370,#17371,#17372,#17373,#17374,#17375,#17376,#17377,
#17378,#17379,#17380,#17381,#17382,#17383,#17384,#17385,#17386,#17387,#17388,
#17389,#17390,#17391,#17392,#17393,#17394,#17395,#17396,#17397,#17398,#17399,
#17400,#17401,#17402,#17403,#17404,#17405,#17406,#17407,#17408,#17409,#17410,
#17411,#17412,#17413,#17414,#17415,#17416,#17417,#17418,#17419,#17420,#17421,
#17422,#17423,#17424,#17425,#17426,#17427,#17428,#17429,#17430,#17431,#17432,
#17433,#17434,#17435,#17436,#17437,#17438,#17439,#17440,#17441,#17442,#17443,
#17444,#17445,#17446,#17447,#17448,#17449,#17450,#17451,#17452,#17453,#17454,
#17455,#17456,#17457,#17458,#17459,#17460,#17461,#17462,#17463,#17464,#17465,
#17466,#17467,#17468,#17469,#17470,#17471,#17472,#17473,#17474,#17475,#17476,
#17477,#17478,#17479,#17480,#17481,#17482,#17483,#17484,#17485,#17486,#17487,
#17488,#17489,#17490,#17491,#17492,#17493,#17494,#17495,#17496,#17497,#17498,
#17499,#17500,#17501,#17502,#17503,#17504,#17505,#17506,#17507,#17508,#17509,
#17510,#17511,#17512,#17513,#17514,#17515,#17516,#17517,#17518,#17519,#17520,
#17521,#17522,#17523,#17524,#17525,#17526,#17527,#17528,#17529,#17530,#17531,
#17532,#17533,#17534,#17535,#17536,#17537,#17538,#17539,#17540,#17541,#17542,
#17543,#17544,#17545,#17546,#17547,#17548,#17549,#17550,#17551,#17552,#17553,
#17554,#17555,#17556,#17557,#17558,#17559,#17560,#17561,#17562,#17563,#17564,
#17565,#17566,#17567,#17568,#17569,#17570,#17571,#17572,#17573,#17574,#17575,
#17576,#17577,#17578,#17579,#17580,#17581,#17582,#17583,#17584,#17585,#17586,
#17587,#17588,#17589,#17590,#17591,#17592,#17593,#17594,#17595,#17596,#17597,
#17598,#17599,#17600,#17601,#17602,#17603,#17604,#17605));
#18447=AXIS2_PLACEMENT_3D('',#33359,#21309,#21310);
#18448=AXIS2_PLACEMENT_3D('',#33360,#21311,#21312);
#18449=AXIS2_PLACEMENT_3D('',#33362,#21313,#21314);
#18450=AXIS2_PLACEMENT_3D('',#33365,#21316,#21317);
#18451=AXIS2_PLACEMENT_3D('',#33366,#21318,#21319);
#18452=AXIS2_PLACEMENT_3D('',#33369,#21320,#21321);
#18453=AXIS2_PLACEMENT_3D('',#33370,#21322,#21323);
#18454=AXIS2_PLACEMENT_3D('',#33373,#21325,#21326);
#18455=AXIS2_PLACEMENT_3D('',#33374,#21327,#21328);
#18456=AXIS2_PLACEMENT_3D('',#33377,#21329,#21330);
#18457=AXIS2_PLACEMENT_3D('',#33378,#21331,#21332);
#18458=AXIS2_PLACEMENT_3D('',#33381,#21334,#21335);
#18459=AXIS2_PLACEMENT_3D('',#33382,#21336,#21337);
#18460=AXIS2_PLACEMENT_3D('',#33384,#21338,#21339);
#18461=AXIS2_PLACEMENT_3D('',#33387,#21341,#21342);
#18462=AXIS2_PLACEMENT_3D('',#33388,#21343,#21344);
#18463=AXIS2_PLACEMENT_3D('',#33391,#21345,#21346);
#18464=AXIS2_PLACEMENT_3D('',#33397,#21347,#21348);
#18465=AXIS2_PLACEMENT_3D('',#33401,#21349,#21350);
#18466=AXIS2_PLACEMENT_3D('',#33404,#21351,#21352);
#18467=AXIS2_PLACEMENT_3D('',#33405,#21353,#21354);
#18468=AXIS2_PLACEMENT_3D('',#33408,#21356,#21357);
#18469=AXIS2_PLACEMENT_3D('',#33409,#21358,#21359);
#18470=AXIS2_PLACEMENT_3D('',#33412,#21360,#21361);
#18471=AXIS2_PLACEMENT_3D('',#33413,#21362,#21363);
#18472=AXIS2_PLACEMENT_3D('',#33416,#21365,#21366);
#18473=AXIS2_PLACEMENT_3D('',#33417,#21367,#21368);
#18474=AXIS2_PLACEMENT_3D('',#33419,#21369,#21370);
#18475=AXIS2_PLACEMENT_3D('',#33422,#21372,#21373);
#18476=AXIS2_PLACEMENT_3D('',#33423,#21374,#21375);
#18477=AXIS2_PLACEMENT_3D('',#33425,#21376,#21377);
#18478=AXIS2_PLACEMENT_3D('',#33428,#21379,#21380);
#18479=AXIS2_PLACEMENT_3D('',#33429,#21381,#21382);
#18480=AXIS2_PLACEMENT_3D('',#33432,#21383,#21384);
#18481=AXIS2_PLACEMENT_3D('',#33438,#21385,#21386);
#18482=AXIS2_PLACEMENT_3D('',#33442,#21387,#21388);
#18483=AXIS2_PLACEMENT_3D('',#33446,#21390,#21391);
#18484=AXIS2_PLACEMENT_3D('',#33475,#21392,#21393);
#18485=AXIS2_PLACEMENT_3D('',#33476,#21394,#21395);
#18486=AXIS2_PLACEMENT_3D('',#33478,#21396,#21397);
#18487=AXIS2_PLACEMENT_3D('',#33480,#21399,#21400);
#18488=AXIS2_PLACEMENT_3D('',#33482,#21402,#21403);
#18489=AXIS2_PLACEMENT_3D('',#33486,#21407,#21408);
#18490=AXIS2_PLACEMENT_3D('',#33488,#21410,#21411);
#18491=AXIS2_PLACEMENT_3D('',#33490,#21413,#21414);
#18492=AXIS2_PLACEMENT_3D('',#33499,#21419,#21420);
#18493=AXIS2_PLACEMENT_3D('',#33508,#21425,#21426);
#18494=AXIS2_PLACEMENT_3D('',#33512,#21428,#21429);
#18495=AXIS2_PLACEMENT_3D('',#33533,#21440,#21441);
#18496=AXIS2_PLACEMENT_3D('',#33535,#21443,#21444);
#18497=AXIS2_PLACEMENT_3D('',#33541,#21448,#21449);
#18498=AXIS2_PLACEMENT_3D('',#33547,#21452,#21453);
#18499=AXIS2_PLACEMENT_3D('',#33572,#21467,#21468);
#18500=AXIS2_PLACEMENT_3D('',#33573,#21469,#21470);
#18501=AXIS2_PLACEMENT_3D('',#33582,#21475,#21476);
#18502=AXIS2_PLACEMENT_3D('',#33596,#21484,#21485);
#18503=AXIS2_PLACEMENT_3D('',#33607,#21490,#21491);
#18504=AXIS2_PLACEMENT_3D('',#33611,#21494,#21495);
#18505=AXIS2_PLACEMENT_3D('',#33622,#21500,#21501);
#18506=AXIS2_PLACEMENT_3D('',#33630,#21506,#21507);
#18507=AXIS2_PLACEMENT_3D('',#33635,#21509,#21510);
#18508=AXIS2_PLACEMENT_3D('',#33638,#21512,#21513);
#18509=AXIS2_PLACEMENT_3D('',#33639,#21514,#21515);
#18510=AXIS2_PLACEMENT_3D('',#33648,#21516,#21517);
#18511=AXIS2_PLACEMENT_3D('',#33660,#21519,#21520);
#18512=AXIS2_PLACEMENT_3D('',#33664,#21522,#21523);
#18513=AXIS2_PLACEMENT_3D('',#33665,#21524,#21525);
#18514=AXIS2_PLACEMENT_3D('',#33666,#21526,#21527);
#18515=AXIS2_PLACEMENT_3D('',#33676,#21529,#21530);
#18516=AXIS2_PLACEMENT_3D('',#33678,#21532,#21533);
#18517=AXIS2_PLACEMENT_3D('',#33679,#21534,#21535);
#18518=AXIS2_PLACEMENT_3D('',#33681,#21537,#21538);
#18519=AXIS2_PLACEMENT_3D('',#33683,#21540,#21541);
#18520=AXIS2_PLACEMENT_3D('',#33692,#21542,#21543);
#18521=AXIS2_PLACEMENT_3D('',#33698,#21546,#21547);
#18522=AXIS2_PLACEMENT_3D('',#33702,#21550,#21551);
#18523=AXIS2_PLACEMENT_3D('',#33706,#21554,#21555);
#18524=AXIS2_PLACEMENT_3D('',#33712,#21559,#21560);
#18525=AXIS2_PLACEMENT_3D('',#33716,#21563,#21564);
#18526=AXIS2_PLACEMENT_3D('',#33717,#21565,#21566);
#18527=AXIS2_PLACEMENT_3D('',#33718,#21567,#21568);
#18528=AXIS2_PLACEMENT_3D('',#33723,#21571,#21572);
#18529=AXIS2_PLACEMENT_3D('',#33724,#21573,#21574);
#18530=AXIS2_PLACEMENT_3D('',#33730,#21578,#21579);
#18531=AXIS2_PLACEMENT_3D('',#33731,#21580,#21581);
#18532=AXIS2_PLACEMENT_3D('',#33732,#21582,#21583);
#18533=AXIS2_PLACEMENT_3D('',#33733,#21584,#21585);
#18534=AXIS2_PLACEMENT_3D('',#33734,#21586,#21587);
#18535=AXIS2_PLACEMENT_3D('',#33735,#21588,#21589);
#18536=AXIS2_PLACEMENT_3D('',#33736,#21590,#21591);
#18537=AXIS2_PLACEMENT_3D('',#33737,#21592,#21593);
#18538=AXIS2_PLACEMENT_3D('',#33738,#21594,#21595);
#18539=AXIS2_PLACEMENT_3D('',#33739,#21596,#21597);
#18540=AXIS2_PLACEMENT_3D('',#33740,#21598,#21599);
#18541=AXIS2_PLACEMENT_3D('',#33741,#21600,#21601);
#18542=AXIS2_PLACEMENT_3D('',#33742,#21602,#21603);
#18543=AXIS2_PLACEMENT_3D('',#33743,#21604,#21605);
#18544=AXIS2_PLACEMENT_3D('',#33744,#21606,#21607);
#18545=AXIS2_PLACEMENT_3D('',#33745,#21608,#21609);
#18546=AXIS2_PLACEMENT_3D('',#33746,#21610,#21611);
#18547=AXIS2_PLACEMENT_3D('',#33747,#21612,#21613);
#18548=AXIS2_PLACEMENT_3D('',#33748,#21614,#21615);
#18549=AXIS2_PLACEMENT_3D('',#33749,#21616,#21617);
#18550=AXIS2_PLACEMENT_3D('',#33750,#21618,#21619);
#18551=AXIS2_PLACEMENT_3D('',#33751,#21620,#21621);
#18552=AXIS2_PLACEMENT_3D('',#33752,#21622,#21623);
#18553=AXIS2_PLACEMENT_3D('',#33753,#21624,#21625);
#18554=AXIS2_PLACEMENT_3D('',#33754,#21626,#21627);
#18555=AXIS2_PLACEMENT_3D('',#33755,#21628,#21629);
#18556=AXIS2_PLACEMENT_3D('',#33756,#21630,#21631);
#18557=AXIS2_PLACEMENT_3D('',#33757,#21632,#21633);
#18558=AXIS2_PLACEMENT_3D('',#33758,#21634,#21635);
#18559=AXIS2_PLACEMENT_3D('',#33759,#21636,#21637);
#18560=AXIS2_PLACEMENT_3D('',#33760,#21638,#21639);
#18561=AXIS2_PLACEMENT_3D('',#33761,#21640,#21641);
#18562=AXIS2_PLACEMENT_3D('',#33762,#21642,#21643);
#18563=AXIS2_PLACEMENT_3D('',#33763,#21644,#21645);
#18564=AXIS2_PLACEMENT_3D('',#33764,#21646,#21647);
#18565=AXIS2_PLACEMENT_3D('',#33765,#21648,#21649);
#18566=AXIS2_PLACEMENT_3D('',#33766,#21650,#21651);
#18567=AXIS2_PLACEMENT_3D('',#33767,#21652,#21653);
#18568=AXIS2_PLACEMENT_3D('',#33768,#21654,#21655);
#18569=AXIS2_PLACEMENT_3D('',#33769,#21656,#21657);
#18570=AXIS2_PLACEMENT_3D('',#33770,#21658,#21659);
#18571=AXIS2_PLACEMENT_3D('',#33771,#21660,#21661);
#18572=AXIS2_PLACEMENT_3D('',#33772,#21662,#21663);
#18573=AXIS2_PLACEMENT_3D('',#33773,#21664,#21665);
#18574=AXIS2_PLACEMENT_3D('',#33774,#21666,#21667);
#18575=AXIS2_PLACEMENT_3D('',#33775,#21668,#21669);
#18576=AXIS2_PLACEMENT_3D('',#33776,#21670,#21671);
#18577=AXIS2_PLACEMENT_3D('',#33777,#21672,#21673);
#18578=AXIS2_PLACEMENT_3D('',#33778,#21674,#21675);
#18579=AXIS2_PLACEMENT_3D('',#33779,#21676,#21677);
#18580=AXIS2_PLACEMENT_3D('',#33780,#21678,#21679);
#18581=AXIS2_PLACEMENT_3D('',#33781,#21680,#21681);
#18582=AXIS2_PLACEMENT_3D('',#33782,#21682,#21683);
#18583=AXIS2_PLACEMENT_3D('',#33783,#21684,#21685);
#18584=AXIS2_PLACEMENT_3D('',#33784,#21686,#21687);
#18585=AXIS2_PLACEMENT_3D('',#33785,#21688,#21689);
#18586=AXIS2_PLACEMENT_3D('',#33786,#21690,#21691);
#18587=AXIS2_PLACEMENT_3D('',#33787,#21692,#21693);
#18588=AXIS2_PLACEMENT_3D('',#33788,#21694,#21695);
#18589=AXIS2_PLACEMENT_3D('',#33789,#21696,#21697);
#18590=AXIS2_PLACEMENT_3D('',#33790,#21698,#21699);
#18591=AXIS2_PLACEMENT_3D('',#33791,#21700,#21701);
#18592=AXIS2_PLACEMENT_3D('',#33792,#21702,#21703);
#18593=AXIS2_PLACEMENT_3D('',#33793,#21704,#21705);
#18594=AXIS2_PLACEMENT_3D('',#33794,#21706,#21707);
#18595=AXIS2_PLACEMENT_3D('',#33795,#21708,#21709);
#18596=AXIS2_PLACEMENT_3D('',#33796,#21710,#21711);
#18597=AXIS2_PLACEMENT_3D('',#33797,#21712,#21713);
#18598=AXIS2_PLACEMENT_3D('',#33799,#21714,#21715);
#18599=AXIS2_PLACEMENT_3D('',#33801,#21716,#21717);
#18600=AXIS2_PLACEMENT_3D('',#33803,#21718,#21719);
#18601=AXIS2_PLACEMENT_3D('',#33804,#21720,#21721);
#18602=AXIS2_PLACEMENT_3D('',#33805,#21722,#21723);
#18603=AXIS2_PLACEMENT_3D('',#33808,#21724,#21725);
#18604=AXIS2_PLACEMENT_3D('',#33809,#21726,#21727);
#18605=AXIS2_PLACEMENT_3D('',#33811,#21728,#21729);
#18606=AXIS2_PLACEMENT_3D('',#33812,#21730,#21731);
#18607=AXIS2_PLACEMENT_3D('',#33813,#21732,#21733);
#18608=AXIS2_PLACEMENT_3D('',#33815,#21735,#21736);
#18609=AXIS2_PLACEMENT_3D('',#33816,#21737,#21738);
#18610=AXIS2_PLACEMENT_3D('',#33817,#21739,#21740);
#18611=AXIS2_PLACEMENT_3D('',#33819,#21741,#21742);
#18612=AXIS2_PLACEMENT_3D('',#33822,#21744,#21745);
#18613=AXIS2_PLACEMENT_3D('',#33823,#21746,#21747);
#18614=AXIS2_PLACEMENT_3D('',#33826,#21748,#21749);
#18615=AXIS2_PLACEMENT_3D('',#33828,#21750,#21751);
#18616=AXIS2_PLACEMENT_3D('',#33831,#21753,#21754);
#18617=AXIS2_PLACEMENT_3D('',#33832,#21755,#21756);
#18618=AXIS2_PLACEMENT_3D('',#33833,#21757,#21758);
#18619=AXIS2_PLACEMENT_3D('',#33835,#21759,#21760);
#18620=AXIS2_PLACEMENT_3D('',#33838,#21762,#21763);
#18621=AXIS2_PLACEMENT_3D('',#33839,#21764,#21765);
#18622=AXIS2_PLACEMENT_3D('',#33841,#21766,#21767);
#18623=AXIS2_PLACEMENT_3D('',#33844,#21769,#21770);
#18624=AXIS2_PLACEMENT_3D('',#33845,#21771,#21772);
#18625=AXIS2_PLACEMENT_3D('',#33847,#21773,#21774);
#18626=AXIS2_PLACEMENT_3D('',#33850,#21776,#21777);
#18627=AXIS2_PLACEMENT_3D('',#33851,#21778,#21779);
#18628=AXIS2_PLACEMENT_3D('',#33853,#21780,#21781);
#18629=AXIS2_PLACEMENT_3D('',#33856,#21783,#21784);
#18630=AXIS2_PLACEMENT_3D('',#33857,#21785,#21786);
#18631=AXIS2_PLACEMENT_3D('',#33863,#21790,#21791);
#18632=AXIS2_PLACEMENT_3D('',#33868,#21793,#21794);
#18633=AXIS2_PLACEMENT_3D('',#33871,#21796,#21797);
#18634=AXIS2_PLACEMENT_3D('',#33872,#21798,#21799);
#18635=AXIS2_PLACEMENT_3D('',#33878,#21803,#21804);
#18636=AXIS2_PLACEMENT_3D('',#33881,#21807,#21808);
#18637=AXIS2_PLACEMENT_3D('',#33890,#21812,#21813);
#18638=AXIS2_PLACEMENT_3D('',#33892,#21815,#21816);
#18639=AXIS2_PLACEMENT_3D('',#33895,#21819,#21820);
#18640=AXIS2_PLACEMENT_3D('',#33903,#21825,#21826);
#18641=AXIS2_PLACEMENT_3D('',#33906,#21828,#21829);
#18642=AXIS2_PLACEMENT_3D('',#33907,#21830,#21831);
#18643=AXIS2_PLACEMENT_3D('',#33911,#21834,#21835);
#18644=AXIS2_PLACEMENT_3D('',#33917,#21839,#21840);
#18645=AXIS2_PLACEMENT_3D('',#33919,#21842,#21843);
#18646=AXIS2_PLACEMENT_3D('',#33921,#21845,#21846);
#18647=AXIS2_PLACEMENT_3D('',#33922,#21847,#21848);
#18648=AXIS2_PLACEMENT_3D('',#33923,#21849,#21850);
#18649=AXIS2_PLACEMENT_3D('',#33924,#21851,#21852);
#18650=AXIS2_PLACEMENT_3D('',#33925,#21853,#21854);
#18651=AXIS2_PLACEMENT_3D('',#33927,#21855,#21856);
#18652=AXIS2_PLACEMENT_3D('',#33930,#21858,#21859);
#18653=AXIS2_PLACEMENT_3D('',#33931,#21860,#21861);
#18654=AXIS2_PLACEMENT_3D('',#33934,#21862,#21863);
#18655=AXIS2_PLACEMENT_3D('',#33935,#21864,#21865);
#18656=AXIS2_PLACEMENT_3D('',#33936,#21866,#21867);
#18657=AXIS2_PLACEMENT_3D('',#33938,#21868,#21869);
#18658=AXIS2_PLACEMENT_3D('',#33940,#21870,#21871);
#18659=AXIS2_PLACEMENT_3D('',#33941,#21872,#21873);
#18660=AXIS2_PLACEMENT_3D('',#33942,#21874,#21875);
#18661=AXIS2_PLACEMENT_3D('',#33945,#21876,#21877);
#18662=AXIS2_PLACEMENT_3D('',#33946,#21878,#21879);
#18663=AXIS2_PLACEMENT_3D('',#33949,#21881,#21882);
#18664=AXIS2_PLACEMENT_3D('',#33950,#21883,#21884);
#18665=AXIS2_PLACEMENT_3D('',#33953,#21885,#21886);
#18666=AXIS2_PLACEMENT_3D('',#33954,#21887,#21888);
#18667=AXIS2_PLACEMENT_3D('',#33958,#21890,#21891);
#18668=AXIS2_PLACEMENT_3D('',#33959,#21892,#21893);
#18669=AXIS2_PLACEMENT_3D('',#33960,#21894,#21895);
#18670=AXIS2_PLACEMENT_3D('',#33962,#21897,#21898);
#18671=AXIS2_PLACEMENT_3D('',#33965,#21899,#21900);
#18672=AXIS2_PLACEMENT_3D('',#33966,#21901,#21902);
#18673=AXIS2_PLACEMENT_3D('',#33968,#21904,#21905);
#18674=AXIS2_PLACEMENT_3D('',#33971,#21906,#21907);
#18675=AXIS2_PLACEMENT_3D('',#33972,#21908,#21909);
#18676=AXIS2_PLACEMENT_3D('',#33976,#21911,#21912);
#18677=AXIS2_PLACEMENT_3D('',#33977,#21913,#21914);
#18678=AXIS2_PLACEMENT_3D('',#33978,#21915,#21916);
#18679=AXIS2_PLACEMENT_3D('',#33980,#21918,#21919);
#18680=AXIS2_PLACEMENT_3D('',#33983,#21920,#21921);
#18681=AXIS2_PLACEMENT_3D('',#33984,#21922,#21923);
#18682=AXIS2_PLACEMENT_3D('',#33986,#21925,#21926);
#18683=AXIS2_PLACEMENT_3D('',#33989,#21927,#21928);
#18684=AXIS2_PLACEMENT_3D('',#33990,#21929,#21930);
#18685=AXIS2_PLACEMENT_3D('',#33994,#21932,#21933);
#18686=AXIS2_PLACEMENT_3D('',#33995,#21934,#21935);
#18687=AXIS2_PLACEMENT_3D('',#33996,#21936,#21937);
#18688=AXIS2_PLACEMENT_3D('',#33998,#21939,#21940);
#18689=AXIS2_PLACEMENT_3D('',#34001,#21941,#21942);
#18690=AXIS2_PLACEMENT_3D('',#34002,#21943,#21944);
#18691=AXIS2_PLACEMENT_3D('',#34004,#21946,#21947);
#18692=AXIS2_PLACEMENT_3D('',#34007,#21948,#21949);
#18693=AXIS2_PLACEMENT_3D('',#34008,#21950,#21951);
#18694=AXIS2_PLACEMENT_3D('',#34012,#21953,#21954);
#18695=AXIS2_PLACEMENT_3D('',#34013,#21955,#21956);
#18696=AXIS2_PLACEMENT_3D('',#34014,#21957,#21958);
#18697=AXIS2_PLACEMENT_3D('',#34016,#21960,#21961);
#18698=AXIS2_PLACEMENT_3D('',#34019,#21962,#21963);
#18699=AXIS2_PLACEMENT_3D('',#34020,#21964,#21965);
#18700=AXIS2_PLACEMENT_3D('',#34022,#21967,#21968);
#18701=AXIS2_PLACEMENT_3D('',#34025,#21969,#21970);
#18702=AXIS2_PLACEMENT_3D('',#34026,#21971,#21972);
#18703=AXIS2_PLACEMENT_3D('',#34030,#21974,#21975);
#18704=AXIS2_PLACEMENT_3D('',#34031,#21976,#21977);
#18705=AXIS2_PLACEMENT_3D('',#34032,#21978,#21979);
#18706=AXIS2_PLACEMENT_3D('',#34034,#21981,#21982);
#18707=AXIS2_PLACEMENT_3D('',#34037,#21983,#21984);
#18708=AXIS2_PLACEMENT_3D('',#34038,#21985,#21986);
#18709=AXIS2_PLACEMENT_3D('',#34040,#21988,#21989);
#18710=AXIS2_PLACEMENT_3D('',#34043,#21990,#21991);
#18711=AXIS2_PLACEMENT_3D('',#34044,#21992,#21993);
#18712=AXIS2_PLACEMENT_3D('',#34048,#21995,#21996);
#18713=AXIS2_PLACEMENT_3D('',#34049,#21997,#21998);
#18714=AXIS2_PLACEMENT_3D('',#34050,#21999,#22000);
#18715=AXIS2_PLACEMENT_3D('',#34052,#22002,#22003);
#18716=AXIS2_PLACEMENT_3D('',#34055,#22004,#22005);
#18717=AXIS2_PLACEMENT_3D('',#34056,#22006,#22007);
#18718=AXIS2_PLACEMENT_3D('',#34058,#22009,#22010);
#18719=AXIS2_PLACEMENT_3D('',#34061,#22011,#22012);
#18720=AXIS2_PLACEMENT_3D('',#34062,#22013,#22014);
#18721=AXIS2_PLACEMENT_3D('',#34066,#22016,#22017);
#18722=AXIS2_PLACEMENT_3D('',#34067,#22018,#22019);
#18723=AXIS2_PLACEMENT_3D('',#34068,#22020,#22021);
#18724=AXIS2_PLACEMENT_3D('',#34070,#22023,#22024);
#18725=AXIS2_PLACEMENT_3D('',#34073,#22025,#22026);
#18726=AXIS2_PLACEMENT_3D('',#34074,#22027,#22028);
#18727=AXIS2_PLACEMENT_3D('',#34076,#22030,#22031);
#18728=AXIS2_PLACEMENT_3D('',#34079,#22032,#22033);
#18729=AXIS2_PLACEMENT_3D('',#34080,#22034,#22035);
#18730=AXIS2_PLACEMENT_3D('',#34084,#22037,#22038);
#18731=AXIS2_PLACEMENT_3D('',#34085,#22039,#22040);
#18732=AXIS2_PLACEMENT_3D('',#34086,#22041,#22042);
#18733=AXIS2_PLACEMENT_3D('',#34088,#22044,#22045);
#18734=AXIS2_PLACEMENT_3D('',#34091,#22046,#22047);
#18735=AXIS2_PLACEMENT_3D('',#34092,#22048,#22049);
#18736=AXIS2_PLACEMENT_3D('',#34094,#22051,#22052);
#18737=AXIS2_PLACEMENT_3D('',#34097,#22053,#22054);
#18738=AXIS2_PLACEMENT_3D('',#34098,#22055,#22056);
#18739=AXIS2_PLACEMENT_3D('',#34102,#22058,#22059);
#18740=AXIS2_PLACEMENT_3D('',#34103,#22060,#22061);
#18741=AXIS2_PLACEMENT_3D('',#34104,#22062,#22063);
#18742=AXIS2_PLACEMENT_3D('',#34106,#22065,#22066);
#18743=AXIS2_PLACEMENT_3D('',#34109,#22067,#22068);
#18744=AXIS2_PLACEMENT_3D('',#34110,#22069,#22070);
#18745=AXIS2_PLACEMENT_3D('',#34112,#22072,#22073);
#18746=AXIS2_PLACEMENT_3D('',#34115,#22074,#22075);
#18747=AXIS2_PLACEMENT_3D('',#34116,#22076,#22077);
#18748=AXIS2_PLACEMENT_3D('',#34120,#22079,#22080);
#18749=AXIS2_PLACEMENT_3D('',#34121,#22081,#22082);
#18750=AXIS2_PLACEMENT_3D('',#34122,#22083,#22084);
#18751=AXIS2_PLACEMENT_3D('',#34124,#22086,#22087);
#18752=AXIS2_PLACEMENT_3D('',#34127,#22088,#22089);
#18753=AXIS2_PLACEMENT_3D('',#34128,#22090,#22091);
#18754=AXIS2_PLACEMENT_3D('',#34130,#22093,#22094);
#18755=AXIS2_PLACEMENT_3D('',#34133,#22095,#22096);
#18756=AXIS2_PLACEMENT_3D('',#34134,#22097,#22098);
#18757=AXIS2_PLACEMENT_3D('',#34138,#22100,#22101);
#18758=AXIS2_PLACEMENT_3D('',#34139,#22102,#22103);
#18759=AXIS2_PLACEMENT_3D('',#34140,#22104,#22105);
#18760=AXIS2_PLACEMENT_3D('',#34142,#22107,#22108);
#18761=AXIS2_PLACEMENT_3D('',#34145,#22109,#22110);
#18762=AXIS2_PLACEMENT_3D('',#34146,#22111,#22112);
#18763=AXIS2_PLACEMENT_3D('',#34148,#22114,#22115);
#18764=AXIS2_PLACEMENT_3D('',#34151,#22116,#22117);
#18765=AXIS2_PLACEMENT_3D('',#34152,#22118,#22119);
#18766=AXIS2_PLACEMENT_3D('',#34156,#22121,#22122);
#18767=AXIS2_PLACEMENT_3D('',#34157,#22123,#22124);
#18768=AXIS2_PLACEMENT_3D('',#34158,#22125,#22126);
#18769=AXIS2_PLACEMENT_3D('',#34160,#22128,#22129);
#18770=AXIS2_PLACEMENT_3D('',#34163,#22130,#22131);
#18771=AXIS2_PLACEMENT_3D('',#34164,#22132,#22133);
#18772=AXIS2_PLACEMENT_3D('',#34166,#22135,#22136);
#18773=AXIS2_PLACEMENT_3D('',#34169,#22137,#22138);
#18774=AXIS2_PLACEMENT_3D('',#34170,#22139,#22140);
#18775=AXIS2_PLACEMENT_3D('',#34174,#22142,#22143);
#18776=AXIS2_PLACEMENT_3D('',#34175,#22144,#22145);
#18777=AXIS2_PLACEMENT_3D('',#34176,#22146,#22147);
#18778=AXIS2_PLACEMENT_3D('',#34178,#22149,#22150);
#18779=AXIS2_PLACEMENT_3D('',#34181,#22151,#22152);
#18780=AXIS2_PLACEMENT_3D('',#34182,#22153,#22154);
#18781=AXIS2_PLACEMENT_3D('',#34184,#22156,#22157);
#18782=AXIS2_PLACEMENT_3D('',#34187,#22158,#22159);
#18783=AXIS2_PLACEMENT_3D('',#34188,#22160,#22161);
#18784=AXIS2_PLACEMENT_3D('',#34192,#22163,#22164);
#18785=AXIS2_PLACEMENT_3D('',#34193,#22165,#22166);
#18786=AXIS2_PLACEMENT_3D('',#34194,#22167,#22168);
#18787=AXIS2_PLACEMENT_3D('',#34196,#22170,#22171);
#18788=AXIS2_PLACEMENT_3D('',#34199,#22172,#22173);
#18789=AXIS2_PLACEMENT_3D('',#34200,#22174,#22175);
#18790=AXIS2_PLACEMENT_3D('',#34202,#22177,#22178);
#18791=AXIS2_PLACEMENT_3D('',#34205,#22179,#22180);
#18792=AXIS2_PLACEMENT_3D('',#34206,#22181,#22182);
#18793=AXIS2_PLACEMENT_3D('',#34210,#22184,#22185);
#18794=AXIS2_PLACEMENT_3D('',#34211,#22186,#22187);
#18795=AXIS2_PLACEMENT_3D('',#34212,#22188,#22189);
#18796=AXIS2_PLACEMENT_3D('',#34214,#22191,#22192);
#18797=AXIS2_PLACEMENT_3D('',#34221,#22193,#22194);
#18798=AXIS2_PLACEMENT_3D('',#34231,#22195,#22196);
#18799=AXIS2_PLACEMENT_3D('',#34241,#22197,#22198);
#18800=AXIS2_PLACEMENT_3D('',#34251,#22199,#22200);
#18801=AXIS2_PLACEMENT_3D('',#34261,#22201,#22202);
#18802=AXIS2_PLACEMENT_3D('',#34271,#22203,#22204);
#18803=AXIS2_PLACEMENT_3D('',#34281,#22205,#22206);
#18804=AXIS2_PLACEMENT_3D('',#34291,#22207,#22208);
#18805=AXIS2_PLACEMENT_3D('',#34301,#22209,#22210);
#18806=AXIS2_PLACEMENT_3D('',#34311,#22211,#22212);
#18807=AXIS2_PLACEMENT_3D('',#34321,#22213,#22214);
#18808=AXIS2_PLACEMENT_3D('',#34331,#22215,#22216);
#18809=AXIS2_PLACEMENT_3D('',#34341,#22217,#22218);
#18810=AXIS2_PLACEMENT_3D('',#34351,#22219,#22220);
#18811=AXIS2_PLACEMENT_3D('',#34361,#22221,#22222);
#18812=AXIS2_PLACEMENT_3D('',#34371,#22223,#22224);
#18813=AXIS2_PLACEMENT_3D('',#34381,#22225,#22226);
#18814=AXIS2_PLACEMENT_3D('',#34391,#22227,#22228);
#18815=AXIS2_PLACEMENT_3D('',#34401,#22229,#22230);
#18816=AXIS2_PLACEMENT_3D('',#34411,#22231,#22232);
#18817=AXIS2_PLACEMENT_3D('',#34421,#22233,#22234);
#18818=AXIS2_PLACEMENT_3D('',#34431,#22235,#22236);
#18819=AXIS2_PLACEMENT_3D('',#34441,#22237,#22238);
#18820=AXIS2_PLACEMENT_3D('',#34451,#22239,#22240);
#18821=AXIS2_PLACEMENT_3D('',#34461,#22241,#22242);
#18822=AXIS2_PLACEMENT_3D('',#34471,#22243,#22244);
#18823=AXIS2_PLACEMENT_3D('',#34481,#22245,#22246);
#18824=AXIS2_PLACEMENT_3D('',#34491,#22247,#22248);
#18825=AXIS2_PLACEMENT_3D('',#34501,#22249,#22250);
#18826=AXIS2_PLACEMENT_3D('',#34511,#22251,#22252);
#18827=AXIS2_PLACEMENT_3D('',#34521,#22253,#22254);
#18828=AXIS2_PLACEMENT_3D('',#34531,#22255,#22256);
#18829=AXIS2_PLACEMENT_3D('',#34541,#22257,#22258);
#18830=AXIS2_PLACEMENT_3D('',#34551,#22259,#22260);
#18831=AXIS2_PLACEMENT_3D('',#34561,#22261,#22262);
#18832=AXIS2_PLACEMENT_3D('',#34571,#22263,#22264);
#18833=AXIS2_PLACEMENT_3D('',#34581,#22265,#22266);
#18834=AXIS2_PLACEMENT_3D('',#34591,#22267,#22268);
#18835=AXIS2_PLACEMENT_3D('',#34601,#22269,#22270);
#18836=AXIS2_PLACEMENT_3D('',#34608,#22272,#22273);
#18837=AXIS2_PLACEMENT_3D('',#34618,#22274,#22275);
#18838=AXIS2_PLACEMENT_3D('',#34628,#22276,#22277);
#18839=AXIS2_PLACEMENT_3D('',#34638,#22278,#22279);
#18840=AXIS2_PLACEMENT_3D('',#34648,#22280,#22281);
#18841=AXIS2_PLACEMENT_3D('',#34658,#22282,#22283);
#18842=AXIS2_PLACEMENT_3D('',#34668,#22284,#22285);
#18843=AXIS2_PLACEMENT_3D('',#34678,#22286,#22287);
#18844=AXIS2_PLACEMENT_3D('',#34688,#22288,#22289);
#18845=AXIS2_PLACEMENT_3D('',#34698,#22290,#22291);
#18846=AXIS2_PLACEMENT_3D('',#34708,#22292,#22293);
#18847=AXIS2_PLACEMENT_3D('',#34718,#22294,#22295);
#18848=AXIS2_PLACEMENT_3D('',#34728,#22296,#22297);
#18849=AXIS2_PLACEMENT_3D('',#34738,#22298,#22299);
#18850=AXIS2_PLACEMENT_3D('',#34748,#22300,#22301);
#18851=AXIS2_PLACEMENT_3D('',#34758,#22302,#22303);
#18852=AXIS2_PLACEMENT_3D('',#34768,#22304,#22305);
#18853=AXIS2_PLACEMENT_3D('',#34778,#22306,#22307);
#18854=AXIS2_PLACEMENT_3D('',#34788,#22308,#22309);
#18855=AXIS2_PLACEMENT_3D('',#34798,#22310,#22311);
#18856=AXIS2_PLACEMENT_3D('',#34808,#22312,#22313);
#18857=AXIS2_PLACEMENT_3D('',#34818,#22314,#22315);
#18858=AXIS2_PLACEMENT_3D('',#34828,#22316,#22317);
#18859=AXIS2_PLACEMENT_3D('',#34838,#22318,#22319);
#18860=AXIS2_PLACEMENT_3D('',#34848,#22320,#22321);
#18861=AXIS2_PLACEMENT_3D('',#34858,#22322,#22323);
#18862=AXIS2_PLACEMENT_3D('',#34868,#22324,#22325);
#18863=AXIS2_PLACEMENT_3D('',#34878,#22326,#22327);
#18864=AXIS2_PLACEMENT_3D('',#34888,#22328,#22329);
#18865=AXIS2_PLACEMENT_3D('',#34898,#22330,#22331);
#18866=AXIS2_PLACEMENT_3D('',#34908,#22332,#22333);
#18867=AXIS2_PLACEMENT_3D('',#34918,#22334,#22335);
#18868=AXIS2_PLACEMENT_3D('',#34928,#22336,#22337);
#18869=AXIS2_PLACEMENT_3D('',#34938,#22338,#22339);
#18870=AXIS2_PLACEMENT_3D('',#34948,#22340,#22341);
#18871=AXIS2_PLACEMENT_3D('',#34958,#22342,#22343);
#18872=AXIS2_PLACEMENT_3D('',#34968,#22344,#22345);
#18873=AXIS2_PLACEMENT_3D('',#34978,#22346,#22347);
#18874=AXIS2_PLACEMENT_3D('',#34988,#22348,#22349);
#18875=AXIS2_PLACEMENT_3D('',#34992,#22350,#22351);
#18876=AXIS2_PLACEMENT_3D('',#34999,#22352,#22353);
#18877=AXIS2_PLACEMENT_3D('',#35009,#22354,#22355);
#18878=AXIS2_PLACEMENT_3D('',#35019,#22356,#22357);
#18879=AXIS2_PLACEMENT_3D('',#35029,#22358,#22359);
#18880=AXIS2_PLACEMENT_3D('',#35039,#22360,#22361);
#18881=AXIS2_PLACEMENT_3D('',#35049,#22362,#22363);
#18882=AXIS2_PLACEMENT_3D('',#35059,#22364,#22365);
#18883=AXIS2_PLACEMENT_3D('',#35069,#22366,#22367);
#18884=AXIS2_PLACEMENT_3D('',#35079,#22368,#22369);
#18885=AXIS2_PLACEMENT_3D('',#35089,#22370,#22371);
#18886=AXIS2_PLACEMENT_3D('',#35099,#22372,#22373);
#18887=AXIS2_PLACEMENT_3D('',#35109,#22374,#22375);
#18888=AXIS2_PLACEMENT_3D('',#35119,#22376,#22377);
#18889=AXIS2_PLACEMENT_3D('',#35129,#22378,#22379);
#18890=AXIS2_PLACEMENT_3D('',#35139,#22380,#22381);
#18891=AXIS2_PLACEMENT_3D('',#35149,#22382,#22383);
#18892=AXIS2_PLACEMENT_3D('',#35159,#22384,#22385);
#18893=AXIS2_PLACEMENT_3D('',#35169,#22386,#22387);
#18894=AXIS2_PLACEMENT_3D('',#35179,#22388,#22389);
#18895=AXIS2_PLACEMENT_3D('',#35189,#22390,#22391);
#18896=AXIS2_PLACEMENT_3D('',#35199,#22392,#22393);
#18897=AXIS2_PLACEMENT_3D('',#35209,#22394,#22395);
#18898=AXIS2_PLACEMENT_3D('',#35219,#22396,#22397);
#18899=AXIS2_PLACEMENT_3D('',#35229,#22398,#22399);
#18900=AXIS2_PLACEMENT_3D('',#35239,#22400,#22401);
#18901=AXIS2_PLACEMENT_3D('',#35249,#22402,#22403);
#18902=AXIS2_PLACEMENT_3D('',#35259,#22404,#22405);
#18903=AXIS2_PLACEMENT_3D('',#35269,#22406,#22407);
#18904=AXIS2_PLACEMENT_3D('',#35279,#22408,#22409);
#18905=AXIS2_PLACEMENT_3D('',#35289,#22410,#22411);
#18906=AXIS2_PLACEMENT_3D('',#35299,#22412,#22413);
#18907=AXIS2_PLACEMENT_3D('',#35309,#22414,#22415);
#18908=AXIS2_PLACEMENT_3D('',#35319,#22416,#22417);
#18909=AXIS2_PLACEMENT_3D('',#35329,#22418,#22419);
#18910=AXIS2_PLACEMENT_3D('',#35339,#22420,#22421);
#18911=AXIS2_PLACEMENT_3D('',#35349,#22422,#22423);
#18912=AXIS2_PLACEMENT_3D('',#35359,#22424,#22425);
#18913=AXIS2_PLACEMENT_3D('',#35369,#22426,#22427);
#18914=AXIS2_PLACEMENT_3D('',#35379,#22428,#22429);
#18915=AXIS2_PLACEMENT_3D('',#35386,#22431,#22432);
#18916=AXIS2_PLACEMENT_3D('',#35396,#22433,#22434);
#18917=AXIS2_PLACEMENT_3D('',#35406,#22435,#22436);
#18918=AXIS2_PLACEMENT_3D('',#35416,#22437,#22438);
#18919=AXIS2_PLACEMENT_3D('',#35426,#22439,#22440);
#18920=AXIS2_PLACEMENT_3D('',#35436,#22441,#22442);
#18921=AXIS2_PLACEMENT_3D('',#35446,#22443,#22444);
#18922=AXIS2_PLACEMENT_3D('',#35456,#22445,#22446);
#18923=AXIS2_PLACEMENT_3D('',#35466,#22447,#22448);
#18924=AXIS2_PLACEMENT_3D('',#35476,#22449,#22450);
#18925=AXIS2_PLACEMENT_3D('',#35486,#22451,#22452);
#18926=AXIS2_PLACEMENT_3D('',#35496,#22453,#22454);
#18927=AXIS2_PLACEMENT_3D('',#35506,#22455,#22456);
#18928=AXIS2_PLACEMENT_3D('',#35516,#22457,#22458);
#18929=AXIS2_PLACEMENT_3D('',#35526,#22459,#22460);
#18930=AXIS2_PLACEMENT_3D('',#35536,#22461,#22462);
#18931=AXIS2_PLACEMENT_3D('',#35546,#22463,#22464);
#18932=AXIS2_PLACEMENT_3D('',#35556,#22465,#22466);
#18933=AXIS2_PLACEMENT_3D('',#35566,#22467,#22468);
#18934=AXIS2_PLACEMENT_3D('',#35576,#22469,#22470);
#18935=AXIS2_PLACEMENT_3D('',#35586,#22471,#22472);
#18936=AXIS2_PLACEMENT_3D('',#35596,#22473,#22474);
#18937=AXIS2_PLACEMENT_3D('',#35606,#22475,#22476);
#18938=AXIS2_PLACEMENT_3D('',#35616,#22477,#22478);
#18939=AXIS2_PLACEMENT_3D('',#35626,#22479,#22480);
#18940=AXIS2_PLACEMENT_3D('',#35636,#22481,#22482);
#18941=AXIS2_PLACEMENT_3D('',#35646,#22483,#22484);
#18942=AXIS2_PLACEMENT_3D('',#35656,#22485,#22486);
#18943=AXIS2_PLACEMENT_3D('',#35666,#22487,#22488);
#18944=AXIS2_PLACEMENT_3D('',#35676,#22489,#22490);
#18945=AXIS2_PLACEMENT_3D('',#35686,#22491,#22492);
#18946=AXIS2_PLACEMENT_3D('',#35696,#22493,#22494);
#18947=AXIS2_PLACEMENT_3D('',#35706,#22495,#22496);
#18948=AXIS2_PLACEMENT_3D('',#35716,#22497,#22498);
#18949=AXIS2_PLACEMENT_3D('',#35726,#22499,#22500);
#18950=AXIS2_PLACEMENT_3D('',#35736,#22501,#22502);
#18951=AXIS2_PLACEMENT_3D('',#35746,#22503,#22504);
#18952=AXIS2_PLACEMENT_3D('',#35756,#22505,#22506);
#18953=AXIS2_PLACEMENT_3D('',#35766,#22507,#22508);
#18954=AXIS2_PLACEMENT_3D('',#35770,#22509,#22510);
#18955=AXIS2_PLACEMENT_3D('',#35772,#22512,#22513);
#18956=AXIS2_PLACEMENT_3D('',#35775,#22516,#22517);
#18957=AXIS2_PLACEMENT_3D('',#35778,#22520,#22521);
#18958=AXIS2_PLACEMENT_3D('',#35781,#22524,#22525);
#18959=AXIS2_PLACEMENT_3D('',#35784,#22528,#22529);
#18960=AXIS2_PLACEMENT_3D('',#35787,#22532,#22533);
#18961=AXIS2_PLACEMENT_3D('',#35790,#22536,#22537);
#18962=AXIS2_PLACEMENT_3D('',#35793,#22540,#22541);
#18963=AXIS2_PLACEMENT_3D('',#35796,#22544,#22545);
#18964=AXIS2_PLACEMENT_3D('',#35799,#22548,#22549);
#18965=AXIS2_PLACEMENT_3D('',#35802,#22552,#22553);
#18966=AXIS2_PLACEMENT_3D('',#35805,#22556,#22557);
#18967=AXIS2_PLACEMENT_3D('',#35808,#22560,#22561);
#18968=AXIS2_PLACEMENT_3D('',#35811,#22564,#22565);
#18969=AXIS2_PLACEMENT_3D('',#35814,#22568,#22569);
#18970=AXIS2_PLACEMENT_3D('',#35817,#22572,#22573);
#18971=AXIS2_PLACEMENT_3D('',#35820,#22576,#22577);
#18972=AXIS2_PLACEMENT_3D('',#35823,#22580,#22581);
#18973=AXIS2_PLACEMENT_3D('',#35826,#22584,#22585);
#18974=AXIS2_PLACEMENT_3D('',#35829,#22588,#22589);
#18975=AXIS2_PLACEMENT_3D('',#35832,#22592,#22593);
#18976=AXIS2_PLACEMENT_3D('',#35835,#22596,#22597);
#18977=AXIS2_PLACEMENT_3D('',#35838,#22600,#22601);
#18978=AXIS2_PLACEMENT_3D('',#35841,#22604,#22605);
#18979=AXIS2_PLACEMENT_3D('',#35844,#22608,#22609);
#18980=AXIS2_PLACEMENT_3D('',#35847,#22612,#22613);
#18981=AXIS2_PLACEMENT_3D('',#35850,#22616,#22617);
#18982=AXIS2_PLACEMENT_3D('',#35853,#22620,#22621);
#18983=AXIS2_PLACEMENT_3D('',#35856,#22624,#22625);
#18984=AXIS2_PLACEMENT_3D('',#35859,#22628,#22629);
#18985=AXIS2_PLACEMENT_3D('',#35862,#22632,#22633);
#18986=AXIS2_PLACEMENT_3D('',#35865,#22636,#22637);
#18987=AXIS2_PLACEMENT_3D('',#35868,#22640,#22641);
#18988=AXIS2_PLACEMENT_3D('',#35871,#22644,#22645);
#18989=AXIS2_PLACEMENT_3D('',#35874,#22648,#22649);
#18990=AXIS2_PLACEMENT_3D('',#35877,#22652,#22653);
#18991=AXIS2_PLACEMENT_3D('',#35880,#22656,#22657);
#18992=AXIS2_PLACEMENT_3D('',#35883,#22660,#22661);
#18993=AXIS2_PLACEMENT_3D('',#35886,#22664,#22665);
#18994=AXIS2_PLACEMENT_3D('',#35889,#22668,#22669);
#18995=AXIS2_PLACEMENT_3D('',#35892,#22672,#22673);
#18996=AXIS2_PLACEMENT_3D('',#35895,#22676,#22677);
#18997=AXIS2_PLACEMENT_3D('',#35898,#22680,#22681);
#18998=AXIS2_PLACEMENT_3D('',#35901,#22684,#22685);
#18999=AXIS2_PLACEMENT_3D('',#35904,#22688,#22689);
#19000=AXIS2_PLACEMENT_3D('',#35907,#22692,#22693);
#19001=AXIS2_PLACEMENT_3D('',#35910,#22696,#22697);
#19002=AXIS2_PLACEMENT_3D('',#35913,#22700,#22701);
#19003=AXIS2_PLACEMENT_3D('',#35916,#22704,#22705);
#19004=AXIS2_PLACEMENT_3D('',#35919,#22708,#22709);
#19005=AXIS2_PLACEMENT_3D('',#35922,#22712,#22713);
#19006=AXIS2_PLACEMENT_3D('',#35925,#22716,#22717);
#19007=AXIS2_PLACEMENT_3D('',#35928,#22720,#22721);
#19008=AXIS2_PLACEMENT_3D('',#35931,#22724,#22725);
#19009=AXIS2_PLACEMENT_3D('',#35934,#22728,#22729);
#19010=AXIS2_PLACEMENT_3D('',#35937,#22732,#22733);
#19011=AXIS2_PLACEMENT_3D('',#35940,#22736,#22737);
#19012=AXIS2_PLACEMENT_3D('',#35943,#22740,#22741);
#19013=AXIS2_PLACEMENT_3D('',#35946,#22744,#22745);
#19014=AXIS2_PLACEMENT_3D('',#35949,#22748,#22749);
#19015=AXIS2_PLACEMENT_3D('',#35952,#22752,#22753);
#19016=AXIS2_PLACEMENT_3D('',#35955,#22756,#22757);
#19017=AXIS2_PLACEMENT_3D('',#35958,#22760,#22761);
#19018=AXIS2_PLACEMENT_3D('',#35961,#22764,#22765);
#19019=AXIS2_PLACEMENT_3D('',#35964,#22768,#22769);
#19020=AXIS2_PLACEMENT_3D('',#35967,#22772,#22773);
#19021=AXIS2_PLACEMENT_3D('',#35970,#22776,#22777);
#19022=AXIS2_PLACEMENT_3D('',#35973,#22780,#22781);
#19023=AXIS2_PLACEMENT_3D('',#35976,#22784,#22785);
#19024=AXIS2_PLACEMENT_3D('',#35979,#22788,#22789);
#19025=AXIS2_PLACEMENT_3D('',#35982,#22792,#22793);
#19026=AXIS2_PLACEMENT_3D('',#35985,#22796,#22797);
#19027=AXIS2_PLACEMENT_3D('',#35988,#22800,#22801);
#19028=AXIS2_PLACEMENT_3D('',#35991,#22804,#22805);
#19029=AXIS2_PLACEMENT_3D('',#35994,#22808,#22809);
#19030=AXIS2_PLACEMENT_3D('',#35997,#22812,#22813);
#19031=AXIS2_PLACEMENT_3D('',#36000,#22816,#22817);
#19032=AXIS2_PLACEMENT_3D('',#36001,#22818,#22819);
#19033=AXIS2_PLACEMENT_3D('',#36004,#22822,#22823);
#19034=AXIS2_PLACEMENT_3D('',#36005,#22824,#22825);
#19035=AXIS2_PLACEMENT_3D('',#36006,#22826,#22827);
#19036=AXIS2_PLACEMENT_3D('',#36008,#22829,#22830);
#19037=AXIS2_PLACEMENT_3D('',#36009,#22831,#22832);
#19038=AXIS2_PLACEMENT_3D('',#36011,#22834,#22835);
#19039=AXIS2_PLACEMENT_3D('',#36012,#22836,#22837);
#19040=AXIS2_PLACEMENT_3D('',#36014,#22839,#22840);
#19041=AXIS2_PLACEMENT_3D('',#36015,#22841,#22842);
#19042=AXIS2_PLACEMENT_3D('',#36017,#22844,#22845);
#19043=AXIS2_PLACEMENT_3D('',#36018,#22846,#22847);
#19044=AXIS2_PLACEMENT_3D('',#36020,#22849,#22850);
#19045=AXIS2_PLACEMENT_3D('',#36021,#22851,#22852);
#19046=AXIS2_PLACEMENT_3D('',#36023,#22854,#22855);
#19047=AXIS2_PLACEMENT_3D('',#36024,#22856,#22857);
#19048=AXIS2_PLACEMENT_3D('',#36026,#22859,#22860);
#19049=AXIS2_PLACEMENT_3D('',#36027,#22861,#22862);
#19050=AXIS2_PLACEMENT_3D('',#36029,#22864,#22865);
#19051=AXIS2_PLACEMENT_3D('',#36030,#22866,#22867);
#19052=AXIS2_PLACEMENT_3D('',#36032,#22869,#22870);
#19053=AXIS2_PLACEMENT_3D('',#36033,#22871,#22872);
#19054=AXIS2_PLACEMENT_3D('',#36035,#22874,#22875);
#19055=AXIS2_PLACEMENT_3D('',#36036,#22876,#22877);
#19056=AXIS2_PLACEMENT_3D('',#36038,#22879,#22880);
#19057=AXIS2_PLACEMENT_3D('',#36039,#22881,#22882);
#19058=AXIS2_PLACEMENT_3D('',#36041,#22884,#22885);
#19059=AXIS2_PLACEMENT_3D('',#36042,#22886,#22887);
#19060=AXIS2_PLACEMENT_3D('',#36044,#22889,#22890);
#19061=AXIS2_PLACEMENT_3D('',#36045,#22891,#22892);
#19062=AXIS2_PLACEMENT_3D('',#36047,#22894,#22895);
#19063=AXIS2_PLACEMENT_3D('',#36048,#22896,#22897);
#19064=AXIS2_PLACEMENT_3D('',#36050,#22899,#22900);
#19065=AXIS2_PLACEMENT_3D('',#36051,#22901,#22902);
#19066=AXIS2_PLACEMENT_3D('',#36053,#22904,#22905);
#19067=AXIS2_PLACEMENT_3D('',#36054,#22906,#22907);
#19068=AXIS2_PLACEMENT_3D('',#36056,#22909,#22910);
#19069=AXIS2_PLACEMENT_3D('',#36057,#22911,#22912);
#19070=AXIS2_PLACEMENT_3D('',#36059,#22914,#22915);
#19071=AXIS2_PLACEMENT_3D('',#36060,#22916,#22917);
#19072=AXIS2_PLACEMENT_3D('',#36062,#22919,#22920);
#19073=AXIS2_PLACEMENT_3D('',#36063,#22921,#22922);
#19074=AXIS2_PLACEMENT_3D('',#36065,#22924,#22925);
#19075=AXIS2_PLACEMENT_3D('',#36066,#22926,#22927);
#19076=AXIS2_PLACEMENT_3D('',#36068,#22929,#22930);
#19077=AXIS2_PLACEMENT_3D('',#36069,#22931,#22932);
#19078=AXIS2_PLACEMENT_3D('',#36071,#22934,#22935);
#19079=AXIS2_PLACEMENT_3D('',#36072,#22936,#22937);
#19080=AXIS2_PLACEMENT_3D('',#36074,#22939,#22940);
#19081=AXIS2_PLACEMENT_3D('',#36075,#22941,#22942);
#19082=AXIS2_PLACEMENT_3D('',#36077,#22944,#22945);
#19083=AXIS2_PLACEMENT_3D('',#36078,#22946,#22947);
#19084=AXIS2_PLACEMENT_3D('',#36080,#22949,#22950);
#19085=AXIS2_PLACEMENT_3D('',#36081,#22951,#22952);
#19086=AXIS2_PLACEMENT_3D('',#36083,#22954,#22955);
#19087=AXIS2_PLACEMENT_3D('',#36084,#22956,#22957);
#19088=AXIS2_PLACEMENT_3D('',#36086,#22959,#22960);
#19089=AXIS2_PLACEMENT_3D('',#36087,#22961,#22962);
#19090=AXIS2_PLACEMENT_3D('',#36089,#22964,#22965);
#19091=AXIS2_PLACEMENT_3D('',#36090,#22966,#22967);
#19092=AXIS2_PLACEMENT_3D('',#36092,#22969,#22970);
#19093=AXIS2_PLACEMENT_3D('',#36093,#22971,#22972);
#19094=AXIS2_PLACEMENT_3D('',#36095,#22974,#22975);
#19095=AXIS2_PLACEMENT_3D('',#36096,#22976,#22977);
#19096=AXIS2_PLACEMENT_3D('',#36098,#22979,#22980);
#19097=AXIS2_PLACEMENT_3D('',#36099,#22981,#22982);
#19098=AXIS2_PLACEMENT_3D('',#36101,#22984,#22985);
#19099=AXIS2_PLACEMENT_3D('',#36102,#22986,#22987);
#19100=AXIS2_PLACEMENT_3D('',#36104,#22989,#22990);
#19101=AXIS2_PLACEMENT_3D('',#36105,#22991,#22992);
#19102=AXIS2_PLACEMENT_3D('',#36107,#22994,#22995);
#19103=AXIS2_PLACEMENT_3D('',#36108,#22996,#22997);
#19104=AXIS2_PLACEMENT_3D('',#36110,#22999,#23000);
#19105=AXIS2_PLACEMENT_3D('',#36111,#23001,#23002);
#19106=AXIS2_PLACEMENT_3D('',#36113,#23004,#23005);
#19107=AXIS2_PLACEMENT_3D('',#36114,#23006,#23007);
#19108=AXIS2_PLACEMENT_3D('',#36116,#23009,#23010);
#19109=AXIS2_PLACEMENT_3D('',#36117,#23011,#23012);
#19110=AXIS2_PLACEMENT_3D('',#36119,#23014,#23015);
#19111=AXIS2_PLACEMENT_3D('',#36120,#23016,#23017);
#19112=AXIS2_PLACEMENT_3D('',#36122,#23019,#23020);
#19113=AXIS2_PLACEMENT_3D('',#36123,#23021,#23022);
#19114=AXIS2_PLACEMENT_3D('',#36125,#23024,#23025);
#19115=AXIS2_PLACEMENT_3D('',#36126,#23026,#23027);
#19116=AXIS2_PLACEMENT_3D('',#36128,#23029,#23030);
#19117=AXIS2_PLACEMENT_3D('',#36129,#23031,#23032);
#19118=AXIS2_PLACEMENT_3D('',#36131,#23034,#23035);
#19119=AXIS2_PLACEMENT_3D('',#36132,#23036,#23037);
#19120=AXIS2_PLACEMENT_3D('',#36134,#23039,#23040);
#19121=AXIS2_PLACEMENT_3D('',#36135,#23041,#23042);
#19122=AXIS2_PLACEMENT_3D('',#36137,#23044,#23045);
#19123=AXIS2_PLACEMENT_3D('',#36138,#23046,#23047);
#19124=AXIS2_PLACEMENT_3D('',#36140,#23049,#23050);
#19125=AXIS2_PLACEMENT_3D('',#36141,#23051,#23052);
#19126=AXIS2_PLACEMENT_3D('',#36143,#23054,#23055);
#19127=AXIS2_PLACEMENT_3D('',#36144,#23056,#23057);
#19128=AXIS2_PLACEMENT_3D('',#36146,#23059,#23060);
#19129=AXIS2_PLACEMENT_3D('',#36147,#23061,#23062);
#19130=AXIS2_PLACEMENT_3D('',#36149,#23064,#23065);
#19131=AXIS2_PLACEMENT_3D('',#36150,#23066,#23067);
#19132=AXIS2_PLACEMENT_3D('',#36152,#23069,#23070);
#19133=AXIS2_PLACEMENT_3D('',#36153,#23071,#23072);
#19134=AXIS2_PLACEMENT_3D('',#36155,#23074,#23075);
#19135=AXIS2_PLACEMENT_3D('',#36156,#23076,#23077);
#19136=AXIS2_PLACEMENT_3D('',#36158,#23079,#23080);
#19137=AXIS2_PLACEMENT_3D('',#36159,#23081,#23082);
#19138=AXIS2_PLACEMENT_3D('',#36161,#23084,#23085);
#19139=AXIS2_PLACEMENT_3D('',#36162,#23086,#23087);
#19140=AXIS2_PLACEMENT_3D('',#36164,#23089,#23090);
#19141=AXIS2_PLACEMENT_3D('',#36165,#23091,#23092);
#19142=AXIS2_PLACEMENT_3D('',#36167,#23094,#23095);
#19143=AXIS2_PLACEMENT_3D('',#36168,#23096,#23097);
#19144=AXIS2_PLACEMENT_3D('',#36170,#23099,#23100);
#19145=AXIS2_PLACEMENT_3D('',#36171,#23101,#23102);
#19146=AXIS2_PLACEMENT_3D('',#36173,#23104,#23105);
#19147=AXIS2_PLACEMENT_3D('',#36174,#23106,#23107);
#19148=AXIS2_PLACEMENT_3D('',#36176,#23109,#23110);
#19149=AXIS2_PLACEMENT_3D('',#36177,#23111,#23112);
#19150=AXIS2_PLACEMENT_3D('',#36179,#23114,#23115);
#19151=AXIS2_PLACEMENT_3D('',#36180,#23116,#23117);
#19152=AXIS2_PLACEMENT_3D('',#36182,#23119,#23120);
#19153=AXIS2_PLACEMENT_3D('',#36183,#23121,#23122);
#19154=AXIS2_PLACEMENT_3D('',#36185,#23124,#23125);
#19155=AXIS2_PLACEMENT_3D('',#36186,#23126,#23127);
#19156=AXIS2_PLACEMENT_3D('',#36188,#23129,#23130);
#19157=AXIS2_PLACEMENT_3D('',#36189,#23131,#23132);
#19158=AXIS2_PLACEMENT_3D('',#36191,#23134,#23135);
#19159=AXIS2_PLACEMENT_3D('',#36192,#23136,#23137);
#19160=AXIS2_PLACEMENT_3D('',#36194,#23139,#23140);
#19161=AXIS2_PLACEMENT_3D('',#36195,#23141,#23142);
#19162=AXIS2_PLACEMENT_3D('',#36197,#23144,#23145);
#19163=AXIS2_PLACEMENT_3D('',#36198,#23146,#23147);
#19164=AXIS2_PLACEMENT_3D('',#36200,#23149,#23150);
#19165=AXIS2_PLACEMENT_3D('',#36201,#23151,#23152);
#19166=AXIS2_PLACEMENT_3D('',#36203,#23154,#23155);
#19167=AXIS2_PLACEMENT_3D('',#36204,#23156,#23157);
#19168=AXIS2_PLACEMENT_3D('',#36206,#23159,#23160);
#19169=AXIS2_PLACEMENT_3D('',#36207,#23161,#23162);
#19170=AXIS2_PLACEMENT_3D('',#36209,#23164,#23165);
#19171=AXIS2_PLACEMENT_3D('',#36210,#23166,#23167);
#19172=AXIS2_PLACEMENT_3D('',#36212,#23169,#23170);
#19173=AXIS2_PLACEMENT_3D('',#36213,#23171,#23172);
#19174=AXIS2_PLACEMENT_3D('',#36215,#23174,#23175);
#19175=AXIS2_PLACEMENT_3D('',#36216,#23176,#23177);
#19176=AXIS2_PLACEMENT_3D('',#36218,#23179,#23180);
#19177=AXIS2_PLACEMENT_3D('',#36219,#23181,#23182);
#19178=AXIS2_PLACEMENT_3D('',#36221,#23184,#23185);
#19179=AXIS2_PLACEMENT_3D('',#36222,#23186,#23187);
#19180=AXIS2_PLACEMENT_3D('',#36224,#23189,#23190);
#19181=AXIS2_PLACEMENT_3D('',#36225,#23191,#23192);
#19182=AXIS2_PLACEMENT_3D('',#36227,#23194,#23195);
#19183=AXIS2_PLACEMENT_3D('',#36228,#23196,#23197);
#19184=AXIS2_PLACEMENT_3D('',#36230,#23199,#23200);
#19185=AXIS2_PLACEMENT_3D('',#36231,#23201,#23202);
#19186=AXIS2_PLACEMENT_3D('',#36233,#23204,#23205);
#19187=AXIS2_PLACEMENT_3D('',#36234,#23206,#23207);
#19188=AXIS2_PLACEMENT_3D('',#36236,#23209,#23210);
#19189=AXIS2_PLACEMENT_3D('',#36237,#23211,#23212);
#19190=AXIS2_PLACEMENT_3D('',#36240,#23213,#23214);
#19191=AXIS2_PLACEMENT_3D('',#36253,#23215,#23216);
#19192=AXIS2_PLACEMENT_3D('',#36266,#23217,#23218);
#19193=AXIS2_PLACEMENT_3D('',#36268,#23219,#23220);
#19194=AXIS2_PLACEMENT_3D('',#36270,#23221,#23222);
#19195=AXIS2_PLACEMENT_3D('',#36271,#23223,#23224);
#19196=AXIS2_PLACEMENT_3D('',#36273,#23225,#23226);
#19197=AXIS2_PLACEMENT_3D('',#36286,#23227,#23228);
#19198=AXIS2_PLACEMENT_3D('',#36297,#23229,#23230);
#19199=AXIS2_PLACEMENT_3D('',#36299,#23231,#23232);
#19200=AXIS2_PLACEMENT_3D('',#36301,#23234,#23235);
#19201=AXIS2_PLACEMENT_3D('',#36303,#23236,#23237);
#19202=AXIS2_PLACEMENT_3D('',#36306,#23239,#23240);
#19203=AXIS2_PLACEMENT_3D('',#36307,#23241,#23242);
#19204=AXIS2_PLACEMENT_3D('',#36309,#23244,#23245);
#19205=AXIS2_PLACEMENT_3D('',#36310,#23246,#23247);
#19206=AXIS2_PLACEMENT_3D('',#36312,#23249,#23250);
#19207=AXIS2_PLACEMENT_3D('',#36313,#23251,#23252);
#19208=AXIS2_PLACEMENT_3D('',#36315,#23254,#23255);
#19209=AXIS2_PLACEMENT_3D('',#36317,#23257,#23258);
#19210=AXIS2_PLACEMENT_3D('',#36318,#23259,#23260);
#19211=AXIS2_PLACEMENT_3D('',#36320,#23261,#23262);
#19212=AXIS2_PLACEMENT_3D('',#36322,#23263,#23264);
#19213=AXIS2_PLACEMENT_3D('',#36323,#23265,#23266);
#19214=AXIS2_PLACEMENT_3D('',#36324,#23267,#23268);
#19215=AXIS2_PLACEMENT_3D('',#36327,#23269,#23270);
#19216=AXIS2_PLACEMENT_3D('',#36328,#23271,#23272);
#19217=AXIS2_PLACEMENT_3D('',#36331,#23274,#23275);
#19218=AXIS2_PLACEMENT_3D('',#36332,#23276,#23277);
#19219=AXIS2_PLACEMENT_3D('',#36335,#23278,#23279);
#19220=AXIS2_PLACEMENT_3D('',#36336,#23280,#23281);
#19221=AXIS2_PLACEMENT_3D('',#36340,#23283,#23284);
#19222=AXIS2_PLACEMENT_3D('',#36341,#23285,#23286);
#19223=AXIS2_PLACEMENT_3D('',#36342,#23287,#23288);
#19224=AXIS2_PLACEMENT_3D('',#36344,#23290,#23291);
#19225=AXIS2_PLACEMENT_3D('',#36347,#23292,#23293);
#19226=AXIS2_PLACEMENT_3D('',#36348,#23294,#23295);
#19227=AXIS2_PLACEMENT_3D('',#36350,#23297,#23298);
#19228=AXIS2_PLACEMENT_3D('',#36353,#23299,#23300);
#19229=AXIS2_PLACEMENT_3D('',#36354,#23301,#23302);
#19230=AXIS2_PLACEMENT_3D('',#36358,#23304,#23305);
#19231=AXIS2_PLACEMENT_3D('',#36359,#23306,#23307);
#19232=AXIS2_PLACEMENT_3D('',#36360,#23308,#23309);
#19233=AXIS2_PLACEMENT_3D('',#36362,#23311,#23312);
#19234=AXIS2_PLACEMENT_3D('',#36365,#23313,#23314);
#19235=AXIS2_PLACEMENT_3D('',#36366,#23315,#23316);
#19236=AXIS2_PLACEMENT_3D('',#36368,#23318,#23319);
#19237=AXIS2_PLACEMENT_3D('',#36371,#23320,#23321);
#19238=AXIS2_PLACEMENT_3D('',#36372,#23322,#23323);
#19239=AXIS2_PLACEMENT_3D('',#36376,#23325,#23326);
#19240=AXIS2_PLACEMENT_3D('',#36377,#23327,#23328);
#19241=AXIS2_PLACEMENT_3D('',#36378,#23329,#23330);
#19242=AXIS2_PLACEMENT_3D('',#36380,#23332,#23333);
#19243=AXIS2_PLACEMENT_3D('',#36383,#23334,#23335);
#19244=AXIS2_PLACEMENT_3D('',#36384,#23336,#23337);
#19245=AXIS2_PLACEMENT_3D('',#36386,#23339,#23340);
#19246=AXIS2_PLACEMENT_3D('',#36389,#23341,#23342);
#19247=AXIS2_PLACEMENT_3D('',#36390,#23343,#23344);
#19248=AXIS2_PLACEMENT_3D('',#36394,#23346,#23347);
#19249=AXIS2_PLACEMENT_3D('',#36395,#23348,#23349);
#19250=AXIS2_PLACEMENT_3D('',#36396,#23350,#23351);
#19251=AXIS2_PLACEMENT_3D('',#36398,#23353,#23354);
#19252=AXIS2_PLACEMENT_3D('',#36401,#23355,#23356);
#19253=AXIS2_PLACEMENT_3D('',#36402,#23357,#23358);
#19254=AXIS2_PLACEMENT_3D('',#36404,#23360,#23361);
#19255=AXIS2_PLACEMENT_3D('',#36407,#23362,#23363);
#19256=AXIS2_PLACEMENT_3D('',#36408,#23364,#23365);
#19257=AXIS2_PLACEMENT_3D('',#36412,#23367,#23368);
#19258=AXIS2_PLACEMENT_3D('',#36413,#23369,#23370);
#19259=AXIS2_PLACEMENT_3D('',#36414,#23371,#23372);
#19260=AXIS2_PLACEMENT_3D('',#36416,#23374,#23375);
#19261=AXIS2_PLACEMENT_3D('',#36419,#23376,#23377);
#19262=AXIS2_PLACEMENT_3D('',#36420,#23378,#23379);
#19263=AXIS2_PLACEMENT_3D('',#36422,#23381,#23382);
#19264=AXIS2_PLACEMENT_3D('',#36425,#23383,#23384);
#19265=AXIS2_PLACEMENT_3D('',#36426,#23385,#23386);
#19266=AXIS2_PLACEMENT_3D('',#36430,#23388,#23389);
#19267=AXIS2_PLACEMENT_3D('',#36431,#23390,#23391);
#19268=AXIS2_PLACEMENT_3D('',#36432,#23392,#23393);
#19269=AXIS2_PLACEMENT_3D('',#36434,#23395,#23396);
#19270=AXIS2_PLACEMENT_3D('',#36437,#23397,#23398);
#19271=AXIS2_PLACEMENT_3D('',#36438,#23399,#23400);
#19272=AXIS2_PLACEMENT_3D('',#36440,#23402,#23403);
#19273=AXIS2_PLACEMENT_3D('',#36443,#23404,#23405);
#19274=AXIS2_PLACEMENT_3D('',#36444,#23406,#23407);
#19275=AXIS2_PLACEMENT_3D('',#36448,#23409,#23410);
#19276=AXIS2_PLACEMENT_3D('',#36449,#23411,#23412);
#19277=AXIS2_PLACEMENT_3D('',#36450,#23413,#23414);
#19278=AXIS2_PLACEMENT_3D('',#36452,#23416,#23417);
#19279=AXIS2_PLACEMENT_3D('',#36455,#23418,#23419);
#19280=AXIS2_PLACEMENT_3D('',#36456,#23420,#23421);
#19281=AXIS2_PLACEMENT_3D('',#36458,#23423,#23424);
#19282=AXIS2_PLACEMENT_3D('',#36461,#23425,#23426);
#19283=AXIS2_PLACEMENT_3D('',#36462,#23427,#23428);
#19284=AXIS2_PLACEMENT_3D('',#36466,#23430,#23431);
#19285=AXIS2_PLACEMENT_3D('',#36467,#23432,#23433);
#19286=AXIS2_PLACEMENT_3D('',#36468,#23434,#23435);
#19287=AXIS2_PLACEMENT_3D('',#36470,#23437,#23438);
#19288=AXIS2_PLACEMENT_3D('',#36473,#23439,#23440);
#19289=AXIS2_PLACEMENT_3D('',#36474,#23441,#23442);
#19290=AXIS2_PLACEMENT_3D('',#36476,#23444,#23445);
#19291=AXIS2_PLACEMENT_3D('',#36479,#23446,#23447);
#19292=AXIS2_PLACEMENT_3D('',#36480,#23448,#23449);
#19293=AXIS2_PLACEMENT_3D('',#36484,#23451,#23452);
#19294=AXIS2_PLACEMENT_3D('',#36485,#23453,#23454);
#19295=AXIS2_PLACEMENT_3D('',#36486,#23455,#23456);
#19296=AXIS2_PLACEMENT_3D('',#36488,#23458,#23459);
#19297=AXIS2_PLACEMENT_3D('',#36491,#23460,#23461);
#19298=AXIS2_PLACEMENT_3D('',#36492,#23462,#23463);
#19299=AXIS2_PLACEMENT_3D('',#36494,#23465,#23466);
#19300=AXIS2_PLACEMENT_3D('',#36497,#23467,#23468);
#19301=AXIS2_PLACEMENT_3D('',#36498,#23469,#23470);
#19302=AXIS2_PLACEMENT_3D('',#36502,#23472,#23473);
#19303=AXIS2_PLACEMENT_3D('',#36503,#23474,#23475);
#19304=AXIS2_PLACEMENT_3D('',#36504,#23476,#23477);
#19305=AXIS2_PLACEMENT_3D('',#36506,#23479,#23480);
#19306=AXIS2_PLACEMENT_3D('',#36509,#23481,#23482);
#19307=AXIS2_PLACEMENT_3D('',#36510,#23483,#23484);
#19308=AXIS2_PLACEMENT_3D('',#36512,#23486,#23487);
#19309=AXIS2_PLACEMENT_3D('',#36515,#23488,#23489);
#19310=AXIS2_PLACEMENT_3D('',#36516,#23490,#23491);
#19311=AXIS2_PLACEMENT_3D('',#36520,#23493,#23494);
#19312=AXIS2_PLACEMENT_3D('',#36521,#23495,#23496);
#19313=AXIS2_PLACEMENT_3D('',#36522,#23497,#23498);
#19314=AXIS2_PLACEMENT_3D('',#36524,#23500,#23501);
#19315=AXIS2_PLACEMENT_3D('',#36527,#23502,#23503);
#19316=AXIS2_PLACEMENT_3D('',#36528,#23504,#23505);
#19317=AXIS2_PLACEMENT_3D('',#36530,#23507,#23508);
#19318=AXIS2_PLACEMENT_3D('',#36533,#23509,#23510);
#19319=AXIS2_PLACEMENT_3D('',#36534,#23511,#23512);
#19320=AXIS2_PLACEMENT_3D('',#36538,#23514,#23515);
#19321=AXIS2_PLACEMENT_3D('',#36539,#23516,#23517);
#19322=AXIS2_PLACEMENT_3D('',#36540,#23518,#23519);
#19323=AXIS2_PLACEMENT_3D('',#36542,#23521,#23522);
#19324=AXIS2_PLACEMENT_3D('',#36545,#23523,#23524);
#19325=AXIS2_PLACEMENT_3D('',#36546,#23525,#23526);
#19326=AXIS2_PLACEMENT_3D('',#36548,#23528,#23529);
#19327=AXIS2_PLACEMENT_3D('',#36551,#23530,#23531);
#19328=AXIS2_PLACEMENT_3D('',#36552,#23532,#23533);
#19329=AXIS2_PLACEMENT_3D('',#36556,#23535,#23536);
#19330=AXIS2_PLACEMENT_3D('',#36557,#23537,#23538);
#19331=AXIS2_PLACEMENT_3D('',#36558,#23539,#23540);
#19332=AXIS2_PLACEMENT_3D('',#36560,#23542,#23543);
#19333=AXIS2_PLACEMENT_3D('',#36563,#23545,#23546);
#19334=AXIS2_PLACEMENT_3D('',#36564,#23547,#23548);
#19335=AXIS2_PLACEMENT_3D('',#36571,#23549,#23550);
#19336=AXIS2_PLACEMENT_3D('',#36581,#23551,#23552);
#19337=AXIS2_PLACEMENT_3D('',#36591,#23553,#23554);
#19338=AXIS2_PLACEMENT_3D('',#36601,#23555,#23556);
#19339=AXIS2_PLACEMENT_3D('',#36611,#23557,#23558);
#19340=AXIS2_PLACEMENT_3D('',#36621,#23559,#23560);
#19341=AXIS2_PLACEMENT_3D('',#36631,#23561,#23562);
#19342=AXIS2_PLACEMENT_3D('',#36641,#23563,#23564);
#19343=AXIS2_PLACEMENT_3D('',#36651,#23565,#23566);
#19344=AXIS2_PLACEMENT_3D('',#36661,#23567,#23568);
#19345=AXIS2_PLACEMENT_3D('',#36671,#23569,#23570);
#19346=AXIS2_PLACEMENT_3D('',#36681,#23571,#23572);
#19347=AXIS2_PLACEMENT_3D('',#36691,#23573,#23574);
#19348=AXIS2_PLACEMENT_3D('',#36701,#23575,#23576);
#19349=AXIS2_PLACEMENT_3D('',#36711,#23577,#23578);
#19350=AXIS2_PLACEMENT_3D('',#36721,#23579,#23580);
#19351=AXIS2_PLACEMENT_3D('',#36731,#23581,#23582);
#19352=AXIS2_PLACEMENT_3D('',#36741,#23583,#23584);
#19353=AXIS2_PLACEMENT_3D('',#36751,#23585,#23586);
#19354=AXIS2_PLACEMENT_3D('',#36761,#23587,#23588);
#19355=AXIS2_PLACEMENT_3D('',#36771,#23589,#23590);
#19356=AXIS2_PLACEMENT_3D('',#36781,#23591,#23592);
#19357=AXIS2_PLACEMENT_3D('',#36791,#23593,#23594);
#19358=AXIS2_PLACEMENT_3D('',#36801,#23595,#23596);
#19359=AXIS2_PLACEMENT_3D('',#36811,#23597,#23598);
#19360=AXIS2_PLACEMENT_3D('',#36821,#23599,#23600);
#19361=AXIS2_PLACEMENT_3D('',#36831,#23601,#23602);
#19362=AXIS2_PLACEMENT_3D('',#36841,#23603,#23604);
#19363=AXIS2_PLACEMENT_3D('',#36851,#23605,#23606);
#19364=AXIS2_PLACEMENT_3D('',#36861,#23607,#23608);
#19365=AXIS2_PLACEMENT_3D('',#36871,#23609,#23610);
#19366=AXIS2_PLACEMENT_3D('',#36881,#23611,#23612);
#19367=AXIS2_PLACEMENT_3D('',#36891,#23613,#23614);
#19368=AXIS2_PLACEMENT_3D('',#36901,#23615,#23616);
#19369=AXIS2_PLACEMENT_3D('',#36911,#23617,#23618);
#19370=AXIS2_PLACEMENT_3D('',#36921,#23619,#23620);
#19371=AXIS2_PLACEMENT_3D('',#36931,#23621,#23622);
#19372=AXIS2_PLACEMENT_3D('',#36941,#23623,#23624);
#19373=AXIS2_PLACEMENT_3D('',#36951,#23625,#23626);
#19374=AXIS2_PLACEMENT_3D('',#36958,#23628,#23629);
#19375=AXIS2_PLACEMENT_3D('',#36968,#23630,#23631);
#19376=AXIS2_PLACEMENT_3D('',#36978,#23632,#23633);
#19377=AXIS2_PLACEMENT_3D('',#36988,#23634,#23635);
#19378=AXIS2_PLACEMENT_3D('',#36998,#23636,#23637);
#19379=AXIS2_PLACEMENT_3D('',#37008,#23638,#23639);
#19380=AXIS2_PLACEMENT_3D('',#37018,#23640,#23641);
#19381=AXIS2_PLACEMENT_3D('',#37028,#23642,#23643);
#19382=AXIS2_PLACEMENT_3D('',#37038,#23644,#23645);
#19383=AXIS2_PLACEMENT_3D('',#37048,#23646,#23647);
#19384=AXIS2_PLACEMENT_3D('',#37058,#23648,#23649);
#19385=AXIS2_PLACEMENT_3D('',#37068,#23650,#23651);
#19386=AXIS2_PLACEMENT_3D('',#37078,#23652,#23653);
#19387=AXIS2_PLACEMENT_3D('',#37088,#23654,#23655);
#19388=AXIS2_PLACEMENT_3D('',#37098,#23656,#23657);
#19389=AXIS2_PLACEMENT_3D('',#37108,#23658,#23659);
#19390=AXIS2_PLACEMENT_3D('',#37118,#23660,#23661);
#19391=AXIS2_PLACEMENT_3D('',#37128,#23662,#23663);
#19392=AXIS2_PLACEMENT_3D('',#37138,#23664,#23665);
#19393=AXIS2_PLACEMENT_3D('',#37148,#23666,#23667);
#19394=AXIS2_PLACEMENT_3D('',#37158,#23668,#23669);
#19395=AXIS2_PLACEMENT_3D('',#37168,#23670,#23671);
#19396=AXIS2_PLACEMENT_3D('',#37178,#23672,#23673);
#19397=AXIS2_PLACEMENT_3D('',#37188,#23674,#23675);
#19398=AXIS2_PLACEMENT_3D('',#37198,#23676,#23677);
#19399=AXIS2_PLACEMENT_3D('',#37208,#23678,#23679);
#19400=AXIS2_PLACEMENT_3D('',#37218,#23680,#23681);
#19401=AXIS2_PLACEMENT_3D('',#37228,#23682,#23683);
#19402=AXIS2_PLACEMENT_3D('',#37238,#23684,#23685);
#19403=AXIS2_PLACEMENT_3D('',#37248,#23686,#23687);
#19404=AXIS2_PLACEMENT_3D('',#37258,#23688,#23689);
#19405=AXIS2_PLACEMENT_3D('',#37268,#23690,#23691);
#19406=AXIS2_PLACEMENT_3D('',#37278,#23692,#23693);
#19407=AXIS2_PLACEMENT_3D('',#37288,#23694,#23695);
#19408=AXIS2_PLACEMENT_3D('',#37298,#23696,#23697);
#19409=AXIS2_PLACEMENT_3D('',#37308,#23698,#23699);
#19410=AXIS2_PLACEMENT_3D('',#37318,#23700,#23701);
#19411=AXIS2_PLACEMENT_3D('',#37328,#23702,#23703);
#19412=AXIS2_PLACEMENT_3D('',#37338,#23704,#23705);
#19413=AXIS2_PLACEMENT_3D('',#37342,#23706,#23707);
#19414=AXIS2_PLACEMENT_3D('',#37349,#23708,#23709);
#19415=AXIS2_PLACEMENT_3D('',#37359,#23710,#23711);
#19416=AXIS2_PLACEMENT_3D('',#37369,#23712,#23713);
#19417=AXIS2_PLACEMENT_3D('',#37379,#23714,#23715);
#19418=AXIS2_PLACEMENT_3D('',#37389,#23716,#23717);
#19419=AXIS2_PLACEMENT_3D('',#37399,#23718,#23719);
#19420=AXIS2_PLACEMENT_3D('',#37409,#23720,#23721);
#19421=AXIS2_PLACEMENT_3D('',#37419,#23722,#23723);
#19422=AXIS2_PLACEMENT_3D('',#37429,#23724,#23725);
#19423=AXIS2_PLACEMENT_3D('',#37439,#23726,#23727);
#19424=AXIS2_PLACEMENT_3D('',#37449,#23728,#23729);
#19425=AXIS2_PLACEMENT_3D('',#37459,#23730,#23731);
#19426=AXIS2_PLACEMENT_3D('',#37469,#23732,#23733);
#19427=AXIS2_PLACEMENT_3D('',#37479,#23734,#23735);
#19428=AXIS2_PLACEMENT_3D('',#37489,#23736,#23737);
#19429=AXIS2_PLACEMENT_3D('',#37499,#23738,#23739);
#19430=AXIS2_PLACEMENT_3D('',#37509,#23740,#23741);
#19431=AXIS2_PLACEMENT_3D('',#37519,#23742,#23743);
#19432=AXIS2_PLACEMENT_3D('',#37529,#23744,#23745);
#19433=AXIS2_PLACEMENT_3D('',#37539,#23746,#23747);
#19434=AXIS2_PLACEMENT_3D('',#37549,#23748,#23749);
#19435=AXIS2_PLACEMENT_3D('',#37559,#23750,#23751);
#19436=AXIS2_PLACEMENT_3D('',#37569,#23752,#23753);
#19437=AXIS2_PLACEMENT_3D('',#37579,#23754,#23755);
#19438=AXIS2_PLACEMENT_3D('',#37589,#23756,#23757);
#19439=AXIS2_PLACEMENT_3D('',#37599,#23758,#23759);
#19440=AXIS2_PLACEMENT_3D('',#37609,#23760,#23761);
#19441=AXIS2_PLACEMENT_3D('',#37619,#23762,#23763);
#19442=AXIS2_PLACEMENT_3D('',#37629,#23764,#23765);
#19443=AXIS2_PLACEMENT_3D('',#37639,#23766,#23767);
#19444=AXIS2_PLACEMENT_3D('',#37649,#23768,#23769);
#19445=AXIS2_PLACEMENT_3D('',#37659,#23770,#23771);
#19446=AXIS2_PLACEMENT_3D('',#37669,#23772,#23773);
#19447=AXIS2_PLACEMENT_3D('',#37679,#23774,#23775);
#19448=AXIS2_PLACEMENT_3D('',#37689,#23776,#23777);
#19449=AXIS2_PLACEMENT_3D('',#37699,#23778,#23779);
#19450=AXIS2_PLACEMENT_3D('',#37709,#23780,#23781);
#19451=AXIS2_PLACEMENT_3D('',#37719,#23782,#23783);
#19452=AXIS2_PLACEMENT_3D('',#37729,#23784,#23785);
#19453=AXIS2_PLACEMENT_3D('',#37736,#23787,#23788);
#19454=AXIS2_PLACEMENT_3D('',#37746,#23789,#23790);
#19455=AXIS2_PLACEMENT_3D('',#37756,#23791,#23792);
#19456=AXIS2_PLACEMENT_3D('',#37766,#23793,#23794);
#19457=AXIS2_PLACEMENT_3D('',#37776,#23795,#23796);
#19458=AXIS2_PLACEMENT_3D('',#37786,#23797,#23798);
#19459=AXIS2_PLACEMENT_3D('',#37796,#23799,#23800);
#19460=AXIS2_PLACEMENT_3D('',#37806,#23801,#23802);
#19461=AXIS2_PLACEMENT_3D('',#37816,#23803,#23804);
#19462=AXIS2_PLACEMENT_3D('',#37826,#23805,#23806);
#19463=AXIS2_PLACEMENT_3D('',#37836,#23807,#23808);
#19464=AXIS2_PLACEMENT_3D('',#37846,#23809,#23810);
#19465=AXIS2_PLACEMENT_3D('',#37856,#23811,#23812);
#19466=AXIS2_PLACEMENT_3D('',#37866,#23813,#23814);
#19467=AXIS2_PLACEMENT_3D('',#37876,#23815,#23816);
#19468=AXIS2_PLACEMENT_3D('',#37886,#23817,#23818);
#19469=AXIS2_PLACEMENT_3D('',#37896,#23819,#23820);
#19470=AXIS2_PLACEMENT_3D('',#37906,#23821,#23822);
#19471=AXIS2_PLACEMENT_3D('',#37916,#23823,#23824);
#19472=AXIS2_PLACEMENT_3D('',#37926,#23825,#23826);
#19473=AXIS2_PLACEMENT_3D('',#37936,#23827,#23828);
#19474=AXIS2_PLACEMENT_3D('',#37946,#23829,#23830);
#19475=AXIS2_PLACEMENT_3D('',#37956,#23831,#23832);
#19476=AXIS2_PLACEMENT_3D('',#37966,#23833,#23834);
#19477=AXIS2_PLACEMENT_3D('',#37976,#23835,#23836);
#19478=AXIS2_PLACEMENT_3D('',#37986,#23837,#23838);
#19479=AXIS2_PLACEMENT_3D('',#37996,#23839,#23840);
#19480=AXIS2_PLACEMENT_3D('',#38006,#23841,#23842);
#19481=AXIS2_PLACEMENT_3D('',#38016,#23843,#23844);
#19482=AXIS2_PLACEMENT_3D('',#38026,#23845,#23846);
#19483=AXIS2_PLACEMENT_3D('',#38036,#23847,#23848);
#19484=AXIS2_PLACEMENT_3D('',#38046,#23849,#23850);
#19485=AXIS2_PLACEMENT_3D('',#38056,#23851,#23852);
#19486=AXIS2_PLACEMENT_3D('',#38066,#23853,#23854);
#19487=AXIS2_PLACEMENT_3D('',#38076,#23855,#23856);
#19488=AXIS2_PLACEMENT_3D('',#38086,#23857,#23858);
#19489=AXIS2_PLACEMENT_3D('',#38096,#23859,#23860);
#19490=AXIS2_PLACEMENT_3D('',#38106,#23861,#23862);
#19491=AXIS2_PLACEMENT_3D('',#38116,#23863,#23864);
#19492=AXIS2_PLACEMENT_3D('',#38120,#23865,#23866);
#19493=AXIS2_PLACEMENT_3D('',#38122,#23867,#23868);
#19494=AXIS2_PLACEMENT_3D('',#38124,#23870,#23871);
#19495=AXIS2_PLACEMENT_3D('',#38127,#23874,#23875);
#19496=AXIS2_PLACEMENT_3D('',#38130,#23878,#23879);
#19497=AXIS2_PLACEMENT_3D('',#38133,#23882,#23883);
#19498=AXIS2_PLACEMENT_3D('',#38136,#23886,#23887);
#19499=AXIS2_PLACEMENT_3D('',#38139,#23890,#23891);
#19500=AXIS2_PLACEMENT_3D('',#38142,#23894,#23895);
#19501=AXIS2_PLACEMENT_3D('',#38145,#23898,#23899);
#19502=AXIS2_PLACEMENT_3D('',#38148,#23902,#23903);
#19503=AXIS2_PLACEMENT_3D('',#38151,#23906,#23907);
#19504=AXIS2_PLACEMENT_3D('',#38154,#23910,#23911);
#19505=AXIS2_PLACEMENT_3D('',#38157,#23914,#23915);
#19506=AXIS2_PLACEMENT_3D('',#38160,#23918,#23919);
#19507=AXIS2_PLACEMENT_3D('',#38163,#23922,#23923);
#19508=AXIS2_PLACEMENT_3D('',#38166,#23926,#23927);
#19509=AXIS2_PLACEMENT_3D('',#38169,#23930,#23931);
#19510=AXIS2_PLACEMENT_3D('',#38172,#23934,#23935);
#19511=AXIS2_PLACEMENT_3D('',#38175,#23938,#23939);
#19512=AXIS2_PLACEMENT_3D('',#38178,#23942,#23943);
#19513=AXIS2_PLACEMENT_3D('',#38181,#23946,#23947);
#19514=AXIS2_PLACEMENT_3D('',#38184,#23950,#23951);
#19515=AXIS2_PLACEMENT_3D('',#38187,#23954,#23955);
#19516=AXIS2_PLACEMENT_3D('',#38190,#23958,#23959);
#19517=AXIS2_PLACEMENT_3D('',#38193,#23962,#23963);
#19518=AXIS2_PLACEMENT_3D('',#38196,#23966,#23967);
#19519=AXIS2_PLACEMENT_3D('',#38199,#23970,#23971);
#19520=AXIS2_PLACEMENT_3D('',#38202,#23974,#23975);
#19521=AXIS2_PLACEMENT_3D('',#38205,#23978,#23979);
#19522=AXIS2_PLACEMENT_3D('',#38208,#23982,#23983);
#19523=AXIS2_PLACEMENT_3D('',#38211,#23986,#23987);
#19524=AXIS2_PLACEMENT_3D('',#38214,#23990,#23991);
#19525=AXIS2_PLACEMENT_3D('',#38217,#23994,#23995);
#19526=AXIS2_PLACEMENT_3D('',#38220,#23998,#23999);
#19527=AXIS2_PLACEMENT_3D('',#38223,#24002,#24003);
#19528=AXIS2_PLACEMENT_3D('',#38226,#24006,#24007);
#19529=AXIS2_PLACEMENT_3D('',#38229,#24010,#24011);
#19530=AXIS2_PLACEMENT_3D('',#38232,#24014,#24015);
#19531=AXIS2_PLACEMENT_3D('',#38235,#24018,#24019);
#19532=AXIS2_PLACEMENT_3D('',#38238,#24022,#24023);
#19533=AXIS2_PLACEMENT_3D('',#38241,#24026,#24027);
#19534=AXIS2_PLACEMENT_3D('',#38244,#24030,#24031);
#19535=AXIS2_PLACEMENT_3D('',#38247,#24034,#24035);
#19536=AXIS2_PLACEMENT_3D('',#38250,#24038,#24039);
#19537=AXIS2_PLACEMENT_3D('',#38253,#24042,#24043);
#19538=AXIS2_PLACEMENT_3D('',#38256,#24046,#24047);
#19539=AXIS2_PLACEMENT_3D('',#38259,#24050,#24051);
#19540=AXIS2_PLACEMENT_3D('',#38262,#24054,#24055);
#19541=AXIS2_PLACEMENT_3D('',#38265,#24058,#24059);
#19542=AXIS2_PLACEMENT_3D('',#38268,#24062,#24063);
#19543=AXIS2_PLACEMENT_3D('',#38271,#24066,#24067);
#19544=AXIS2_PLACEMENT_3D('',#38274,#24070,#24071);
#19545=AXIS2_PLACEMENT_3D('',#38277,#24074,#24075);
#19546=AXIS2_PLACEMENT_3D('',#38280,#24078,#24079);
#19547=AXIS2_PLACEMENT_3D('',#38283,#24082,#24083);
#19548=AXIS2_PLACEMENT_3D('',#38286,#24086,#24087);
#19549=AXIS2_PLACEMENT_3D('',#38289,#24090,#24091);
#19550=AXIS2_PLACEMENT_3D('',#38292,#24094,#24095);
#19551=AXIS2_PLACEMENT_3D('',#38295,#24098,#24099);
#19552=AXIS2_PLACEMENT_3D('',#38298,#24102,#24103);
#19553=AXIS2_PLACEMENT_3D('',#38301,#24106,#24107);
#19554=AXIS2_PLACEMENT_3D('',#38304,#24110,#24111);
#19555=AXIS2_PLACEMENT_3D('',#38307,#24114,#24115);
#19556=AXIS2_PLACEMENT_3D('',#38310,#24118,#24119);
#19557=AXIS2_PLACEMENT_3D('',#38313,#24122,#24123);
#19558=AXIS2_PLACEMENT_3D('',#38316,#24126,#24127);
#19559=AXIS2_PLACEMENT_3D('',#38319,#24130,#24131);
#19560=AXIS2_PLACEMENT_3D('',#38322,#24134,#24135);
#19561=AXIS2_PLACEMENT_3D('',#38325,#24138,#24139);
#19562=AXIS2_PLACEMENT_3D('',#38328,#24142,#24143);
#19563=AXIS2_PLACEMENT_3D('',#38331,#24146,#24147);
#19564=AXIS2_PLACEMENT_3D('',#38334,#24150,#24151);
#19565=AXIS2_PLACEMENT_3D('',#38337,#24154,#24155);
#19566=AXIS2_PLACEMENT_3D('',#38340,#24158,#24159);
#19567=AXIS2_PLACEMENT_3D('',#38343,#24162,#24163);
#19568=AXIS2_PLACEMENT_3D('',#38346,#24166,#24167);
#19569=AXIS2_PLACEMENT_3D('',#38349,#24170,#24171);
#19570=AXIS2_PLACEMENT_3D('',#38352,#24174,#24175);
#19571=AXIS2_PLACEMENT_3D('',#38353,#24176,#24177);
#19572=AXIS2_PLACEMENT_3D('',#38356,#24180,#24181);
#19573=AXIS2_PLACEMENT_3D('',#38357,#24182,#24183);
#19574=AXIS2_PLACEMENT_3D('',#38358,#24184,#24185);
#19575=AXIS2_PLACEMENT_3D('',#38359,#24186,#24187);
#19576=AXIS2_PLACEMENT_3D('',#38361,#24189,#24190);
#19577=AXIS2_PLACEMENT_3D('',#38362,#24191,#24192);
#19578=AXIS2_PLACEMENT_3D('',#38364,#24194,#24195);
#19579=AXIS2_PLACEMENT_3D('',#38365,#24196,#24197);
#19580=AXIS2_PLACEMENT_3D('',#38367,#24199,#24200);
#19581=AXIS2_PLACEMENT_3D('',#38368,#24201,#24202);
#19582=AXIS2_PLACEMENT_3D('',#38370,#24204,#24205);
#19583=AXIS2_PLACEMENT_3D('',#38371,#24206,#24207);
#19584=AXIS2_PLACEMENT_3D('',#38373,#24209,#24210);
#19585=AXIS2_PLACEMENT_3D('',#38374,#24211,#24212);
#19586=AXIS2_PLACEMENT_3D('',#38376,#24214,#24215);
#19587=AXIS2_PLACEMENT_3D('',#38377,#24216,#24217);
#19588=AXIS2_PLACEMENT_3D('',#38379,#24219,#24220);
#19589=AXIS2_PLACEMENT_3D('',#38380,#24221,#24222);
#19590=AXIS2_PLACEMENT_3D('',#38382,#24224,#24225);
#19591=AXIS2_PLACEMENT_3D('',#38383,#24226,#24227);
#19592=AXIS2_PLACEMENT_3D('',#38385,#24229,#24230);
#19593=AXIS2_PLACEMENT_3D('',#38386,#24231,#24232);
#19594=AXIS2_PLACEMENT_3D('',#38388,#24234,#24235);
#19595=AXIS2_PLACEMENT_3D('',#38389,#24236,#24237);
#19596=AXIS2_PLACEMENT_3D('',#38391,#24239,#24240);
#19597=AXIS2_PLACEMENT_3D('',#38392,#24241,#24242);
#19598=AXIS2_PLACEMENT_3D('',#38394,#24244,#24245);
#19599=AXIS2_PLACEMENT_3D('',#38395,#24246,#24247);
#19600=AXIS2_PLACEMENT_3D('',#38397,#24249,#24250);
#19601=AXIS2_PLACEMENT_3D('',#38398,#24251,#24252);
#19602=AXIS2_PLACEMENT_3D('',#38400,#24254,#24255);
#19603=AXIS2_PLACEMENT_3D('',#38401,#24256,#24257);
#19604=AXIS2_PLACEMENT_3D('',#38403,#24259,#24260);
#19605=AXIS2_PLACEMENT_3D('',#38404,#24261,#24262);
#19606=AXIS2_PLACEMENT_3D('',#38406,#24264,#24265);
#19607=AXIS2_PLACEMENT_3D('',#38407,#24266,#24267);
#19608=AXIS2_PLACEMENT_3D('',#38409,#24269,#24270);
#19609=AXIS2_PLACEMENT_3D('',#38410,#24271,#24272);
#19610=AXIS2_PLACEMENT_3D('',#38412,#24274,#24275);
#19611=AXIS2_PLACEMENT_3D('',#38413,#24276,#24277);
#19612=AXIS2_PLACEMENT_3D('',#38415,#24279,#24280);
#19613=AXIS2_PLACEMENT_3D('',#38416,#24281,#24282);
#19614=AXIS2_PLACEMENT_3D('',#38418,#24284,#24285);
#19615=AXIS2_PLACEMENT_3D('',#38419,#24286,#24287);
#19616=AXIS2_PLACEMENT_3D('',#38421,#24289,#24290);
#19617=AXIS2_PLACEMENT_3D('',#38422,#24291,#24292);
#19618=AXIS2_PLACEMENT_3D('',#38424,#24294,#24295);
#19619=AXIS2_PLACEMENT_3D('',#38425,#24296,#24297);
#19620=AXIS2_PLACEMENT_3D('',#38427,#24299,#24300);
#19621=AXIS2_PLACEMENT_3D('',#38428,#24301,#24302);
#19622=AXIS2_PLACEMENT_3D('',#38430,#24304,#24305);
#19623=AXIS2_PLACEMENT_3D('',#38431,#24306,#24307);
#19624=AXIS2_PLACEMENT_3D('',#38433,#24309,#24310);
#19625=AXIS2_PLACEMENT_3D('',#38434,#24311,#24312);
#19626=AXIS2_PLACEMENT_3D('',#38436,#24314,#24315);
#19627=AXIS2_PLACEMENT_3D('',#38437,#24316,#24317);
#19628=AXIS2_PLACEMENT_3D('',#38439,#24319,#24320);
#19629=AXIS2_PLACEMENT_3D('',#38440,#24321,#24322);
#19630=AXIS2_PLACEMENT_3D('',#38442,#24324,#24325);
#19631=AXIS2_PLACEMENT_3D('',#38443,#24326,#24327);
#19632=AXIS2_PLACEMENT_3D('',#38445,#24329,#24330);
#19633=AXIS2_PLACEMENT_3D('',#38446,#24331,#24332);
#19634=AXIS2_PLACEMENT_3D('',#38448,#24334,#24335);
#19635=AXIS2_PLACEMENT_3D('',#38449,#24336,#24337);
#19636=AXIS2_PLACEMENT_3D('',#38451,#24339,#24340);
#19637=AXIS2_PLACEMENT_3D('',#38452,#24341,#24342);
#19638=AXIS2_PLACEMENT_3D('',#38454,#24344,#24345);
#19639=AXIS2_PLACEMENT_3D('',#38455,#24346,#24347);
#19640=AXIS2_PLACEMENT_3D('',#38457,#24349,#24350);
#19641=AXIS2_PLACEMENT_3D('',#38458,#24351,#24352);
#19642=AXIS2_PLACEMENT_3D('',#38460,#24354,#24355);
#19643=AXIS2_PLACEMENT_3D('',#38461,#24356,#24357);
#19644=AXIS2_PLACEMENT_3D('',#38463,#24359,#24360);
#19645=AXIS2_PLACEMENT_3D('',#38464,#24361,#24362);
#19646=AXIS2_PLACEMENT_3D('',#38466,#24364,#24365);
#19647=AXIS2_PLACEMENT_3D('',#38467,#24366,#24367);
#19648=AXIS2_PLACEMENT_3D('',#38469,#24369,#24370);
#19649=AXIS2_PLACEMENT_3D('',#38470,#24371,#24372);
#19650=AXIS2_PLACEMENT_3D('',#38472,#24374,#24375);
#19651=AXIS2_PLACEMENT_3D('',#38473,#24376,#24377);
#19652=AXIS2_PLACEMENT_3D('',#38475,#24379,#24380);
#19653=AXIS2_PLACEMENT_3D('',#38476,#24381,#24382);
#19654=AXIS2_PLACEMENT_3D('',#38478,#24384,#24385);
#19655=AXIS2_PLACEMENT_3D('',#38479,#24386,#24387);
#19656=AXIS2_PLACEMENT_3D('',#38481,#24389,#24390);
#19657=AXIS2_PLACEMENT_3D('',#38482,#24391,#24392);
#19658=AXIS2_PLACEMENT_3D('',#38484,#24394,#24395);
#19659=AXIS2_PLACEMENT_3D('',#38485,#24396,#24397);
#19660=AXIS2_PLACEMENT_3D('',#38487,#24399,#24400);
#19661=AXIS2_PLACEMENT_3D('',#38488,#24401,#24402);
#19662=AXIS2_PLACEMENT_3D('',#38490,#24404,#24405);
#19663=AXIS2_PLACEMENT_3D('',#38491,#24406,#24407);
#19664=AXIS2_PLACEMENT_3D('',#38493,#24409,#24410);
#19665=AXIS2_PLACEMENT_3D('',#38494,#24411,#24412);
#19666=AXIS2_PLACEMENT_3D('',#38496,#24414,#24415);
#19667=AXIS2_PLACEMENT_3D('',#38497,#24416,#24417);
#19668=AXIS2_PLACEMENT_3D('',#38499,#24419,#24420);
#19669=AXIS2_PLACEMENT_3D('',#38500,#24421,#24422);
#19670=AXIS2_PLACEMENT_3D('',#38502,#24424,#24425);
#19671=AXIS2_PLACEMENT_3D('',#38503,#24426,#24427);
#19672=AXIS2_PLACEMENT_3D('',#38505,#24429,#24430);
#19673=AXIS2_PLACEMENT_3D('',#38506,#24431,#24432);
#19674=AXIS2_PLACEMENT_3D('',#38508,#24434,#24435);
#19675=AXIS2_PLACEMENT_3D('',#38509,#24436,#24437);
#19676=AXIS2_PLACEMENT_3D('',#38511,#24439,#24440);
#19677=AXIS2_PLACEMENT_3D('',#38512,#24441,#24442);
#19678=AXIS2_PLACEMENT_3D('',#38514,#24444,#24445);
#19679=AXIS2_PLACEMENT_3D('',#38515,#24446,#24447);
#19680=AXIS2_PLACEMENT_3D('',#38517,#24449,#24450);
#19681=AXIS2_PLACEMENT_3D('',#38518,#24451,#24452);
#19682=AXIS2_PLACEMENT_3D('',#38520,#24454,#24455);
#19683=AXIS2_PLACEMENT_3D('',#38521,#24456,#24457);
#19684=AXIS2_PLACEMENT_3D('',#38523,#24459,#24460);
#19685=AXIS2_PLACEMENT_3D('',#38524,#24461,#24462);
#19686=AXIS2_PLACEMENT_3D('',#38526,#24464,#24465);
#19687=AXIS2_PLACEMENT_3D('',#38527,#24466,#24467);
#19688=AXIS2_PLACEMENT_3D('',#38529,#24469,#24470);
#19689=AXIS2_PLACEMENT_3D('',#38530,#24471,#24472);
#19690=AXIS2_PLACEMENT_3D('',#38532,#24474,#24475);
#19691=AXIS2_PLACEMENT_3D('',#38533,#24476,#24477);
#19692=AXIS2_PLACEMENT_3D('',#38535,#24479,#24480);
#19693=AXIS2_PLACEMENT_3D('',#38536,#24481,#24482);
#19694=AXIS2_PLACEMENT_3D('',#38538,#24484,#24485);
#19695=AXIS2_PLACEMENT_3D('',#38539,#24486,#24487);
#19696=AXIS2_PLACEMENT_3D('',#38541,#24489,#24490);
#19697=AXIS2_PLACEMENT_3D('',#38542,#24491,#24492);
#19698=AXIS2_PLACEMENT_3D('',#38544,#24494,#24495);
#19699=AXIS2_PLACEMENT_3D('',#38545,#24496,#24497);
#19700=AXIS2_PLACEMENT_3D('',#38547,#24499,#24500);
#19701=AXIS2_PLACEMENT_3D('',#38548,#24501,#24502);
#19702=AXIS2_PLACEMENT_3D('',#38550,#24504,#24505);
#19703=AXIS2_PLACEMENT_3D('',#38551,#24506,#24507);
#19704=AXIS2_PLACEMENT_3D('',#38553,#24509,#24510);
#19705=AXIS2_PLACEMENT_3D('',#38554,#24511,#24512);
#19706=AXIS2_PLACEMENT_3D('',#38556,#24514,#24515);
#19707=AXIS2_PLACEMENT_3D('',#38557,#24516,#24517);
#19708=AXIS2_PLACEMENT_3D('',#38559,#24519,#24520);
#19709=AXIS2_PLACEMENT_3D('',#38560,#24521,#24522);
#19710=AXIS2_PLACEMENT_3D('',#38562,#24524,#24525);
#19711=AXIS2_PLACEMENT_3D('',#38563,#24526,#24527);
#19712=AXIS2_PLACEMENT_3D('',#38565,#24529,#24530);
#19713=AXIS2_PLACEMENT_3D('',#38566,#24531,#24532);
#19714=AXIS2_PLACEMENT_3D('',#38568,#24534,#24535);
#19715=AXIS2_PLACEMENT_3D('',#38569,#24536,#24537);
#19716=AXIS2_PLACEMENT_3D('',#38571,#24539,#24540);
#19717=AXIS2_PLACEMENT_3D('',#38572,#24541,#24542);
#19718=AXIS2_PLACEMENT_3D('',#38574,#24544,#24545);
#19719=AXIS2_PLACEMENT_3D('',#38575,#24546,#24547);
#19720=AXIS2_PLACEMENT_3D('',#38577,#24549,#24550);
#19721=AXIS2_PLACEMENT_3D('',#38578,#24551,#24552);
#19722=AXIS2_PLACEMENT_3D('',#38580,#24554,#24555);
#19723=AXIS2_PLACEMENT_3D('',#38581,#24556,#24557);
#19724=AXIS2_PLACEMENT_3D('',#38583,#24559,#24560);
#19725=AXIS2_PLACEMENT_3D('',#38584,#24561,#24562);
#19726=AXIS2_PLACEMENT_3D('',#38586,#24564,#24565);
#19727=AXIS2_PLACEMENT_3D('',#38587,#24566,#24567);
#19728=AXIS2_PLACEMENT_3D('',#38589,#24569,#24570);
#21309=DIRECTION('axis',(0.,0.,1.));
#21310=DIRECTION('refdir',(1.,0.,0.));
#21311=DIRECTION('center_axis',(0.,1.,0.));
#21312=DIRECTION('ref_axis',(0.,0.,1.));
#21313=DIRECTION('center_axis',(0.,1.,0.));
#21314=DIRECTION('ref_axis',(0.,0.,-1.));
#21315=DIRECTION('',(-8.65956056235501E-17,0.707106781186541,-0.707106781186554));
#21316=DIRECTION('center_axis',(0.,-1.,0.));
#21317=DIRECTION('ref_axis',(0.,0.,-1.));
#21318=DIRECTION('center_axis',(0.,0.,1.));
#21319=DIRECTION('ref_axis',(1.,0.,0.));
#21320=DIRECTION('center_axis',(0.,0.,1.));
#21321=DIRECTION('ref_axis',(-1.,0.,0.));
#21322=DIRECTION('center_axis',(0.,0.,1.));
#21323=DIRECTION('ref_axis',(-1.,0.,0.));
#21324=DIRECTION('',(-0.707106781186545,-8.6595605623549E-17,0.70710678118655));
#21325=DIRECTION('center_axis',(-1.22464679914735E-16,0.,-1.));
#21326=DIRECTION('ref_axis',(-1.,0.,1.22464679914735E-16));
#21327=DIRECTION('center_axis',(0.,0.,1.));
#21328=DIRECTION('ref_axis',(1.,0.,0.));
#21329=DIRECTION('center_axis',(0.,0.,1.));
#21330=DIRECTION('ref_axis',(-1.,0.,0.));
#21331=DIRECTION('center_axis',(0.,0.,1.));
#21332=DIRECTION('ref_axis',(-1.,0.,0.));
#21333=DIRECTION('',(-0.707106781186547,-8.65956056235493E-17,0.707106781186548));
#21334=DIRECTION('center_axis',(-1.22464679914735E-16,0.,-1.));
#21335=DIRECTION('ref_axis',(-1.,0.,1.22464679914735E-16));
#21336=DIRECTION('center_axis',(0.,1.,0.));
#21337=DIRECTION('ref_axis',(0.,0.,1.));
#21338=DIRECTION('center_axis',(0.,1.,0.));
#21339=DIRECTION('ref_axis',(0.,0.,-1.));
#21340=DIRECTION('',(-8.65956056235498E-17,0.707106781186544,-0.707106781186551));
#21341=DIRECTION('center_axis',(0.,-1.,0.));
#21342=DIRECTION('ref_axis',(0.,0.,-1.));
#21343=DIRECTION('center_axis',(0.,0.,1.));
#21344=DIRECTION('ref_axis',(0.81777431008862,-0.575539032350614,0.));
#21345=DIRECTION('center_axis',(0.,0.,1.));
#21346=DIRECTION('ref_axis',(-1.,0.,0.));
#21347=DIRECTION('center_axis',(7.03266274044652E-17,0.,-1.));
#21348=DIRECTION('ref_axis',(-1.,0.,-7.03266274044651E-17));
#21349=DIRECTION('center_axis',(0.,-1.,0.));
#21350=DIRECTION('ref_axis',(0.,0.,-1.));
#21351=DIRECTION('center_axis',(0.,-1.,0.));
#21352=DIRECTION('ref_axis',(0.,0.,1.));
#21353=DIRECTION('center_axis',(0.,-1.,0.));
#21354=DIRECTION('ref_axis',(0.,0.,1.));
#21355=DIRECTION('',(-8.65956056235497E-17,-0.707106781186545,0.70710678118655));
#21356=DIRECTION('center_axis',(0.,1.,0.));
#21357=DIRECTION('ref_axis',(0.,0.,1.));
#21358=DIRECTION('center_axis',(0.,-1.,0.));
#21359=DIRECTION('ref_axis',(0.,0.,-1.));
#21360=DIRECTION('center_axis',(0.,-1.,0.));
#21361=DIRECTION('ref_axis',(0.,0.,-1.));
#21362=DIRECTION('center_axis',(0.,-1.,0.));
#21363=DIRECTION('ref_axis',(0.,0.,-1.));
#21364=DIRECTION('',(-8.6595605623549E-17,-0.707106781186551,0.707106781186544));
#21365=DIRECTION('center_axis',(0.,1.,0.));
#21366=DIRECTION('ref_axis',(0.,0.,-1.));
#21367=DIRECTION('center_axis',(0.,0.,-1.));
#21368=DIRECTION('ref_axis',(-1.,0.,0.));
#21369=DIRECTION('center_axis',(0.,0.,-1.));
#21370=DIRECTION('ref_axis',(1.,0.,0.));
#21371=DIRECTION('',(0.707106781186542,-8.65956056235487E-17,-0.707106781186553));
#21372=DIRECTION('center_axis',(0.,0.,1.));
#21373=DIRECTION('ref_axis',(1.,0.,0.));
#21374=DIRECTION('center_axis',(0.,0.,-1.));
#21375=DIRECTION('ref_axis',(-1.,0.,0.));
#21376=DIRECTION('center_axis',(0.,0.,-1.));
#21377=DIRECTION('ref_axis',(1.,0.,0.));
#21378=DIRECTION('',(0.707106781186544,-8.65956056235489E-17,-0.707106781186551));
#21379=DIRECTION('center_axis',(0.,0.,1.));
#21380=DIRECTION('ref_axis',(1.,0.,0.));
#21381=DIRECTION('center_axis',(0.,0.,-1.));
#21382=DIRECTION('ref_axis',(0.817774310088624,-0.575539032350609,0.));
#21383=DIRECTION('center_axis',(0.,0.,-1.));
#21384=DIRECTION('ref_axis',(1.,0.,0.));
#21385=DIRECTION('center_axis',(0.,0.,1.));
#21386=DIRECTION('ref_axis',(1.,0.,0.));
#21387=DIRECTION('center_axis',(0.,1.,0.));
#21388=DIRECTION('ref_axis',(0.,0.,1.));
#21389=DIRECTION('',(0.,1.,0.));
#21390=DIRECTION('center_axis',(0.,-1.,0.));
#21391=DIRECTION('ref_axis',(0.,0.,-1.));
#21392=DIRECTION('center_axis',(0.,-1.,0.));
#21393=DIRECTION('ref_axis',(0.,0.,-1.));
#21394=DIRECTION('center_axis',(0.,1.,0.));
#21395=DIRECTION('ref_axis',(0.,0.,1.));
#21396=DIRECTION('center_axis',(0.,1.,0.));
#21397=DIRECTION('ref_axis',(0.,0.,1.));
#21398=DIRECTION('',(0.,1.,0.));
#21399=DIRECTION('center_axis',(0.,1.,0.));
#21400=DIRECTION('ref_axis',(0.,0.,1.));
#21401=DIRECTION('',(0.,1.,0.));
#21402=DIRECTION('center_axis',(0.,0.,-1.));
#21403=DIRECTION('ref_axis',(0.782779647501618,-0.622298982368798,0.));
#21404=DIRECTION('',(0.,0.,-1.));
#21405=DIRECTION('',(0.,0.,-1.));
#21406=DIRECTION('',(0.,0.,-1.));
#21407=DIRECTION('center_axis',(0.,0.,-1.));
#21408=DIRECTION('ref_axis',(-1.,0.,0.));
#21409=DIRECTION('',(0.,0.,-1.));
#21410=DIRECTION('center_axis',(0.,0.,-1.));
#21411=DIRECTION('ref_axis',(-1.,0.,0.));
#21412=DIRECTION('',(0.,0.,-1.));
#21413=DIRECTION('center_axis',(1.,0.,0.));
#21414=DIRECTION('ref_axis',(0.,0.,-1.));
#21415=DIRECTION('',(0.,-1.,0.));
#21416=DIRECTION('',(0.,0.,-1.));
#21417=DIRECTION('',(0.,-1.,0.));
#21418=DIRECTION('',(0.,0.,-1.));
#21419=DIRECTION('center_axis',(-1.,0.,0.));
#21420=DIRECTION('ref_axis',(0.,0.,1.));
#21421=DIRECTION('',(0.,0.,1.));
#21422=DIRECTION('',(0.,-1.,0.));
#21423=DIRECTION('',(0.,0.,-1.));
#21424=DIRECTION('',(0.,1.,0.));
#21425=DIRECTION('center_axis',(0.,0.,1.));
#21426=DIRECTION('ref_axis',(1.,0.,0.));
#21427=DIRECTION('',(1.,0.,0.));
#21428=DIRECTION('center_axis',(0.,0.,1.));
#21429=DIRECTION('ref_axis',(1.,0.,0.));
#21430=DIRECTION('',(1.,-3.62769940560266E-16,0.));
#21431=DIRECTION('',(0.,-1.,0.));
#21432=DIRECTION('',(0.866013897511261,0.500019928920193,0.));
#21433=DIRECTION('',(1.,0.,0.));
#21434=DIRECTION('',(0.,-1.,0.));
#21435=DIRECTION('',(-1.,0.,0.));
#21436=DIRECTION('',(0.,-1.,0.));
#21437=DIRECTION('',(-0.866013897511262,0.500019928920192,0.));
#21438=DIRECTION('',(0.,-1.,0.));
#21439=DIRECTION('',(-1.,7.25539881120531E-16,0.));
#21440=DIRECTION('center_axis',(0.,0.,1.));
#21441=DIRECTION('ref_axis',(1.,0.,0.));
#21442=DIRECTION('',(-1.,0.,0.));
#21443=DIRECTION('center_axis',(1.,0.,0.));
#21444=DIRECTION('ref_axis',(0.,0.,-1.));
#21445=DIRECTION('',(0.,0.,1.));
#21446=DIRECTION('',(0.,-1.,0.));
#21447=DIRECTION('',(0.,0.,-1.));
#21448=DIRECTION('center_axis',(7.03266274044652E-17,0.,-1.));
#21449=DIRECTION('ref_axis',(-1.,0.,-7.03266274044652E-17));
#21450=DIRECTION('',(1.,0.,0.));
#21451=DIRECTION('',(-1.,0.,0.));
#21452=DIRECTION('center_axis',(7.03266274044652E-17,0.,-1.));
#21453=DIRECTION('ref_axis',(-1.,0.,-7.03266274044652E-17));
#21454=DIRECTION('',(-1.,7.25539881120531E-16,0.));
#21455=DIRECTION('',(0.,-1.,0.));
#21456=DIRECTION('',(-0.866013897511262,0.500019928920192,0.));
#21457=DIRECTION('',(1.,0.,7.03266274044652E-17));
#21458=DIRECTION('',(0.,1.,0.));
#21459=DIRECTION('',(1.,0.,7.03266274044652E-17));
#21460=DIRECTION('',(0.,1.,0.));
#21461=DIRECTION('',(-1.,0.,-7.03266274044652E-17));
#21462=DIRECTION('',(0.,1.,0.));
#21463=DIRECTION('',(-1.,0.,-7.03266274044652E-17));
#21464=DIRECTION('',(0.866013897511261,0.500019928920193,0.));
#21465=DIRECTION('',(0.,-1.,0.));
#21466=DIRECTION('',(1.,-3.62769940560266E-16,0.));
#21467=DIRECTION('center_axis',(7.03266274044652E-17,0.,-1.));
#21468=DIRECTION('ref_axis',(-1.,0.,-7.03266274044652E-17));
#21469=DIRECTION('center_axis',(-1.,0.,0.));
#21470=DIRECTION('ref_axis',(0.,0.,1.));
#21471=DIRECTION('',(0.,0.,1.));
#21472=DIRECTION('',(0.,-1.,0.));
#21473=DIRECTION('',(0.,0.,-1.));
#21474=DIRECTION('',(0.,-1.,0.));
#21475=DIRECTION('center_axis',(-1.22464679914735E-16,0.,-1.));
#21476=DIRECTION('ref_axis',(-1.,0.,1.22464679914735E-16));
#21477=DIRECTION('',(0.,-1.,0.));
#21478=DIRECTION('',(1.,0.,-1.22464679914735E-16));
#21479=DIRECTION('',(0.,1.,0.));
#21480=DIRECTION('',(-1.,0.,1.22464679914735E-16));
#21481=DIRECTION('',(0.,1.,0.));
#21482=DIRECTION('',(-1.,0.,0.));
#21483=DIRECTION('',(1.,0.,-1.22464679914735E-16));
#21484=DIRECTION('center_axis',(0.,-1.,0.));
#21485=DIRECTION('ref_axis',(0.,0.,-1.));
#21486=DIRECTION('',(-1.,0.,0.));
#21487=DIRECTION('',(0.,0.,1.));
#21488=DIRECTION('',(1.,0.,7.03266274044652E-17));
#21489=DIRECTION('',(0.,0.,-1.));
#21490=DIRECTION('center_axis',(0.,-1.,0.));
#21491=DIRECTION('ref_axis',(0.,0.,-1.));
#21492=DIRECTION('',(1.,0.,-1.22464679914735E-16));
#21493=DIRECTION('',(0.,0.,-1.));
#21494=DIRECTION('center_axis',(0.,-1.,0.));
#21495=DIRECTION('ref_axis',(0.,0.,-1.));
#21496=DIRECTION('',(0.,0.,1.));
#21497=DIRECTION('',(-1.,0.,1.22464679914735E-16));
#21498=DIRECTION('',(0.,0.,-1.));
#21499=DIRECTION('',(-1.,0.,0.));
#21500=DIRECTION('center_axis',(0.,1.,0.));
#21501=DIRECTION('ref_axis',(0.,0.,-1.));
#21502=DIRECTION('',(0.,0.,1.));
#21503=DIRECTION('',(-1.,0.,-7.03266274044652E-17));
#21504=DIRECTION('',(0.,0.,-1.));
#21505=DIRECTION('',(1.,0.,0.));
#21506=DIRECTION('center_axis',(0.,0.,-1.));
#21507=DIRECTION('ref_axis',(-1.,0.,0.));
#21508=DIRECTION('',(0.,0.,-1.));
#21509=DIRECTION('center_axis',(0.,0.,-1.));
#21510=DIRECTION('ref_axis',(1.,0.,0.));
#21511=DIRECTION('',(0.,0.,-1.));
#21512=DIRECTION('center_axis',(0.,0.,1.));
#21513=DIRECTION('ref_axis',(-1.,0.,0.));
#21514=DIRECTION('center_axis',(0.,-1.,0.));
#21515=DIRECTION('ref_axis',(0.,0.,-1.));
#21516=DIRECTION('center_axis',(0.,1.,0.));
#21517=DIRECTION('ref_axis',(0.,0.,1.));
#21518=DIRECTION('',(0.,0.,-1.));
#21519=DIRECTION('center_axis',(0.,0.,-1.));
#21520=DIRECTION('ref_axis',(-1.,0.,0.));
#21521=DIRECTION('',(0.,0.,-1.));
#21522=DIRECTION('center_axis',(0.,0.,-1.));
#21523=DIRECTION('ref_axis',(1.,0.,0.));
#21524=DIRECTION('center_axis',(0.,0.,1.));
#21525=DIRECTION('ref_axis',(-1.,0.,0.));
#21526=DIRECTION('center_axis',(3.62769940560266E-16,1.,0.));
#21527=DIRECTION('ref_axis',(-1.,3.62769940560266E-16,0.));
#21528=DIRECTION('',(0.,0.,-1.));
#21529=DIRECTION('center_axis',(1.,0.,0.));
#21530=DIRECTION('ref_axis',(0.,0.,-1.));
#21531=DIRECTION('',(0.,0.,-1.));
#21532=DIRECTION('center_axis',(-0.500019928920193,0.866013897511261,0.));
#21533=DIRECTION('ref_axis',(-0.866013897511261,-0.500019928920193,0.));
#21534=DIRECTION('center_axis',(-0.500019928920192,-0.866013897511262,0.));
#21535=DIRECTION('ref_axis',(0.866013897511262,-0.500019928920192,0.));
#21536=DIRECTION('',(0.,0.,-1.));
#21537=DIRECTION('center_axis',(1.,0.,0.));
#21538=DIRECTION('ref_axis',(0.,0.,-1.));
#21539=DIRECTION('',(0.,0.,-1.));
#21540=DIRECTION('center_axis',(-7.25539881120531E-16,-1.,0.));
#21541=DIRECTION('ref_axis',(1.,-7.25539881120531E-16,0.));
#21542=DIRECTION('center_axis',(0.,1.,0.));
#21543=DIRECTION('ref_axis',(0.,0.,1.));
#21544=DIRECTION('',(-1.,0.,-7.03266274044652E-17));
#21545=DIRECTION('',(0.,0.,-1.));
#21546=DIRECTION('center_axis',(0.,-1.,0.));
#21547=DIRECTION('ref_axis',(0.,0.,1.));
#21548=DIRECTION('',(1.,0.,0.));
#21549=DIRECTION('',(0.,0.,1.));
#21550=DIRECTION('center_axis',(1.,0.,0.));
#21551=DIRECTION('ref_axis',(0.,0.,-1.));
#21552=DIRECTION('',(0.,-1.,0.));
#21553=DIRECTION('',(0.,0.,1.));
#21554=DIRECTION('center_axis',(-1.,0.,0.));
#21555=DIRECTION('ref_axis',(0.,0.,1.));
#21556=DIRECTION('',(0.,-1.,0.));
#21557=DIRECTION('',(0.,0.,-1.));
#21558=DIRECTION('',(0.,-1.,0.));
#21559=DIRECTION('center_axis',(0.,0.,-1.));
#21560=DIRECTION('ref_axis',(-1.,0.,0.));
#21561=DIRECTION('',(0.,-1.,0.));
#21562=DIRECTION('',(1.,0.,0.));
#21563=DIRECTION('center_axis',(0.,-1.,0.));
#21564=DIRECTION('ref_axis',(0.,0.,-1.));
#21565=DIRECTION('center_axis',(0.,-1.,0.));
#21566=DIRECTION('ref_axis',(0.,0.,-1.));
#21567=DIRECTION('center_axis',(0.,-1.,0.));
#21568=DIRECTION('ref_axis',(0.,0.,-1.));
#21569=DIRECTION('',(0.,0.,1.));
#21570=DIRECTION('',(1.,0.,7.03266274044652E-17));
#21571=DIRECTION('center_axis',(0.,1.,0.));
#21572=DIRECTION('ref_axis',(0.,0.,-1.));
#21573=DIRECTION('center_axis',(-1.,0.,0.));
#21574=DIRECTION('ref_axis',(0.,0.,1.));
#21575=DIRECTION('',(0.,0.,1.));
#21576=DIRECTION('',(0.,-1.,0.));
#21577=DIRECTION('',(0.,1.,0.));
#21578=DIRECTION('center_axis',(0.,1.,0.));
#21579=DIRECTION('ref_axis',(0.,0.,1.));
#21580=DIRECTION('center_axis',(0.,1.,0.));
#21581=DIRECTION('ref_axis',(0.,0.,-1.));
#21582=DIRECTION('center_axis',(1.,0.,7.03266274044652E-17));
#21583=DIRECTION('ref_axis',(7.03266274044652E-17,0.,-1.));
#21584=DIRECTION('center_axis',(-1.,0.,-7.03266274044652E-17));
#21585=DIRECTION('ref_axis',(7.03266274044652E-17,0.,-1.));
#21586=DIRECTION('center_axis',(-0.707106781186551,-1.56441297777777E-14,
-0.707106781186544));
#21587=DIRECTION('ref_axis',(0.707106781186544,1.21590280983195E-12,-0.707106781186551));
#21588=DIRECTION('center_axis',(0.,0.,1.));
#21589=DIRECTION('ref_axis',(1.,0.,0.));
#21590=DIRECTION('center_axis',(0.707106781186562,-4.71888504772254E-14,
-0.707106781186534));
#21591=DIRECTION('ref_axis',(0.707106781186533,-2.06008383212131E-12,0.707106781186561));
#21592=DIRECTION('center_axis',(0.,0.,1.));
#21593=DIRECTION('ref_axis',(1.,0.,0.));
#21594=DIRECTION('center_axis',(0.,0.,-1.));
#21595=DIRECTION('ref_axis',(1.,0.,0.));
#21596=DIRECTION('center_axis',(0.,0.,-1.));
#21597=DIRECTION('ref_axis',(-1.,0.,0.));
#21598=DIRECTION('center_axis',(-1.,0.,0.));
#21599=DIRECTION('ref_axis',(0.,0.,1.));
#21600=DIRECTION('center_axis',(1.,0.,0.));
#21601=DIRECTION('ref_axis',(0.,0.,-1.));
#21602=DIRECTION('center_axis',(-1.,0.,-7.03266274044652E-17));
#21603=DIRECTION('ref_axis',(-7.03266274044652E-17,0.,1.));
#21604=DIRECTION('center_axis',(-1.,0.,-7.03266274044652E-17));
#21605=DIRECTION('ref_axis',(-7.03266274044652E-17,0.,1.));
#21606=DIRECTION('center_axis',(-0.707106781186528,4.00079384480861E-14,
-0.707106781186567));
#21607=DIRECTION('ref_axis',(0.707106781186567,-1.79317795020169E-12,-0.707106781186528));
#21608=DIRECTION('center_axis',(0.,-1.,0.));
#21609=DIRECTION('ref_axis',(0.,0.,-1.));
#21610=DIRECTION('center_axis',(1.,0.,5.78241158658936E-15));
#21611=DIRECTION('ref_axis',(5.78241158658936E-15,0.,-1.));
#21612=DIRECTION('center_axis',(1.,0.,0.));
#21613=DIRECTION('ref_axis',(0.,0.,1.));
#21614=DIRECTION('center_axis',(0.,-1.,0.));
#21615=DIRECTION('ref_axis',(0.,0.,1.));
#21616=DIRECTION('center_axis',(0.,0.,1.));
#21617=DIRECTION('ref_axis',(-1.,0.,0.));
#21618=DIRECTION('center_axis',(0.,0.,-1.));
#21619=DIRECTION('ref_axis',(-1.,0.,0.));
#21620=DIRECTION('center_axis',(0.707106781186562,4.71888504772271E-14,
-0.707106781186534));
#21621=DIRECTION('ref_axis',(0.707106781186534,1.37302321411511E-12,0.707106781186561));
#21622=DIRECTION('center_axis',(0.,0.,1.));
#21623=DIRECTION('ref_axis',(1.,0.,0.));
#21624=DIRECTION('center_axis',(0.,0.,-1.));
#21625=DIRECTION('ref_axis',(1.,0.,0.));
#21626=DIRECTION('center_axis',(0.,0.,-1.));
#21627=DIRECTION('ref_axis',(-1.,0.,0.));
#21628=DIRECTION('center_axis',(1.,0.,-1.22464679914735E-16));
#21629=DIRECTION('ref_axis',(-1.22464679914735E-16,0.,-1.));
#21630=DIRECTION('center_axis',(1.,0.,0.));
#21631=DIRECTION('ref_axis',(0.,0.,-1.));
#21632=DIRECTION('center_axis',(0.,0.,-1.));
#21633=DIRECTION('ref_axis',(-1.,0.,0.));
#21634=DIRECTION('center_axis',(0.,0.,1.));
#21635=DIRECTION('ref_axis',(1.,0.,0.));
#21636=DIRECTION('center_axis',(0.,-1.,0.));
#21637=DIRECTION('ref_axis',(0.,0.,-1.));
#21638=DIRECTION('center_axis',(0.,-1.,0.));
#21639=DIRECTION('ref_axis',(0.,0.,-1.));
#21640=DIRECTION('center_axis',(1.,0.,0.));
#21641=DIRECTION('ref_axis',(0.,0.,-1.));
#21642=DIRECTION('center_axis',(1.,0.,0.));
#21643=DIRECTION('ref_axis',(0.,0.,-1.));
#21644=DIRECTION('center_axis',(0.,-1.,0.));
#21645=DIRECTION('ref_axis',(0.,0.,-1.));
#21646=DIRECTION('center_axis',(1.,0.,5.78241158658936E-15));
#21647=DIRECTION('ref_axis',(5.78241158658936E-15,0.,-1.));
#21648=DIRECTION('center_axis',(1.,0.,0.));
#21649=DIRECTION('ref_axis',(0.,0.,1.));
#21650=DIRECTION('center_axis',(0.,-1.,0.));
#21651=DIRECTION('ref_axis',(0.,0.,1.));
#21652=DIRECTION('center_axis',(1.,0.,0.));
#21653=DIRECTION('ref_axis',(0.,1.,0.));
#21654=DIRECTION('center_axis',(0.,0.,1.));
#21655=DIRECTION('ref_axis',(-1.,0.,0.));
#21656=DIRECTION('center_axis',(-1.,0.,0.));
#21657=DIRECTION('ref_axis',(0.,0.,1.));
#21658=DIRECTION('center_axis',(0.707106781186508,-4.74453116211242E-14,
0.707106781186587));
#21659=DIRECTION('ref_axis',(0.707106781186587,-1.89154275080293E-13,-0.707106781186508));
#21660=DIRECTION('center_axis',(0.,-1.,0.));
#21661=DIRECTION('ref_axis',(0.,0.,-1.));
#21662=DIRECTION('center_axis',(0.,-1.,0.));
#21663=DIRECTION('ref_axis',(0.,0.,-1.));
#21664=DIRECTION('center_axis',(0.,0.,1.));
#21665=DIRECTION('ref_axis',(1.,0.,0.));
#21666=DIRECTION('center_axis',(-1.80700362080916E-16,0.,1.));
#21667=DIRECTION('ref_axis',(1.,0.,1.80700362080916E-16));
#21668=DIRECTION('center_axis',(0.,0.,-1.));
#21669=DIRECTION('ref_axis',(-1.,0.,0.));
#21670=DIRECTION('center_axis',(0.70710678118653,-1.47892592981158E-14,
0.707106781186565));
#21671=DIRECTION('ref_axis',(0.707106781186566,-1.36695930628953E-13,-0.70710678118653));
#21672=DIRECTION('center_axis',(0.,0.,1.));
#21673=DIRECTION('ref_axis',(0.,1.,0.));
#21674=DIRECTION('center_axis',(-1.,0.,0.));
#21675=DIRECTION('ref_axis',(0.,0.,-1.));
#21676=DIRECTION('center_axis',(-1.,0.,1.22464679914735E-16));
#21677=DIRECTION('ref_axis',(1.22464679914735E-16,0.,1.));
#21678=DIRECTION('center_axis',(0.,1.,0.));
#21679=DIRECTION('ref_axis',(1.,0.,0.));
#21680=DIRECTION('center_axis',(0.,-1.,0.));
#21681=DIRECTION('ref_axis',(0.,0.,-1.));
#21682=DIRECTION('center_axis',(0.,1.,0.));
#21683=DIRECTION('ref_axis',(0.,0.,1.));
#21684=DIRECTION('center_axis',(0.707106781186578,-0.707106781186517,4.00934254960531E-14));
#21685=DIRECTION('ref_axis',(0.707106781186517,0.707106781186578,-6.1787772477201E-12));
#21686=DIRECTION('center_axis',(-1.,0.,-7.03266274044652E-17));
#21687=DIRECTION('ref_axis',(-7.03266274044652E-17,0.,1.));
#21688=DIRECTION('center_axis',(0.707106781186556,-0.707106781186539,7.35188612507565E-15));
#21689=DIRECTION('ref_axis',(0.707106781186539,0.707106781186556,-4.57157300412597E-12));
#21690=DIRECTION('center_axis',(0.,-1.,0.));
#21691=DIRECTION('ref_axis',(0.,0.,-1.));
#21692=DIRECTION('center_axis',(-0.707106781186539,-0.707106781186557,7.43737317304176E-15));
#21693=DIRECTION('ref_axis',(0.707106781186556,-0.707106781186538,-2.45750013918949E-12));
#21694=DIRECTION('center_axis',(1.,0.,7.03266274044652E-17));
#21695=DIRECTION('ref_axis',(7.03266274044652E-17,0.,-1.));
#21696=DIRECTION('center_axis',(-0.70710678118656,-0.707106781186535,-2.52186791499698E-14));
#21697=DIRECTION('ref_axis',(0.707106781186535,-0.70710678118656,-4.09319520946051E-12));
#21698=DIRECTION('center_axis',(0.,1.,0.));
#21699=DIRECTION('ref_axis',(0.,0.,1.));
#21700=DIRECTION('center_axis',(0.,-1.,0.));
#21701=DIRECTION('ref_axis',(0.,0.,-1.));
#21702=DIRECTION('center_axis',(0.,1.,0.));
#21703=DIRECTION('ref_axis',(1.,0.,0.));
#21704=DIRECTION('center_axis',(0.,0.,-1.));
#21705=DIRECTION('ref_axis',(-1.,0.,0.));
#21706=DIRECTION('center_axis',(0.,0.,-1.));
#21707=DIRECTION('ref_axis',(-1.,0.,0.));
#21708=DIRECTION('center_axis',(0.,0.,1.));
#21709=DIRECTION('ref_axis',(1.,0.,0.));
#21710=DIRECTION('center_axis',(0.,0.,1.));
#21711=DIRECTION('ref_axis',(1.,0.,0.));
#21712=DIRECTION('center_axis',(1.39659253553725E-14,-1.,-3.49148133884313E-15));
#21713=DIRECTION('ref_axis',(1.,1.1842378929335E-14,0.));
#21714=DIRECTION('center_axis',(1.39659253553725E-14,-1.,-3.49148133884313E-15));
#21715=DIRECTION('ref_axis',(1.,1.39659253553725E-14,4.71264307122384E-30));
#21716=DIRECTION('center_axis',(-5.16843062991028E-29,3.49148133884313E-15,
-1.));
#21717=DIRECTION('ref_axis',(-1.,-1.48029736616687E-14,0.));
#21718=DIRECTION('center_axis',(-1.39659253553725E-14,1.,3.49148133884313E-15));
#21719=DIRECTION('ref_axis',(1.,1.39659253553726E-14,-1.73472347597681E-14));
#21720=DIRECTION('center_axis',(-1.39659253553725E-14,1.,3.49148133884313E-15));
#21721=DIRECTION('ref_axis',(1.,1.39659253553726E-14,-1.73472347597681E-14));
#21722=DIRECTION('center_axis',(1.39659253553725E-14,-1.,-3.49148133884313E-15));
#21723=DIRECTION('ref_axis',(1.,1.1842378929335E-14,0.));
#21724=DIRECTION('center_axis',(1.39659253553725E-14,-1.,-3.49148133884313E-15));
#21725=DIRECTION('ref_axis',(1.,1.39659253553725E-14,8.38340346178524E-30));
#21726=DIRECTION('center_axis',(1.39659253553725E-14,-1.,-3.49148133884313E-15));
#21727=DIRECTION('ref_axis',(1.,1.39659253553725E-14,8.38340346178524E-30));
#21728=DIRECTION('center_axis',(-5.16843062991028E-29,3.49148133884313E-15,
-1.));
#21729=DIRECTION('ref_axis',(-1.,-1.48029736616687E-14,0.));
#21730=DIRECTION('center_axis',(-1.39659253553725E-14,1.,3.49148133884313E-15));
#21731=DIRECTION('ref_axis',(1.,1.39659253553725E-14,4.71264307122384E-30));
#21732=DIRECTION('center_axis',(-1.39659253553725E-14,1.,3.49148133884313E-15));
#21733=DIRECTION('ref_axis',(-1.,-1.39659253553725E-14,-8.38340346178524E-30));
#21734=DIRECTION('',(1.39659253553725E-14,-1.,-3.49148133884313E-15));
#21735=DIRECTION('center_axis',(1.39659253553725E-14,-1.,-3.49148133884313E-15));
#21736=DIRECTION('ref_axis',(1.,1.39659253553725E-14,4.87617677579594E-29));
#21737=DIRECTION('center_axis',(1.39659253553725E-14,-1.,-3.49148133884313E-15));
#21738=DIRECTION('ref_axis',(1.,1.39659253553725E-14,4.87617677579594E-29));
#21739=DIRECTION('center_axis',(-0.999752444790186,-3.23231498703571E-17,
-0.0222496996844003));
#21740=DIRECTION('ref_axis',(-3.23151481062091E-17,1.,-7.19180377469308E-19));
#21741=DIRECTION('center_axis',(0.999752444790186,3.23231498703571E-17,
0.0222496996844003));
#21742=DIRECTION('ref_axis',(3.23151481062091E-17,-1.,7.19180377469308E-19));
#21743=DIRECTION('',(0.999752444790186,3.23231498703571E-17,0.0222496996844003));
#21744=DIRECTION('center_axis',(0.999752444790186,3.23231498703571E-17,
0.0222496996844003));
#21745=DIRECTION('ref_axis',(3.23151481062091E-17,-1.,7.19180377469308E-19));
#21746=DIRECTION('center_axis',(-0.999752444790186,-3.23231498703571E-17,
-0.0222496996844003));
#21747=DIRECTION('ref_axis',(-3.23151481062091E-17,1.,-7.19180377469308E-19));
#21748=DIRECTION('center_axis',(0.999752444790186,3.23231498703571E-17,
0.0222496996844003));
#21749=DIRECTION('ref_axis',(3.23151481062091E-17,-1.,7.19180377469308E-19));
#21750=DIRECTION('center_axis',(0.999752444790186,3.23231498703571E-17,
0.0222496996844003));
#21751=DIRECTION('ref_axis',(3.23151481062091E-17,-1.,7.19180377469308E-19));
#21752=DIRECTION('',(0.999752444790186,3.23231498703571E-17,0.0222496996844003));
#21753=DIRECTION('center_axis',(0.999752444790186,3.23231498703571E-17,
0.0222496996844003));
#21754=DIRECTION('ref_axis',(3.23151481062091E-17,-1.,7.19180377469308E-19));
#21755=DIRECTION('center_axis',(0.999752444790186,3.23231498703571E-17,
0.0222496996844003));
#21756=DIRECTION('ref_axis',(3.23151481062091E-17,-1.,7.19180377469308E-19));
#21757=DIRECTION('center_axis',(-0.0222496996844003,-1.18122020847398E-16,
0.999752444790186));
#21758=DIRECTION('ref_axis',(0.999752444790186,4.16004662851392E-32,0.0222496996844003));
#21759=DIRECTION('center_axis',(-0.0222496996844003,-1.18122020847398E-16,
0.999752444790186));
#21760=DIRECTION('ref_axis',(0.999752444790186,4.16004662851392E-32,0.0222496996844003));
#21761=DIRECTION('',(-0.0222496996844003,-1.18122020847398E-16,0.999752444790186));
#21762=DIRECTION('center_axis',(-0.0222496996844003,-1.18122020847398E-16,
0.999752444790186));
#21763=DIRECTION('ref_axis',(0.999752444790186,4.16004662851392E-32,0.0222496996844003));
#21764=DIRECTION('center_axis',(3.49433275961782E-17,-1.,-1.17373598748275E-16));
#21765=DIRECTION('ref_axis',(-0.999752444790186,-3.23231498703574E-17,-0.0222496996843981));
#21766=DIRECTION('center_axis',(3.49433275961782E-17,-1.,-1.17373598748275E-16));
#21767=DIRECTION('ref_axis',(-0.999752444790186,-3.23231498703574E-17,-0.0222496996843981));
#21768=DIRECTION('',(3.49433275961782E-17,-1.,-1.17373598748275E-16));
#21769=DIRECTION('center_axis',(-3.49433275961782E-17,1.,1.17373598748275E-16));
#21770=DIRECTION('ref_axis',(0.999752444790186,3.23231498703574E-17,0.0222496996843981));
#21771=DIRECTION('center_axis',(3.49433275961782E-17,-1.,-1.17373598748275E-16));
#21772=DIRECTION('ref_axis',(-0.999752444790186,-3.23231498703574E-17,-0.0222496996843981));
#21773=DIRECTION('center_axis',(-3.49433275961782E-17,1.,1.17373598748275E-16));
#21774=DIRECTION('ref_axis',(0.999752444790186,3.23231498703574E-17,0.0222496996843981));
#21775=DIRECTION('',(3.49433275961782E-17,-1.,-1.17373598748275E-16));
#21776=DIRECTION('center_axis',(-3.49433275961782E-17,1.,1.17373598748275E-16));
#21777=DIRECTION('ref_axis',(0.999752444790186,3.23231498703574E-17,0.0222496996843981));
#21778=DIRECTION('center_axis',(-0.0222496996844003,-1.18122020847398E-16,
0.999752444790186));
#21779=DIRECTION('ref_axis',(0.999752444790186,-1.2958542423238E-31,0.0222496996844003));
#21780=DIRECTION('center_axis',(-0.0222496996844003,-1.18122020847398E-16,
0.999752444790186));
#21781=DIRECTION('ref_axis',(0.999752444790186,-1.2958542423238E-31,0.0222496996844003));
#21782=DIRECTION('',(-0.0222496996844003,-1.18122020847398E-16,0.999752444790186));
#21783=DIRECTION('center_axis',(0.0222496996844003,1.18122020847398E-16,
-0.999752444790186));
#21784=DIRECTION('ref_axis',(0.999752444790186,-1.2958542423238E-31,0.0222496996844003));
#21785=DIRECTION('center_axis',(-0.999752444790186,-3.23231498703571E-17,
-0.0222496996844003));
#21786=DIRECTION('ref_axis',(-3.49433275961782E-17,1.,1.17373598748275E-16));
#21787=DIRECTION('',(3.49433275961782E-17,-1.,-1.17373598748275E-16));
#21788=DIRECTION('',(0.0222496996844003,1.18122020847398E-16,-0.999752444790186));
#21789=DIRECTION('',(3.49433275961782E-17,-1.,-1.17373598748275E-16));
#21790=DIRECTION('center_axis',(3.49433275961782E-17,-1.,-1.17373598748275E-16));
#21791=DIRECTION('ref_axis',(-0.999752444790186,-3.23231498703571E-17,-0.0222496996844003));
#21792=DIRECTION('',(3.49433275961782E-17,-1.,-1.17373598748275E-16));
#21793=DIRECTION('center_axis',(-3.49433275961782E-17,1.,1.17373598748275E-16));
#21794=DIRECTION('ref_axis',(0.999752444790186,3.23231498703571E-17,0.0222496996844003));
#21795=DIRECTION('',(3.49433275961782E-17,-1.,-1.17373598748275E-16));
#21796=DIRECTION('center_axis',(-3.49433275961782E-17,1.,1.17373598748275E-16));
#21797=DIRECTION('ref_axis',(-0.999752444790186,-3.23231498703571E-17,-0.0222496996844003));
#21798=DIRECTION('center_axis',(0.999752444790186,3.23231498703571E-17,
0.0222496996844003));
#21799=DIRECTION('ref_axis',(3.49433275961782E-17,-1.,-1.17373598748275E-16));
#21800=DIRECTION('',(-0.0222496996844003,-1.18122020847398E-16,0.999752444790186));
#21801=DIRECTION('',(3.49433275961782E-17,-1.,-1.17373598748275E-16));
#21802=DIRECTION('',(-0.0222496996844003,-1.18122020847398E-16,0.999752444790186));
#21803=DIRECTION('center_axis',(3.49433275961782E-17,-1.,-1.17373598748275E-16));
#21804=DIRECTION('ref_axis',(-0.999752444790186,-3.23231498703571E-17,-0.0222496996844003));
#21805=DIRECTION('',(-0.999752444790186,-3.23231498703571E-17,-0.0222496996844003));
#21806=DIRECTION('',(0.999752444790186,3.23231498703571E-17,0.0222496996844003));
#21807=DIRECTION('center_axis',(3.49433275961782E-17,-1.,-1.17373598748275E-16));
#21808=DIRECTION('ref_axis',(-0.999752444790186,-3.23231498703571E-17,-0.0222496996844003));
#21809=DIRECTION('',(0.0222496996844003,1.18122020847398E-16,-0.999752444790186));
#21810=DIRECTION('',(0.999752444790186,3.23231498703571E-17,0.0222496996844003));
#21811=DIRECTION('',(-0.0222496996844003,-1.18122020847398E-16,0.999752444790186));
#21812=DIRECTION('center_axis',(-3.49433275961782E-17,1.,1.17373598748275E-16));
#21813=DIRECTION('ref_axis',(-0.999752444790186,-3.23231498703571E-17,-0.0222496996844003));
#21814=DIRECTION('',(-0.999752444790186,-3.23231498703571E-17,-0.0222496996844003));
#21815=DIRECTION('center_axis',(-0.999752444790186,-3.23231498703571E-17,
-0.0222496996844003));
#21816=DIRECTION('ref_axis',(-3.49433275961782E-17,1.,1.17373598748275E-16));
#21817=DIRECTION('',(3.49433275961782E-17,-1.,-1.17373598748275E-16));
#21818=DIRECTION('',(3.49433275961782E-17,-1.,-1.17373598748275E-16));
#21819=DIRECTION('center_axis',(-0.0222496996844003,-1.18122020847398E-16,
0.999752444790186));
#21820=DIRECTION('ref_axis',(0.999752444790186,3.23231498703571E-17,0.0222496996844003));
#21821=DIRECTION('',(3.49433275961782E-17,-1.,-1.17373598748275E-16));
#21822=DIRECTION('',(0.999752444790186,3.23231498703571E-17,0.0222496996844003));
#21823=DIRECTION('',(3.49433275961782E-17,-1.,-1.17373598748275E-16));
#21824=DIRECTION('',(-0.999752444790186,-3.23231498703571E-17,-0.0222496996844003));
#21825=DIRECTION('center_axis',(3.49433275961782E-17,-1.,-1.17373598748275E-16));
#21826=DIRECTION('ref_axis',(-0.999752444790186,-3.23231498703571E-17,-0.0222496996844003));
#21827=DIRECTION('',(3.49433275961782E-17,-1.,-1.17373598748275E-16));
#21828=DIRECTION('center_axis',(3.49433275961782E-17,-1.,-1.17373598748275E-16));
#21829=DIRECTION('ref_axis',(-0.999752444790186,-3.23231498703571E-17,-0.0222496996844003));
#21830=DIRECTION('center_axis',(0.999752444790186,3.23231498703571E-17,
0.0222496996844003));
#21831=DIRECTION('ref_axis',(3.49433275961782E-17,-1.,-1.17373598748275E-16));
#21832=DIRECTION('',(3.49433275961782E-17,-1.,-1.17373598748275E-16));
#21833=DIRECTION('',(0.0222496996844003,1.18122020847398E-16,-0.999752444790186));
#21834=DIRECTION('center_axis',(0.0222496996844003,1.18122020847398E-16,
-0.999752444790186));
#21835=DIRECTION('ref_axis',(-0.999752444790186,-3.23231498703571E-17,-0.0222496996844003));
#21836=DIRECTION('',(0.999752444790186,3.23231498703571E-17,0.0222496996844003));
#21837=DIRECTION('',(3.49433275961782E-17,-1.,-1.17373598748275E-16));
#21838=DIRECTION('',(-0.999752444790186,-3.23231498703571E-17,-0.0222496996844003));
#21839=DIRECTION('center_axis',(-3.49433275961782E-17,1.,1.17373598748275E-16));
#21840=DIRECTION('ref_axis',(0.999752444790186,3.23231498703571E-17,0.0222496996844003));
#21841=DIRECTION('',(0.0222496996844003,1.18122020847398E-16,-0.999752444790186));
#21842=DIRECTION('center_axis',(3.49433275961782E-17,-1.,-1.17373598748275E-16));
#21843=DIRECTION('ref_axis',(-0.999752444790186,-3.23231498703571E-17,-0.0222496996844003));
#21844=DIRECTION('',(0.0222496996844003,1.18122020847398E-16,-0.999752444790186));
#21845=DIRECTION('center_axis',(0.999752444790186,3.23231498703571E-17,
0.0222496996844003));
#21846=DIRECTION('ref_axis',(0.0222496996844003,1.18122020847398E-16,-0.999752444790186));
#21847=DIRECTION('center_axis',(-0.0222496996844003,-1.18122020847398E-16,
0.999752444790186));
#21848=DIRECTION('ref_axis',(0.999752444790186,3.23231498703571E-17,0.0222496996844003));
#21849=DIRECTION('center_axis',(0.999752444790186,3.23231498703571E-17,
0.0222496996844003));
#21850=DIRECTION('ref_axis',(3.49433275961782E-17,-1.,-1.17373598748275E-16));
#21851=DIRECTION('center_axis',(0.999752444790186,3.23231498703571E-17,
0.0222496996844003));
#21852=DIRECTION('ref_axis',(3.49433275961782E-17,-1.,-1.17373598748275E-16));
#21853=DIRECTION('center_axis',(0.999752444790186,6.00249380122153E-17,
0.0222496996843998));
#21854=DIRECTION('ref_axis',(-0.0220459940098395,-0.135007583468649,0.990599276475646));
#21855=DIRECTION('center_axis',(0.999752444790186,6.00249380122153E-17,
0.0222496996843998));
#21856=DIRECTION('ref_axis',(-0.0220459940098395,-0.135007583468649,0.990599276475646));
#21857=DIRECTION('',(0.999752444790186,6.00249380122153E-17,0.0222496996843998));
#21858=DIRECTION('center_axis',(0.999752444790186,6.00249380122153E-17,
0.0222496996843998));
#21859=DIRECTION('ref_axis',(-0.0220459940098395,-0.135007583468649,0.990599276475646));
#21860=DIRECTION('center_axis',(-0.00300387818729384,0.99084456520988,0.134974161637996));
#21861=DIRECTION('ref_axis',(0.0220459940098398,0.135007583468648,-0.990599276475646));
#21862=DIRECTION('center_axis',(0.999752444790186,1.11968515267594E-16,
0.0222496996843994));
#21863=DIRECTION('ref_axis',(-0.0220459940098391,-0.135007583468648,0.990599276475646));
#21864=DIRECTION('center_axis',(-0.999752444790186,-5.98479599211999E-17,
-0.0222496996843998));
#21865=DIRECTION('ref_axis',(0.0220459940098395,0.135007583468649,-0.990599276475646));
#21866=DIRECTION('center_axis',(-2.44929359829471E-16,0.,-1.));
#21867=DIRECTION('ref_axis',(-1.,0.,0.));
#21868=DIRECTION('center_axis',(-2.44929359829471E-16,0.,-1.));
#21869=DIRECTION('ref_axis',(-1.,0.,2.44929359829471E-16));
#21870=DIRECTION('center_axis',(0.,1.,0.));
#21871=DIRECTION('ref_axis',(1.,0.,0.));
#21872=DIRECTION('center_axis',(2.44929359829471E-16,0.,1.));
#21873=DIRECTION('ref_axis',(-1.,0.,2.44929359829471E-16));
#21874=DIRECTION('center_axis',(-2.44929359829471E-16,0.,-1.));
#21875=DIRECTION('ref_axis',(-1.,0.,2.44929359829471E-16));
#21876=DIRECTION('center_axis',(-2.44929359829471E-16,-1.22460635382238E-16,
-1.));
#21877=DIRECTION('ref_axis',(-2.99942050284817E-32,1.,-1.22460635382238E-16));
#21878=DIRECTION('center_axis',(-2.44929359829471E-16,-1.22460635382238E-16,
-1.));
#21879=DIRECTION('ref_axis',(-2.99942050284817E-32,1.,-1.22460635382238E-16));
#21880=DIRECTION('',(-0.707106781186546,8.65956056235492E-17,0.707106781186549));
#21881=DIRECTION('center_axis',(-2.44929359829471E-16,0.,-1.));
#21882=DIRECTION('ref_axis',(-1.,0.,2.44929359829471E-16));
#21883=DIRECTION('center_axis',(-2.44929359829471E-16,-1.22460635382238E-16,
-1.));
#21884=DIRECTION('ref_axis',(2.99942050284817E-32,-1.,1.22460635382238E-16));
#21885=DIRECTION('center_axis',(-2.44929359829471E-16,-1.22460635382238E-16,
-1.));
#21886=DIRECTION('ref_axis',(2.99942050284817E-32,-1.,1.22460635382238E-16));
#21887=DIRECTION('center_axis',(-2.44929359829471E-16,-1.22460635382238E-16,
-1.));
#21888=DIRECTION('ref_axis',(2.99942050284817E-32,-1.,1.22460635382238E-16));
#21889=DIRECTION('',(4.01685164633802E-17,-0.819152044288988,0.573576436351052));
#21890=DIRECTION('center_axis',(-2.44929359829471E-16,-1.22460635382238E-16,
-1.));
#21891=DIRECTION('ref_axis',(2.99942050284817E-32,-1.,1.22460635382238E-16));
#21892=DIRECTION('center_axis',(-2.44929359829471E-16,-1.22460635382238E-16,
-1.));
#21893=DIRECTION('ref_axis',(2.99942050284817E-32,-1.,1.22460635382238E-16));
#21894=DIRECTION('center_axis',(2.44929359829471E-16,1.22460635382238E-16,
1.));
#21895=DIRECTION('ref_axis',(-2.99942050284817E-32,1.,-1.22460635382238E-16));
#21896=DIRECTION('',(-2.40802902274083E-16,0.819152044288993,-0.573576436351044));
#21897=DIRECTION('center_axis',(-2.44929359829471E-16,0.,-1.));
#21898=DIRECTION('ref_axis',(-1.,0.,2.44929359829471E-16));
#21899=DIRECTION('center_axis',(-2.44929359829471E-16,-1.22460635382238E-16,
-1.));
#21900=DIRECTION('ref_axis',(2.99942050284817E-32,-1.,1.22460635382238E-16));
#21901=DIRECTION('center_axis',(-2.44929359829471E-16,-1.22460635382238E-16,
-1.));
#21902=DIRECTION('ref_axis',(2.99942050284817E-32,-1.,1.22460635382238E-16));
#21903=DIRECTION('',(2.44929359829471E-16,0.,1.));
#21904=DIRECTION('center_axis',(-2.44929359829471E-16,-1.22460635382238E-16,
-1.));
#21905=DIRECTION('ref_axis',(2.99942050284817E-32,-1.,1.22460635382238E-16));
#21906=DIRECTION('center_axis',(-2.44929359829471E-16,-1.22460635382238E-16,
-1.));
#21907=DIRECTION('ref_axis',(2.99942050284817E-32,-1.,1.22460635382238E-16));
#21908=DIRECTION('center_axis',(-2.44929359829471E-16,-1.22460635382238E-16,
-1.));
#21909=DIRECTION('ref_axis',(2.99942050284817E-32,-1.,1.22460635382238E-16));
#21910=DIRECTION('',(4.01685164633802E-17,-0.819152044288988,0.573576436351052));
#21911=DIRECTION('center_axis',(-2.44929359829471E-16,-1.22460635382238E-16,
-1.));
#21912=DIRECTION('ref_axis',(2.99942050284817E-32,-1.,1.22460635382238E-16));
#21913=DIRECTION('center_axis',(-2.44929359829471E-16,-1.22460635382238E-16,
-1.));
#21914=DIRECTION('ref_axis',(2.99942050284817E-32,-1.,1.22460635382238E-16));
#21915=DIRECTION('center_axis',(2.44929359829471E-16,1.22460635382238E-16,
1.));
#21916=DIRECTION('ref_axis',(-2.99942050284817E-32,1.,-1.22460635382238E-16));
#21917=DIRECTION('',(-2.40802902274083E-16,0.819152044288993,-0.573576436351044));
#21918=DIRECTION('center_axis',(-2.44929359829471E-16,0.,-1.));
#21919=DIRECTION('ref_axis',(-1.,0.,2.44929359829471E-16));
#21920=DIRECTION('center_axis',(-2.44929359829471E-16,-1.22460635382238E-16,
-1.));
#21921=DIRECTION('ref_axis',(2.99942050284817E-32,-1.,1.22460635382238E-16));
#21922=DIRECTION('center_axis',(-2.44929359829471E-16,-1.22460635382238E-16,
-1.));
#21923=DIRECTION('ref_axis',(2.99942050284817E-32,-1.,1.22460635382238E-16));
#21924=DIRECTION('',(2.44929359829471E-16,0.,1.));
#21925=DIRECTION('center_axis',(-2.44929359829471E-16,-1.22460635382238E-16,
-1.));
#21926=DIRECTION('ref_axis',(2.99942050284817E-32,-1.,1.22460635382238E-16));
#21927=DIRECTION('center_axis',(-2.44929359829471E-16,-1.22460635382238E-16,
-1.));
#21928=DIRECTION('ref_axis',(2.99942050284817E-32,-1.,1.22460635382238E-16));
#21929=DIRECTION('center_axis',(-2.44929359829471E-16,-1.22460635382238E-16,
-1.));
#21930=DIRECTION('ref_axis',(2.99942050284817E-32,-1.,1.22460635382238E-16));
#21931=DIRECTION('',(4.01685164633802E-17,-0.819152044288988,0.573576436351052));
#21932=DIRECTION('center_axis',(-2.44929359829471E-16,-1.22460635382238E-16,
-1.));
#21933=DIRECTION('ref_axis',(2.99942050284817E-32,-1.,1.22460635382238E-16));
#21934=DIRECTION('center_axis',(-2.44929359829471E-16,-1.22460635382238E-16,
-1.));
#21935=DIRECTION('ref_axis',(2.99942050284817E-32,-1.,1.22460635382238E-16));
#21936=DIRECTION('center_axis',(2.44929359829471E-16,1.22460635382238E-16,
1.));
#21937=DIRECTION('ref_axis',(-2.99942050284817E-32,1.,-1.22460635382238E-16));
#21938=DIRECTION('',(-2.40802902274083E-16,0.819152044288993,-0.573576436351044));
#21939=DIRECTION('center_axis',(-2.44929359829471E-16,0.,-1.));
#21940=DIRECTION('ref_axis',(-1.,0.,2.44929359829471E-16));
#21941=DIRECTION('center_axis',(-2.44929359829471E-16,-1.22460635382238E-16,
-1.));
#21942=DIRECTION('ref_axis',(2.99942050284817E-32,-1.,1.22460635382238E-16));
#21943=DIRECTION('center_axis',(-2.44929359829471E-16,-1.22460635382238E-16,
-1.));
#21944=DIRECTION('ref_axis',(2.99942050284817E-32,-1.,1.22460635382238E-16));
#21945=DIRECTION('',(2.44929359829471E-16,0.,1.));
#21946=DIRECTION('center_axis',(-2.44929359829471E-16,-1.22460635382238E-16,
-1.));
#21947=DIRECTION('ref_axis',(2.99942050284817E-32,-1.,1.22460635382238E-16));
#21948=DIRECTION('center_axis',(-2.44929359829471E-16,-1.22460635382238E-16,
-1.));
#21949=DIRECTION('ref_axis',(2.99942050284817E-32,-1.,1.22460635382238E-16));
#21950=DIRECTION('center_axis',(-2.44929359829471E-16,-1.22460635382238E-16,
-1.));
#21951=DIRECTION('ref_axis',(2.99942050284817E-32,-1.,1.22460635382238E-16));
#21952=DIRECTION('',(4.01685164633802E-17,-0.819152044288988,0.573576436351052));
#21953=DIRECTION('center_axis',(-2.44929359829471E-16,-1.22460635382238E-16,
-1.));
#21954=DIRECTION('ref_axis',(2.99942050284817E-32,-1.,1.22460635382238E-16));
#21955=DIRECTION('center_axis',(-2.44929359829471E-16,-1.22460635382238E-16,
-1.));
#21956=DIRECTION('ref_axis',(2.99942050284817E-32,-1.,1.22460635382238E-16));
#21957=DIRECTION('center_axis',(2.44929359829471E-16,1.22460635382238E-16,
1.));
#21958=DIRECTION('ref_axis',(-2.99942050284817E-32,1.,-1.22460635382238E-16));
#21959=DIRECTION('',(-2.40802902274083E-16,0.819152044288993,-0.573576436351044));
#21960=DIRECTION('center_axis',(-2.44929359829471E-16,0.,-1.));
#21961=DIRECTION('ref_axis',(-1.,0.,2.44929359829471E-16));
#21962=DIRECTION('center_axis',(-2.44929359829471E-16,-1.22460635382238E-16,
-1.));
#21963=DIRECTION('ref_axis',(2.99942050284817E-32,-1.,1.22460635382238E-16));
#21964=DIRECTION('center_axis',(-2.44929359829471E-16,-1.22460635382238E-16,
-1.));
#21965=DIRECTION('ref_axis',(2.99942050284817E-32,-1.,1.22460635382238E-16));
#21966=DIRECTION('',(2.44929359829471E-16,0.,1.));
#21967=DIRECTION('center_axis',(-2.44929359829471E-16,-1.22460635382238E-16,
-1.));
#21968=DIRECTION('ref_axis',(2.99942050284817E-32,-1.,1.22460635382238E-16));
#21969=DIRECTION('center_axis',(-2.44929359829471E-16,-1.22460635382238E-16,
-1.));
#21970=DIRECTION('ref_axis',(2.99942050284817E-32,-1.,1.22460635382238E-16));
#21971=DIRECTION('center_axis',(-2.44929359829471E-16,-1.22460635382238E-16,
-1.));
#21972=DIRECTION('ref_axis',(2.99942050284817E-32,-1.,1.22460635382238E-16));
#21973=DIRECTION('',(4.01685164633802E-17,-0.819152044288988,0.573576436351052));
#21974=DIRECTION('center_axis',(-2.44929359829471E-16,-1.22460635382238E-16,
-1.));
#21975=DIRECTION('ref_axis',(2.99942050284817E-32,-1.,1.22460635382238E-16));
#21976=DIRECTION('center_axis',(-2.44929359829471E-16,-1.22460635382238E-16,
-1.));
#21977=DIRECTION('ref_axis',(2.99942050284817E-32,-1.,1.22460635382238E-16));
#21978=DIRECTION('center_axis',(2.44929359829471E-16,1.22460635382238E-16,
1.));
#21979=DIRECTION('ref_axis',(-2.99942050284817E-32,1.,-1.22460635382238E-16));
#21980=DIRECTION('',(-2.40802902274083E-16,0.819152044288993,-0.573576436351044));
#21981=DIRECTION('center_axis',(-2.44929359829471E-16,0.,-1.));
#21982=DIRECTION('ref_axis',(-1.,0.,2.44929359829471E-16));
#21983=DIRECTION('center_axis',(-2.44929359829471E-16,-1.22460635382238E-16,
-1.));
#21984=DIRECTION('ref_axis',(2.99942050284817E-32,-1.,1.22460635382238E-16));
#21985=DIRECTION('center_axis',(-2.44929359829471E-16,-1.22460635382238E-16,
-1.));
#21986=DIRECTION('ref_axis',(2.99942050284817E-32,-1.,1.22460635382238E-16));
#21987=DIRECTION('',(2.44929359829471E-16,0.,1.));
#21988=DIRECTION('center_axis',(-2.44929359829471E-16,-1.22460635382238E-16,
-1.));
#21989=DIRECTION('ref_axis',(2.99942050284817E-32,-1.,1.22460635382238E-16));
#21990=DIRECTION('center_axis',(-2.44929359829471E-16,-1.22460635382238E-16,
-1.));
#21991=DIRECTION('ref_axis',(2.99942050284817E-32,-1.,1.22460635382238E-16));
#21992=DIRECTION('center_axis',(-2.44929359829471E-16,-1.22460635382238E-16,
-1.));
#21993=DIRECTION('ref_axis',(2.99942050284817E-32,-1.,1.22460635382238E-16));
#21994=DIRECTION('',(4.01685164633802E-17,-0.819152044288988,0.573576436351052));
#21995=DIRECTION('center_axis',(-2.44929359829471E-16,-1.22460635382238E-16,
-1.));
#21996=DIRECTION('ref_axis',(2.99942050284817E-32,-1.,1.22460635382238E-16));
#21997=DIRECTION('center_axis',(-2.44929359829471E-16,-1.22460635382238E-16,
-1.));
#21998=DIRECTION('ref_axis',(2.99942050284817E-32,-1.,1.22460635382238E-16));
#21999=DIRECTION('center_axis',(2.44929359829471E-16,1.22460635382238E-16,
1.));
#22000=DIRECTION('ref_axis',(-2.99942050284817E-32,1.,-1.22460635382238E-16));
#22001=DIRECTION('',(-2.40802902274083E-16,0.819152044288993,-0.573576436351044));
#22002=DIRECTION('center_axis',(-2.44929359829471E-16,0.,-1.));
#22003=DIRECTION('ref_axis',(-1.,0.,2.44929359829471E-16));
#22004=DIRECTION('center_axis',(-2.44929359829471E-16,-1.22460635382238E-16,
-1.));
#22005=DIRECTION('ref_axis',(2.99942050284817E-32,-1.,1.22460635382238E-16));
#22006=DIRECTION('center_axis',(-2.44929359829471E-16,-1.22460635382238E-16,
-1.));
#22007=DIRECTION('ref_axis',(2.99942050284817E-32,-1.,1.22460635382238E-16));
#22008=DIRECTION('',(2.44929359829471E-16,0.,1.));
#22009=DIRECTION('center_axis',(-2.44929359829471E-16,-1.22460635382238E-16,
-1.));
#22010=DIRECTION('ref_axis',(2.99942050284817E-32,-1.,1.22460635382238E-16));
#22011=DIRECTION('center_axis',(-2.44929359829471E-16,-1.22460635382238E-16,
-1.));
#22012=DIRECTION('ref_axis',(2.99942050284817E-32,-1.,1.22460635382238E-16));
#22013=DIRECTION('center_axis',(-2.44929359829471E-16,-1.22460635382238E-16,
-1.));
#22014=DIRECTION('ref_axis',(2.99942050284817E-32,-1.,1.22460635382238E-16));
#22015=DIRECTION('',(4.01685164633802E-17,-0.819152044288988,0.573576436351052));
#22016=DIRECTION('center_axis',(-2.44929359829471E-16,-1.22460635382238E-16,
-1.));
#22017=DIRECTION('ref_axis',(2.99942050284817E-32,-1.,1.22460635382238E-16));
#22018=DIRECTION('center_axis',(-2.44929359829471E-16,-1.22460635382238E-16,
-1.));
#22019=DIRECTION('ref_axis',(2.99942050284817E-32,-1.,1.22460635382238E-16));
#22020=DIRECTION('center_axis',(2.44929359829471E-16,1.22460635382238E-16,
1.));
#22021=DIRECTION('ref_axis',(-2.99942050284817E-32,1.,-1.22460635382238E-16));
#22022=DIRECTION('',(-2.40802902274083E-16,0.819152044288993,-0.573576436351044));
#22023=DIRECTION('center_axis',(-2.44929359829471E-16,0.,-1.));
#22024=DIRECTION('ref_axis',(-1.,0.,2.44929359829471E-16));
#22025=DIRECTION('center_axis',(-2.44929359829471E-16,-1.22460635382238E-16,
-1.));
#22026=DIRECTION('ref_axis',(2.99942050284817E-32,-1.,1.22460635382238E-16));
#22027=DIRECTION('center_axis',(-2.44929359829471E-16,-1.22460635382238E-16,
-1.));
#22028=DIRECTION('ref_axis',(2.99942050284817E-32,-1.,1.22460635382238E-16));
#22029=DIRECTION('',(2.44929359829471E-16,0.,1.));
#22030=DIRECTION('center_axis',(-2.44929359829471E-16,-1.22460635382238E-16,
-1.));
#22031=DIRECTION('ref_axis',(2.99942050284817E-32,-1.,1.22460635382238E-16));
#22032=DIRECTION('center_axis',(-2.44929359829471E-16,-1.22460635382238E-16,
-1.));
#22033=DIRECTION('ref_axis',(2.99942050284817E-32,-1.,1.22460635382238E-16));
#22034=DIRECTION('center_axis',(-2.44929359829471E-16,-1.22460635382238E-16,
-1.));
#22035=DIRECTION('ref_axis',(2.99942050284817E-32,-1.,1.22460635382238E-16));
#22036=DIRECTION('',(4.01685164633802E-17,-0.819152044288988,0.573576436351052));
#22037=DIRECTION('center_axis',(-2.44929359829471E-16,-1.22460635382238E-16,
-1.));
#22038=DIRECTION('ref_axis',(2.99942050284817E-32,-1.,1.22460635382238E-16));
#22039=DIRECTION('center_axis',(-2.44929359829471E-16,-1.22460635382238E-16,
-1.));
#22040=DIRECTION('ref_axis',(2.99942050284817E-32,-1.,1.22460635382238E-16));
#22041=DIRECTION('center_axis',(2.44929359829471E-16,1.22460635382238E-16,
1.));
#22042=DIRECTION('ref_axis',(-2.99942050284817E-32,1.,-1.22460635382238E-16));
#22043=DIRECTION('',(-2.40802902274083E-16,0.819152044288993,-0.573576436351044));
#22044=DIRECTION('center_axis',(-2.44929359829471E-16,0.,-1.));
#22045=DIRECTION('ref_axis',(-1.,0.,2.44929359829471E-16));
#22046=DIRECTION('center_axis',(-2.44929359829471E-16,-1.22460635382238E-16,
-1.));
#22047=DIRECTION('ref_axis',(2.99942050284817E-32,-1.,1.22460635382238E-16));
#22048=DIRECTION('center_axis',(-2.44929359829471E-16,-1.22460635382238E-16,
-1.));
#22049=DIRECTION('ref_axis',(2.99942050284817E-32,-1.,1.22460635382238E-16));
#22050=DIRECTION('',(2.44929359829471E-16,0.,1.));
#22051=DIRECTION('center_axis',(-2.44929359829471E-16,-1.22460635382238E-16,
-1.));
#22052=DIRECTION('ref_axis',(2.99942050284817E-32,-1.,1.22460635382238E-16));
#22053=DIRECTION('center_axis',(-2.44929359829471E-16,-1.22460635382238E-16,
-1.));
#22054=DIRECTION('ref_axis',(2.99942050284817E-32,-1.,1.22460635382238E-16));
#22055=DIRECTION('center_axis',(-2.44929359829471E-16,-1.22460635382238E-16,
-1.));
#22056=DIRECTION('ref_axis',(2.99942050284817E-32,-1.,1.22460635382238E-16));
#22057=DIRECTION('',(4.01685164633802E-17,-0.819152044288988,0.573576436351052));
#22058=DIRECTION('center_axis',(-2.44929359829471E-16,-1.22460635382238E-16,
-1.));
#22059=DIRECTION('ref_axis',(2.99942050284817E-32,-1.,1.22460635382238E-16));
#22060=DIRECTION('center_axis',(-2.44929359829471E-16,-1.22460635382238E-16,
-1.));
#22061=DIRECTION('ref_axis',(2.99942050284817E-32,-1.,1.22460635382238E-16));
#22062=DIRECTION('center_axis',(2.44929359829471E-16,1.22460635382238E-16,
1.));
#22063=DIRECTION('ref_axis',(-2.99942050284817E-32,1.,-1.22460635382238E-16));
#22064=DIRECTION('',(-2.40802902274083E-16,0.819152044288993,-0.573576436351044));
#22065=DIRECTION('center_axis',(-2.44929359829471E-16,0.,-1.));
#22066=DIRECTION('ref_axis',(-1.,0.,2.44929359829471E-16));
#22067=DIRECTION('center_axis',(-2.44929359829471E-16,-1.22460635382238E-16,
-1.));
#22068=DIRECTION('ref_axis',(2.99942050284817E-32,-1.,1.22460635382238E-16));
#22069=DIRECTION('center_axis',(-2.44929359829471E-16,-1.22460635382238E-16,
-1.));
#22070=DIRECTION('ref_axis',(2.99942050284817E-32,-1.,1.22460635382238E-16));
#22071=DIRECTION('',(2.44929359829471E-16,0.,1.));
#22072=DIRECTION('center_axis',(-2.44929359829471E-16,-1.22460635382238E-16,
-1.));
#22073=DIRECTION('ref_axis',(2.99942050284817E-32,-1.,1.22460635382238E-16));
#22074=DIRECTION('center_axis',(-2.44929359829471E-16,-1.22460635382238E-16,
-1.));
#22075=DIRECTION('ref_axis',(2.99942050284817E-32,-1.,1.22460635382238E-16));
#22076=DIRECTION('center_axis',(-2.44929359829471E-16,-1.22460635382238E-16,
-1.));
#22077=DIRECTION('ref_axis',(2.99942050284817E-32,-1.,1.22460635382238E-16));
#22078=DIRECTION('',(4.01685164633802E-17,-0.819152044288988,0.573576436351052));
#22079=DIRECTION('center_axis',(-2.44929359829471E-16,-1.22460635382238E-16,
-1.));
#22080=DIRECTION('ref_axis',(2.99942050284817E-32,-1.,1.22460635382238E-16));
#22081=DIRECTION('center_axis',(-2.44929359829471E-16,-1.22460635382238E-16,
-1.));
#22082=DIRECTION('ref_axis',(2.99942050284817E-32,-1.,1.22460635382238E-16));
#22083=DIRECTION('center_axis',(2.44929359829471E-16,1.22460635382238E-16,
1.));
#22084=DIRECTION('ref_axis',(-2.99942050284817E-32,1.,-1.22460635382238E-16));
#22085=DIRECTION('',(-2.40802902274083E-16,0.819152044288993,-0.573576436351044));
#22086=DIRECTION('center_axis',(-2.44929359829471E-16,0.,-1.));
#22087=DIRECTION('ref_axis',(-1.,0.,2.44929359829471E-16));
#22088=DIRECTION('center_axis',(-2.44929359829471E-16,-1.22460635382238E-16,
-1.));
#22089=DIRECTION('ref_axis',(2.99942050284817E-32,-1.,1.22460635382238E-16));
#22090=DIRECTION('center_axis',(-2.44929359829471E-16,-1.22460635382238E-16,
-1.));
#22091=DIRECTION('ref_axis',(2.99942050284817E-32,-1.,1.22460635382238E-16));
#22092=DIRECTION('',(2.44929359829471E-16,0.,1.));
#22093=DIRECTION('center_axis',(-2.44929359829471E-16,-1.22460635382238E-16,
-1.));
#22094=DIRECTION('ref_axis',(2.99942050284817E-32,-1.,1.22460635382238E-16));
#22095=DIRECTION('center_axis',(-2.44929359829471E-16,-1.22460635382238E-16,
-1.));
#22096=DIRECTION('ref_axis',(2.99942050284817E-32,-1.,1.22460635382238E-16));
#22097=DIRECTION('center_axis',(-2.44929359829471E-16,-1.22460635382238E-16,
-1.));
#22098=DIRECTION('ref_axis',(2.99942050284817E-32,-1.,1.22460635382238E-16));
#22099=DIRECTION('',(4.01685164633802E-17,-0.819152044288988,0.573576436351052));
#22100=DIRECTION('center_axis',(-2.44929359829471E-16,-1.22460635382238E-16,
-1.));
#22101=DIRECTION('ref_axis',(2.99942050284817E-32,-1.,1.22460635382238E-16));
#22102=DIRECTION('center_axis',(-2.44929359829471E-16,-1.22460635382238E-16,
-1.));
#22103=DIRECTION('ref_axis',(2.99942050284817E-32,-1.,1.22460635382238E-16));
#22104=DIRECTION('center_axis',(2.44929359829471E-16,1.22460635382238E-16,
1.));
#22105=DIRECTION('ref_axis',(-2.99942050284817E-32,1.,-1.22460635382238E-16));
#22106=DIRECTION('',(-2.40802902274083E-16,0.819152044288993,-0.573576436351044));
#22107=DIRECTION('center_axis',(-2.44929359829471E-16,0.,-1.));
#22108=DIRECTION('ref_axis',(-1.,0.,2.44929359829471E-16));
#22109=DIRECTION('center_axis',(-2.44929359829471E-16,-1.22460635382238E-16,
-1.));
#22110=DIRECTION('ref_axis',(2.99942050284817E-32,-1.,1.22460635382238E-16));
#22111=DIRECTION('center_axis',(-2.44929359829471E-16,-1.22460635382238E-16,
-1.));
#22112=DIRECTION('ref_axis',(2.99942050284817E-32,-1.,1.22460635382238E-16));
#22113=DIRECTION('',(2.44929359829471E-16,0.,1.));
#22114=DIRECTION('center_axis',(-2.44929359829471E-16,-1.22460635382238E-16,
-1.));
#22115=DIRECTION('ref_axis',(2.99942050284817E-32,-1.,1.22460635382238E-16));
#22116=DIRECTION('center_axis',(-2.44929359829471E-16,-1.22460635382238E-16,
-1.));
#22117=DIRECTION('ref_axis',(2.99942050284817E-32,-1.,1.22460635382238E-16));
#22118=DIRECTION('center_axis',(-2.44929359829471E-16,-1.22460635382238E-16,
-1.));
#22119=DIRECTION('ref_axis',(2.99942050284817E-32,-1.,1.22460635382238E-16));
#22120=DIRECTION('',(4.01685164633802E-17,-0.819152044288988,0.573576436351052));
#22121=DIRECTION('center_axis',(-2.44929359829471E-16,-1.22460635382238E-16,
-1.));
#22122=DIRECTION('ref_axis',(2.99942050284817E-32,-1.,1.22460635382238E-16));
#22123=DIRECTION('center_axis',(-2.44929359829471E-16,-1.22460635382238E-16,
-1.));
#22124=DIRECTION('ref_axis',(2.99942050284817E-32,-1.,1.22460635382238E-16));
#22125=DIRECTION('center_axis',(2.44929359829471E-16,1.22460635382238E-16,
1.));
#22126=DIRECTION('ref_axis',(-2.99942050284817E-32,1.,-1.22460635382238E-16));
#22127=DIRECTION('',(-2.40802902274083E-16,0.819152044288993,-0.573576436351044));
#22128=DIRECTION('center_axis',(-2.44929359829471E-16,0.,-1.));
#22129=DIRECTION('ref_axis',(-1.,0.,2.44929359829471E-16));
#22130=DIRECTION('center_axis',(-2.44929359829471E-16,-1.22460635382238E-16,
-1.));
#22131=DIRECTION('ref_axis',(2.99942050284817E-32,-1.,1.22460635382238E-16));
#22132=DIRECTION('center_axis',(-2.44929359829471E-16,-1.22460635382238E-16,
-1.));
#22133=DIRECTION('ref_axis',(2.99942050284817E-32,-1.,1.22460635382238E-16));
#22134=DIRECTION('',(2.44929359829471E-16,0.,1.));
#22135=DIRECTION('center_axis',(-2.44929359829471E-16,-1.22460635382238E-16,
-1.));
#22136=DIRECTION('ref_axis',(2.99942050284817E-32,-1.,1.22460635382238E-16));
#22137=DIRECTION('center_axis',(-2.44929359829471E-16,-1.22460635382238E-16,
-1.));
#22138=DIRECTION('ref_axis',(2.99942050284817E-32,-1.,1.22460635382238E-16));
#22139=DIRECTION('center_axis',(-2.44929359829471E-16,-1.22460635382238E-16,
-1.));
#22140=DIRECTION('ref_axis',(2.99942050284817E-32,-1.,1.22460635382238E-16));
#22141=DIRECTION('',(4.01685164633802E-17,-0.819152044288988,0.573576436351052));
#22142=DIRECTION('center_axis',(-2.44929359829471E-16,-1.22460635382238E-16,
-1.));
#22143=DIRECTION('ref_axis',(2.99942050284817E-32,-1.,1.22460635382238E-16));
#22144=DIRECTION('center_axis',(-2.44929359829471E-16,-1.22460635382238E-16,
-1.));
#22145=DIRECTION('ref_axis',(2.99942050284817E-32,-1.,1.22460635382238E-16));
#22146=DIRECTION('center_axis',(2.44929359829471E-16,1.22460635382238E-16,
1.));
#22147=DIRECTION('ref_axis',(-2.99942050284817E-32,1.,-1.22460635382238E-16));
#22148=DIRECTION('',(-2.40802902274083E-16,0.819152044288993,-0.573576436351044));
#22149=DIRECTION('center_axis',(-2.44929359829471E-16,0.,-1.));
#22150=DIRECTION('ref_axis',(-1.,0.,2.44929359829471E-16));
#22151=DIRECTION('center_axis',(-2.44929359829471E-16,-1.22460635382238E-16,
-1.));
#22152=DIRECTION('ref_axis',(2.99942050284817E-32,-1.,1.22460635382238E-16));
#22153=DIRECTION('center_axis',(-2.44929359829471E-16,-1.22460635382238E-16,
-1.));
#22154=DIRECTION('ref_axis',(2.99942050284817E-32,-1.,1.22460635382238E-16));
#22155=DIRECTION('',(2.44929359829471E-16,0.,1.));
#22156=DIRECTION('center_axis',(-2.44929359829471E-16,-1.22460635382238E-16,
-1.));
#22157=DIRECTION('ref_axis',(2.99942050284817E-32,-1.,1.22460635382238E-16));
#22158=DIRECTION('center_axis',(-2.44929359829471E-16,-1.22460635382238E-16,
-1.));
#22159=DIRECTION('ref_axis',(2.99942050284817E-32,-1.,1.22460635382238E-16));
#22160=DIRECTION('center_axis',(-2.44929359829471E-16,-1.22460635382238E-16,
-1.));
#22161=DIRECTION('ref_axis',(2.99942050284817E-32,-1.,1.22460635382238E-16));
#22162=DIRECTION('',(4.01685164633802E-17,-0.819152044288988,0.573576436351052));
#22163=DIRECTION('center_axis',(-2.44929359829471E-16,-1.22460635382238E-16,
-1.));
#22164=DIRECTION('ref_axis',(2.99942050284817E-32,-1.,1.22460635382238E-16));
#22165=DIRECTION('center_axis',(-2.44929359829471E-16,-1.22460635382238E-16,
-1.));
#22166=DIRECTION('ref_axis',(2.99942050284817E-32,-1.,1.22460635382238E-16));
#22167=DIRECTION('center_axis',(2.44929359829471E-16,1.22460635382238E-16,
1.));
#22168=DIRECTION('ref_axis',(-2.99942050284817E-32,1.,-1.22460635382238E-16));
#22169=DIRECTION('',(-2.40802902274083E-16,0.819152044288993,-0.573576436351044));
#22170=DIRECTION('center_axis',(-2.44929359829471E-16,0.,-1.));
#22171=DIRECTION('ref_axis',(-1.,0.,2.44929359829471E-16));
#22172=DIRECTION('center_axis',(-2.44929359829471E-16,-1.22460635382238E-16,
-1.));
#22173=DIRECTION('ref_axis',(2.99942050284817E-32,-1.,1.22460635382238E-16));
#22174=DIRECTION('center_axis',(-2.44929359829471E-16,-1.22460635382238E-16,
-1.));
#22175=DIRECTION('ref_axis',(2.99942050284817E-32,-1.,1.22460635382238E-16));
#22176=DIRECTION('',(2.44929359829471E-16,0.,1.));
#22177=DIRECTION('center_axis',(-2.44929359829471E-16,-1.22460635382238E-16,
-1.));
#22178=DIRECTION('ref_axis',(2.99942050284817E-32,-1.,1.22460635382238E-16));
#22179=DIRECTION('center_axis',(-2.44929359829471E-16,-1.22460635382238E-16,
-1.));
#22180=DIRECTION('ref_axis',(2.99942050284817E-32,-1.,1.22460635382238E-16));
#22181=DIRECTION('center_axis',(-2.44929359829471E-16,-1.22460635382238E-16,
-1.));
#22182=DIRECTION('ref_axis',(2.99942050284817E-32,-1.,1.22460635382238E-16));
#22183=DIRECTION('',(4.01685164633802E-17,-0.819152044288988,0.573576436351052));
#22184=DIRECTION('center_axis',(-2.44929359829471E-16,-1.22460635382238E-16,
-1.));
#22185=DIRECTION('ref_axis',(2.99942050284817E-32,-1.,1.22460635382238E-16));
#22186=DIRECTION('center_axis',(-2.44929359829471E-16,-1.22460635382238E-16,
-1.));
#22187=DIRECTION('ref_axis',(2.99942050284817E-32,-1.,1.22460635382238E-16));
#22188=DIRECTION('center_axis',(2.44929359829471E-16,1.22460635382238E-16,
1.));
#22189=DIRECTION('ref_axis',(-2.99942050284817E-32,1.,-1.22460635382238E-16));
#22190=DIRECTION('',(-2.40802902274083E-16,0.819152044288993,-0.573576436351044));
#22191=DIRECTION('center_axis',(2.44929359829471E-16,0.,1.));
#22192=DIRECTION('ref_axis',(1.,0.,-2.44929359829471E-16));
#22193=DIRECTION('center_axis',(-2.44929359829471E-16,0.,-1.));
#22194=DIRECTION('ref_axis',(-1.,0.,2.44929359829471E-16));
#22195=DIRECTION('center_axis',(-2.44929359829471E-16,0.,-1.));
#22196=DIRECTION('ref_axis',(-1.,0.,2.44929359829471E-16));
#22197=DIRECTION('center_axis',(-2.44929359829471E-16,0.,-1.));
#22198=DIRECTION('ref_axis',(-1.,0.,2.44929359829471E-16));
#22199=DIRECTION('center_axis',(-2.44929359829471E-16,0.,-1.));
#22200=DIRECTION('ref_axis',(-1.,0.,2.44929359829471E-16));
#22201=DIRECTION('center_axis',(-2.44929359829471E-16,0.,-1.));
#22202=DIRECTION('ref_axis',(-1.,0.,2.44929359829471E-16));
#22203=DIRECTION('center_axis',(-2.44929359829471E-16,0.,-1.));
#22204=DIRECTION('ref_axis',(-1.,0.,2.44929359829471E-16));
#22205=DIRECTION('center_axis',(-2.44929359829471E-16,0.,-1.));
#22206=DIRECTION('ref_axis',(-1.,0.,2.44929359829471E-16));
#22207=DIRECTION('center_axis',(-2.44929359829471E-16,0.,-1.));
#22208=DIRECTION('ref_axis',(-1.,0.,2.44929359829471E-16));
#22209=DIRECTION('center_axis',(-2.44929359829471E-16,0.,-1.));
#22210=DIRECTION('ref_axis',(-1.,0.,2.44929359829471E-16));
#22211=DIRECTION('center_axis',(-2.44929359829471E-16,0.,-1.));
#22212=DIRECTION('ref_axis',(-1.,0.,2.44929359829471E-16));
#22213=DIRECTION('center_axis',(-2.44929359829471E-16,0.,-1.));
#22214=DIRECTION('ref_axis',(-1.,0.,2.44929359829471E-16));
#22215=DIRECTION('center_axis',(-2.44929359829471E-16,0.,-1.));
#22216=DIRECTION('ref_axis',(-1.,0.,2.44929359829471E-16));
#22217=DIRECTION('center_axis',(-2.44929359829471E-16,0.,-1.));
#22218=DIRECTION('ref_axis',(-1.,0.,2.44929359829471E-16));
#22219=DIRECTION('center_axis',(-2.44929359829471E-16,0.,-1.));
#22220=DIRECTION('ref_axis',(-1.,0.,2.44929359829471E-16));
#22221=DIRECTION('center_axis',(-2.44929359829471E-16,0.,-1.));
#22222=DIRECTION('ref_axis',(-1.,0.,2.44929359829471E-16));
#22223=DIRECTION('center_axis',(-2.44929359829471E-16,0.,-1.));
#22224=DIRECTION('ref_axis',(-1.,0.,2.44929359829471E-16));
#22225=DIRECTION('center_axis',(-2.44929359829471E-16,0.,-1.));
#22226=DIRECTION('ref_axis',(-1.,0.,2.44929359829471E-16));
#22227=DIRECTION('center_axis',(-2.44929359829471E-16,0.,-1.));
#22228=DIRECTION('ref_axis',(-1.,0.,2.44929359829471E-16));
#22229=DIRECTION('center_axis',(-2.44929359829471E-16,0.,-1.));
#22230=DIRECTION('ref_axis',(-1.,0.,2.44929359829471E-16));
#22231=DIRECTION('center_axis',(-2.44929359829471E-16,0.,-1.));
#22232=DIRECTION('ref_axis',(-1.,0.,2.44929359829471E-16));
#22233=DIRECTION('center_axis',(-2.44929359829471E-16,0.,-1.));
#22234=DIRECTION('ref_axis',(-1.,0.,2.44929359829471E-16));
#22235=DIRECTION('center_axis',(-2.44929359829471E-16,0.,-1.));
#22236=DIRECTION('ref_axis',(-1.,0.,2.44929359829471E-16));
#22237=DIRECTION('center_axis',(-2.44929359829471E-16,0.,-1.));
#22238=DIRECTION('ref_axis',(-1.,0.,2.44929359829471E-16));
#22239=DIRECTION('center_axis',(-2.44929359829471E-16,0.,-1.));
#22240=DIRECTION('ref_axis',(-1.,0.,2.44929359829471E-16));
#22241=DIRECTION('center_axis',(-2.44929359829471E-16,0.,-1.));
#22242=DIRECTION('ref_axis',(-1.,0.,2.44929359829471E-16));
#22243=DIRECTION('center_axis',(-2.44929359829471E-16,0.,-1.));
#22244=DIRECTION('ref_axis',(-1.,0.,2.44929359829471E-16));
#22245=DIRECTION('center_axis',(-2.44929359829471E-16,0.,-1.));
#22246=DIRECTION('ref_axis',(-1.,0.,2.44929359829471E-16));
#22247=DIRECTION('center_axis',(-2.44929359829471E-16,0.,-1.));
#22248=DIRECTION('ref_axis',(-1.,0.,2.44929359829471E-16));
#22249=DIRECTION('center_axis',(-2.44929359829471E-16,0.,-1.));
#22250=DIRECTION('ref_axis',(-1.,0.,2.44929359829471E-16));
#22251=DIRECTION('center_axis',(-2.44929359829471E-16,0.,-1.));
#22252=DIRECTION('ref_axis',(-1.,0.,2.44929359829471E-16));
#22253=DIRECTION('center_axis',(-2.44929359829471E-16,0.,-1.));
#22254=DIRECTION('ref_axis',(-1.,0.,2.44929359829471E-16));
#22255=DIRECTION('center_axis',(-2.44929359829471E-16,0.,-1.));
#22256=DIRECTION('ref_axis',(-1.,0.,2.44929359829471E-16));
#22257=DIRECTION('center_axis',(-2.44929359829471E-16,0.,-1.));
#22258=DIRECTION('ref_axis',(-1.,0.,2.44929359829471E-16));
#22259=DIRECTION('center_axis',(-2.44929359829471E-16,0.,-1.));
#22260=DIRECTION('ref_axis',(-1.,0.,2.44929359829471E-16));
#22261=DIRECTION('center_axis',(-2.44929359829471E-16,0.,-1.));
#22262=DIRECTION('ref_axis',(-1.,0.,2.44929359829471E-16));
#22263=DIRECTION('center_axis',(-2.44929359829471E-16,0.,-1.));
#22264=DIRECTION('ref_axis',(-1.,0.,2.44929359829471E-16));
#22265=DIRECTION('center_axis',(-2.44929359829471E-16,0.,-1.));
#22266=DIRECTION('ref_axis',(-1.,0.,2.44929359829471E-16));
#22267=DIRECTION('center_axis',(-2.44929359829471E-16,0.,-1.));
#22268=DIRECTION('ref_axis',(-1.,0.,2.44929359829471E-16));
#22269=DIRECTION('center_axis',(-2.44929359829471E-16,0.,-1.));
#22270=DIRECTION('ref_axis',(-1.,0.,2.44929359829471E-16));
#22271=DIRECTION('',(0.70710678118655,8.65956056235496E-17,-0.707106781186545));
#22272=DIRECTION('center_axis',(-2.44929359829471E-16,0.,-1.));
#22273=DIRECTION('ref_axis',(-1.,0.,2.44929359829471E-16));
#22274=DIRECTION('center_axis',(-2.44929359829471E-16,0.,-1.));
#22275=DIRECTION('ref_axis',(-1.,0.,2.44929359829471E-16));
#22276=DIRECTION('center_axis',(-2.44929359829471E-16,0.,-1.));
#22277=DIRECTION('ref_axis',(-1.,0.,2.44929359829471E-16));
#22278=DIRECTION('center_axis',(-2.44929359829471E-16,0.,-1.));
#22279=DIRECTION('ref_axis',(-1.,0.,2.44929359829471E-16));
#22280=DIRECTION('center_axis',(-2.44929359829471E-16,0.,-1.));
#22281=DIRECTION('ref_axis',(-1.,0.,2.44929359829471E-16));
#22282=DIRECTION('center_axis',(-2.44929359829471E-16,0.,-1.));
#22283=DIRECTION('ref_axis',(-1.,0.,2.44929359829471E-16));
#22284=DIRECTION('center_axis',(-2.44929359829471E-16,0.,-1.));
#22285=DIRECTION('ref_axis',(-1.,0.,2.44929359829471E-16));
#22286=DIRECTION('center_axis',(-2.44929359829471E-16,0.,-1.));
#22287=DIRECTION('ref_axis',(-1.,0.,2.44929359829471E-16));
#22288=DIRECTION('center_axis',(-2.44929359829471E-16,0.,-1.));
#22289=DIRECTION('ref_axis',(-1.,0.,2.44929359829471E-16));
#22290=DIRECTION('center_axis',(-2.44929359829471E-16,0.,-1.));
#22291=DIRECTION('ref_axis',(-1.,0.,2.44929359829471E-16));
#22292=DIRECTION('center_axis',(-2.44929359829471E-16,0.,-1.));
#22293=DIRECTION('ref_axis',(-1.,0.,2.44929359829471E-16));
#22294=DIRECTION('center_axis',(-2.44929359829471E-16,0.,-1.));
#22295=DIRECTION('ref_axis',(-1.,0.,2.44929359829471E-16));
#22296=DIRECTION('center_axis',(-2.44929359829471E-16,0.,-1.));
#22297=DIRECTION('ref_axis',(-1.,0.,2.44929359829471E-16));
#22298=DIRECTION('center_axis',(-2.44929359829471E-16,0.,-1.));
#22299=DIRECTION('ref_axis',(-1.,0.,2.44929359829471E-16));
#22300=DIRECTION('center_axis',(-2.44929359829471E-16,0.,-1.));
#22301=DIRECTION('ref_axis',(-1.,0.,2.44929359829471E-16));
#22302=DIRECTION('center_axis',(-2.44929359829471E-16,0.,-1.));
#22303=DIRECTION('ref_axis',(-1.,0.,2.44929359829471E-16));
#22304=DIRECTION('center_axis',(-2.44929359829471E-16,0.,-1.));
#22305=DIRECTION('ref_axis',(-1.,0.,2.44929359829471E-16));
#22306=DIRECTION('center_axis',(-2.44929359829471E-16,0.,-1.));
#22307=DIRECTION('ref_axis',(-1.,0.,2.44929359829471E-16));
#22308=DIRECTION('center_axis',(-2.44929359829471E-16,0.,-1.));
#22309=DIRECTION('ref_axis',(-1.,0.,2.44929359829471E-16));
#22310=DIRECTION('center_axis',(-2.44929359829471E-16,0.,-1.));
#22311=DIRECTION('ref_axis',(-1.,0.,2.44929359829471E-16));
#22312=DIRECTION('center_axis',(-2.44929359829471E-16,0.,-1.));
#22313=DIRECTION('ref_axis',(-1.,0.,2.44929359829471E-16));
#22314=DIRECTION('center_axis',(-2.44929359829471E-16,0.,-1.));
#22315=DIRECTION('ref_axis',(-1.,0.,2.44929359829471E-16));
#22316=DIRECTION('center_axis',(-2.44929359829471E-16,0.,-1.));
#22317=DIRECTION('ref_axis',(-1.,0.,2.44929359829471E-16));
#22318=DIRECTION('center_axis',(-2.44929359829471E-16,0.,-1.));
#22319=DIRECTION('ref_axis',(-1.,0.,2.44929359829471E-16));
#22320=DIRECTION('center_axis',(-2.44929359829471E-16,0.,-1.));
#22321=DIRECTION('ref_axis',(-1.,0.,2.44929359829471E-16));
#22322=DIRECTION('center_axis',(-2.44929359829471E-16,0.,-1.));
#22323=DIRECTION('ref_axis',(-1.,0.,2.44929359829471E-16));
#22324=DIRECTION('center_axis',(-2.44929359829471E-16,0.,-1.));
#22325=DIRECTION('ref_axis',(-1.,0.,2.44929359829471E-16));
#22326=DIRECTION('center_axis',(-2.44929359829471E-16,0.,-1.));
#22327=DIRECTION('ref_axis',(-1.,0.,2.44929359829471E-16));
#22328=DIRECTION('center_axis',(-2.44929359829471E-16,0.,-1.));
#22329=DIRECTION('ref_axis',(-1.,0.,2.44929359829471E-16));
#22330=DIRECTION('center_axis',(-2.44929359829471E-16,0.,-1.));
#22331=DIRECTION('ref_axis',(-1.,0.,2.44929359829471E-16));
#22332=DIRECTION('center_axis',(-2.44929359829471E-16,0.,-1.));
#22333=DIRECTION('ref_axis',(-1.,0.,2.44929359829471E-16));
#22334=DIRECTION('center_axis',(-2.44929359829471E-16,0.,-1.));
#22335=DIRECTION('ref_axis',(-1.,0.,2.44929359829471E-16));
#22336=DIRECTION('center_axis',(-2.44929359829471E-16,0.,-1.));
#22337=DIRECTION('ref_axis',(-1.,0.,2.44929359829471E-16));
#22338=DIRECTION('center_axis',(-2.44929359829471E-16,0.,-1.));
#22339=DIRECTION('ref_axis',(-1.,0.,2.44929359829471E-16));
#22340=DIRECTION('center_axis',(-2.44929359829471E-16,0.,-1.));
#22341=DIRECTION('ref_axis',(-1.,0.,2.44929359829471E-16));
#22342=DIRECTION('center_axis',(-2.44929359829471E-16,0.,-1.));
#22343=DIRECTION('ref_axis',(-1.,0.,2.44929359829471E-16));
#22344=DIRECTION('center_axis',(-2.44929359829471E-16,0.,-1.));
#22345=DIRECTION('ref_axis',(-1.,0.,2.44929359829471E-16));
#22346=DIRECTION('center_axis',(-2.44929359829471E-16,0.,-1.));
#22347=DIRECTION('ref_axis',(-1.,0.,2.44929359829471E-16));
#22348=DIRECTION('center_axis',(-2.44929359829471E-16,0.,-1.));
#22349=DIRECTION('ref_axis',(-1.,0.,2.44929359829471E-16));
#22350=DIRECTION('center_axis',(-2.44929359829471E-16,0.,-1.));
#22351=DIRECTION('ref_axis',(-1.,0.,2.44929359829471E-16));
#22352=DIRECTION('center_axis',(-2.44929359829471E-16,0.,-1.));
#22353=DIRECTION('ref_axis',(-1.,0.,2.44929359829471E-16));
#22354=DIRECTION('center_axis',(-2.44929359829471E-16,0.,-1.));
#22355=DIRECTION('ref_axis',(-1.,0.,2.44929359829471E-16));
#22356=DIRECTION('center_axis',(-2.44929359829471E-16,0.,-1.));
#22357=DIRECTION('ref_axis',(-1.,0.,2.44929359829471E-16));
#22358=DIRECTION('center_axis',(-2.44929359829471E-16,0.,-1.));
#22359=DIRECTION('ref_axis',(-1.,0.,2.44929359829471E-16));
#22360=DIRECTION('center_axis',(-2.44929359829471E-16,0.,-1.));
#22361=DIRECTION('ref_axis',(-1.,0.,2.44929359829471E-16));
#22362=DIRECTION('center_axis',(-2.44929359829471E-16,0.,-1.));
#22363=DIRECTION('ref_axis',(-1.,0.,2.44929359829471E-16));
#22364=DIRECTION('center_axis',(-2.44929359829471E-16,0.,-1.));
#22365=DIRECTION('ref_axis',(-1.,0.,2.44929359829471E-16));
#22366=DIRECTION('center_axis',(-2.44929359829471E-16,0.,-1.));
#22367=DIRECTION('ref_axis',(-1.,0.,2.44929359829471E-16));
#22368=DIRECTION('center_axis',(-2.44929359829471E-16,0.,-1.));
#22369=DIRECTION('ref_axis',(-1.,0.,2.44929359829471E-16));
#22370=DIRECTION('center_axis',(-2.44929359829471E-16,0.,-1.));
#22371=DIRECTION('ref_axis',(-1.,0.,2.44929359829471E-16));
#22372=DIRECTION('center_axis',(-2.44929359829471E-16,0.,-1.));
#22373=DIRECTION('ref_axis',(-1.,0.,2.44929359829471E-16));
#22374=DIRECTION('center_axis',(-2.44929359829471E-16,0.,-1.));
#22375=DIRECTION('ref_axis',(-1.,0.,2.44929359829471E-16));
#22376=DIRECTION('center_axis',(-2.44929359829471E-16,0.,-1.));
#22377=DIRECTION('ref_axis',(-1.,0.,2.44929359829471E-16));
#22378=DIRECTION('center_axis',(-2.44929359829471E-16,0.,-1.));
#22379=DIRECTION('ref_axis',(-1.,0.,2.44929359829471E-16));
#22380=DIRECTION('center_axis',(-2.44929359829471E-16,0.,-1.));
#22381=DIRECTION('ref_axis',(-1.,0.,2.44929359829471E-16));
#22382=DIRECTION('center_axis',(-2.44929359829471E-16,0.,-1.));
#22383=DIRECTION('ref_axis',(-1.,0.,2.44929359829471E-16));
#22384=DIRECTION('center_axis',(-2.44929359829471E-16,0.,-1.));
#22385=DIRECTION('ref_axis',(-1.,0.,2.44929359829471E-16));
#22386=DIRECTION('center_axis',(-2.44929359829471E-16,0.,-1.));
#22387=DIRECTION('ref_axis',(-1.,0.,2.44929359829471E-16));
#22388=DIRECTION('center_axis',(-2.44929359829471E-16,0.,-1.));
#22389=DIRECTION('ref_axis',(-1.,0.,2.44929359829471E-16));
#22390=DIRECTION('center_axis',(-2.44929359829471E-16,0.,-1.));
#22391=DIRECTION('ref_axis',(-1.,0.,2.44929359829471E-16));
#22392=DIRECTION('center_axis',(-2.44929359829471E-16,0.,-1.));
#22393=DIRECTION('ref_axis',(-1.,0.,2.44929359829471E-16));
#22394=DIRECTION('center_axis',(-2.44929359829471E-16,0.,-1.));
#22395=DIRECTION('ref_axis',(-1.,0.,2.44929359829471E-16));
#22396=DIRECTION('center_axis',(-2.44929359829471E-16,0.,-1.));
#22397=DIRECTION('ref_axis',(-1.,0.,2.44929359829471E-16));
#22398=DIRECTION('center_axis',(-2.44929359829471E-16,0.,-1.));
#22399=DIRECTION('ref_axis',(-1.,0.,2.44929359829471E-16));
#22400=DIRECTION('center_axis',(-2.44929359829471E-16,0.,-1.));
#22401=DIRECTION('ref_axis',(-1.,0.,2.44929359829471E-16));
#22402=DIRECTION('center_axis',(-2.44929359829471E-16,0.,-1.));
#22403=DIRECTION('ref_axis',(-1.,0.,2.44929359829471E-16));
#22404=DIRECTION('center_axis',(-2.44929359829471E-16,0.,-1.));
#22405=DIRECTION('ref_axis',(-1.,0.,2.44929359829471E-16));
#22406=DIRECTION('center_axis',(-2.44929359829471E-16,0.,-1.));
#22407=DIRECTION('ref_axis',(-1.,0.,2.44929359829471E-16));
#22408=DIRECTION('center_axis',(-2.44929359829471E-16,0.,-1.));
#22409=DIRECTION('ref_axis',(-1.,0.,2.44929359829471E-16));
#22410=DIRECTION('center_axis',(-2.44929359829471E-16,0.,-1.));
#22411=DIRECTION('ref_axis',(-1.,0.,2.44929359829471E-16));
#22412=DIRECTION('center_axis',(-2.44929359829471E-16,0.,-1.));
#22413=DIRECTION('ref_axis',(-1.,0.,2.44929359829471E-16));
#22414=DIRECTION('center_axis',(-2.44929359829471E-16,0.,-1.));
#22415=DIRECTION('ref_axis',(-1.,0.,2.44929359829471E-16));
#22416=DIRECTION('center_axis',(-2.44929359829471E-16,0.,-1.));
#22417=DIRECTION('ref_axis',(-1.,0.,2.44929359829471E-16));
#22418=DIRECTION('center_axis',(-2.44929359829471E-16,0.,-1.));
#22419=DIRECTION('ref_axis',(-1.,0.,2.44929359829471E-16));
#22420=DIRECTION('center_axis',(-2.44929359829471E-16,0.,-1.));
#22421=DIRECTION('ref_axis',(-1.,0.,2.44929359829471E-16));
#22422=DIRECTION('center_axis',(-2.44929359829471E-16,0.,-1.));
#22423=DIRECTION('ref_axis',(-1.,0.,2.44929359829471E-16));
#22424=DIRECTION('center_axis',(-2.44929359829471E-16,0.,-1.));
#22425=DIRECTION('ref_axis',(-1.,0.,2.44929359829471E-16));
#22426=DIRECTION('center_axis',(-2.44929359829471E-16,0.,-1.));
#22427=DIRECTION('ref_axis',(-1.,0.,2.44929359829471E-16));
#22428=DIRECTION('center_axis',(-2.44929359829471E-16,0.,-1.));
#22429=DIRECTION('ref_axis',(-1.,0.,2.44929359829471E-16));
#22430=DIRECTION('',(-0.70710678118655,8.65956056235496E-17,0.707106781186545));
#22431=DIRECTION('center_axis',(-2.44929359829471E-16,0.,-1.));
#22432=DIRECTION('ref_axis',(-1.,0.,2.44929359829471E-16));
#22433=DIRECTION('center_axis',(-2.44929359829471E-16,0.,-1.));
#22434=DIRECTION('ref_axis',(-1.,0.,2.44929359829471E-16));
#22435=DIRECTION('center_axis',(-2.44929359829471E-16,0.,-1.));
#22436=DIRECTION('ref_axis',(-1.,0.,2.44929359829471E-16));
#22437=DIRECTION('center_axis',(-2.44929359829471E-16,0.,-1.));
#22438=DIRECTION('ref_axis',(-1.,0.,2.44929359829471E-16));
#22439=DIRECTION('center_axis',(-2.44929359829471E-16,0.,-1.));
#22440=DIRECTION('ref_axis',(-1.,0.,2.44929359829471E-16));
#22441=DIRECTION('center_axis',(-2.44929359829471E-16,0.,-1.));
#22442=DIRECTION('ref_axis',(-1.,0.,2.44929359829471E-16));
#22443=DIRECTION('center_axis',(-2.44929359829471E-16,0.,-1.));
#22444=DIRECTION('ref_axis',(-1.,0.,2.44929359829471E-16));
#22445=DIRECTION('center_axis',(-2.44929359829471E-16,0.,-1.));
#22446=DIRECTION('ref_axis',(-1.,0.,2.44929359829471E-16));
#22447=DIRECTION('center_axis',(-2.44929359829471E-16,0.,-1.));
#22448=DIRECTION('ref_axis',(-1.,0.,2.44929359829471E-16));
#22449=DIRECTION('center_axis',(-2.44929359829471E-16,0.,-1.));
#22450=DIRECTION('ref_axis',(-1.,0.,2.44929359829471E-16));
#22451=DIRECTION('center_axis',(-2.44929359829471E-16,0.,-1.));
#22452=DIRECTION('ref_axis',(-1.,0.,2.44929359829471E-16));
#22453=DIRECTION('center_axis',(-2.44929359829471E-16,0.,-1.));
#22454=DIRECTION('ref_axis',(-1.,0.,2.44929359829471E-16));
#22455=DIRECTION('center_axis',(-2.44929359829471E-16,0.,-1.));
#22456=DIRECTION('ref_axis',(-1.,0.,2.44929359829471E-16));
#22457=DIRECTION('center_axis',(-2.44929359829471E-16,0.,-1.));
#22458=DIRECTION('ref_axis',(-1.,0.,2.44929359829471E-16));
#22459=DIRECTION('center_axis',(-2.44929359829471E-16,0.,-1.));
#22460=DIRECTION('ref_axis',(-1.,0.,2.44929359829471E-16));
#22461=DIRECTION('center_axis',(-2.44929359829471E-16,0.,-1.));
#22462=DIRECTION('ref_axis',(-1.,0.,2.44929359829471E-16));
#22463=DIRECTION('center_axis',(-2.44929359829471E-16,0.,-1.));
#22464=DIRECTION('ref_axis',(-1.,0.,2.44929359829471E-16));
#22465=DIRECTION('center_axis',(-2.44929359829471E-16,0.,-1.));
#22466=DIRECTION('ref_axis',(-1.,0.,2.44929359829471E-16));
#22467=DIRECTION('center_axis',(-2.44929359829471E-16,0.,-1.));
#22468=DIRECTION('ref_axis',(-1.,0.,2.44929359829471E-16));
#22469=DIRECTION('center_axis',(-2.44929359829471E-16,0.,-1.));
#22470=DIRECTION('ref_axis',(-1.,0.,2.44929359829471E-16));
#22471=DIRECTION('center_axis',(-2.44929359829471E-16,0.,-1.));
#22472=DIRECTION('ref_axis',(-1.,0.,2.44929359829471E-16));
#22473=DIRECTION('center_axis',(-2.44929359829471E-16,0.,-1.));
#22474=DIRECTION('ref_axis',(-1.,0.,2.44929359829471E-16));
#22475=DIRECTION('center_axis',(-2.44929359829471E-16,0.,-1.));
#22476=DIRECTION('ref_axis',(-1.,0.,2.44929359829471E-16));
#22477=DIRECTION('center_axis',(-2.44929359829471E-16,0.,-1.));
#22478=DIRECTION('ref_axis',(-1.,0.,2.44929359829471E-16));
#22479=DIRECTION('center_axis',(-2.44929359829471E-16,0.,-1.));
#22480=DIRECTION('ref_axis',(-1.,0.,2.44929359829471E-16));
#22481=DIRECTION('center_axis',(-2.44929359829471E-16,0.,-1.));
#22482=DIRECTION('ref_axis',(-1.,0.,2.44929359829471E-16));
#22483=DIRECTION('center_axis',(-2.44929359829471E-16,0.,-1.));
#22484=DIRECTION('ref_axis',(-1.,0.,2.44929359829471E-16));
#22485=DIRECTION('center_axis',(-2.44929359829471E-16,0.,-1.));
#22486=DIRECTION('ref_axis',(-1.,0.,2.44929359829471E-16));
#22487=DIRECTION('center_axis',(-2.44929359829471E-16,0.,-1.));
#22488=DIRECTION('ref_axis',(-1.,0.,2.44929359829471E-16));
#22489=DIRECTION('center_axis',(-2.44929359829471E-16,0.,-1.));
#22490=DIRECTION('ref_axis',(-1.,0.,2.44929359829471E-16));
#22491=DIRECTION('center_axis',(-2.44929359829471E-16,0.,-1.));
#22492=DIRECTION('ref_axis',(-1.,0.,2.44929359829471E-16));
#22493=DIRECTION('center_axis',(-2.44929359829471E-16,0.,-1.));
#22494=DIRECTION('ref_axis',(-1.,0.,2.44929359829471E-16));
#22495=DIRECTION('center_axis',(-2.44929359829471E-16,0.,-1.));
#22496=DIRECTION('ref_axis',(-1.,0.,2.44929359829471E-16));
#22497=DIRECTION('center_axis',(-2.44929359829471E-16,0.,-1.));
#22498=DIRECTION('ref_axis',(-1.,0.,2.44929359829471E-16));
#22499=DIRECTION('center_axis',(-2.44929359829471E-16,0.,-1.));
#22500=DIRECTION('ref_axis',(-1.,0.,2.44929359829471E-16));
#22501=DIRECTION('center_axis',(-2.44929359829471E-16,0.,-1.));
#22502=DIRECTION('ref_axis',(-1.,0.,2.44929359829471E-16));
#22503=DIRECTION('center_axis',(-2.44929359829471E-16,0.,-1.));
#22504=DIRECTION('ref_axis',(-1.,0.,2.44929359829471E-16));
#22505=DIRECTION('center_axis',(-2.44929359829471E-16,0.,-1.));
#22506=DIRECTION('ref_axis',(-1.,0.,2.44929359829471E-16));
#22507=DIRECTION('center_axis',(-2.44929359829471E-16,0.,-1.));
#22508=DIRECTION('ref_axis',(-1.,0.,2.44929359829471E-16));
#22509=DIRECTION('center_axis',(-2.44929359829471E-16,0.,-1.));
#22510=DIRECTION('ref_axis',(-1.,0.,2.44929359829471E-16));
#22511=DIRECTION('',(2.44929359829471E-16,0.,1.));
#22512=DIRECTION('center_axis',(-2.44929359829471E-16,0.,-1.));
#22513=DIRECTION('ref_axis',(-1.,0.,2.44929359829471E-16));
#22514=DIRECTION('',(-2.44929359829471E-16,0.,-1.));
#22515=DIRECTION('',(-2.44929359829471E-16,0.,-1.));
#22516=DIRECTION('center_axis',(-2.44929359829471E-16,0.,-1.));
#22517=DIRECTION('ref_axis',(-1.,0.,2.44929359829471E-16));
#22518=DIRECTION('',(-2.44929359829471E-16,0.,-1.));
#22519=DIRECTION('',(-2.44929359829471E-16,0.,-1.));
#22520=DIRECTION('center_axis',(-2.44929359829471E-16,0.,-1.));
#22521=DIRECTION('ref_axis',(-1.,0.,2.44929359829471E-16));
#22522=DIRECTION('',(-2.44929359829471E-16,0.,-1.));
#22523=DIRECTION('',(-2.44929359829471E-16,0.,-1.));
#22524=DIRECTION('center_axis',(-2.44929359829471E-16,0.,-1.));
#22525=DIRECTION('ref_axis',(-1.,0.,2.44929359829471E-16));
#22526=DIRECTION('',(-2.44929359829471E-16,0.,-1.));
#22527=DIRECTION('',(-2.44929359829471E-16,0.,-1.));
#22528=DIRECTION('center_axis',(-2.44929359829471E-16,0.,-1.));
#22529=DIRECTION('ref_axis',(-1.,0.,2.44929359829471E-16));
#22530=DIRECTION('',(-2.44929359829471E-16,0.,-1.));
#22531=DIRECTION('',(-2.44929359829471E-16,0.,-1.));
#22532=DIRECTION('center_axis',(-2.44929359829471E-16,0.,-1.));
#22533=DIRECTION('ref_axis',(-1.,0.,2.44929359829471E-16));
#22534=DIRECTION('',(-2.44929359829471E-16,0.,-1.));
#22535=DIRECTION('',(-2.44929359829471E-16,0.,-1.));
#22536=DIRECTION('center_axis',(-2.44929359829471E-16,0.,-1.));
#22537=DIRECTION('ref_axis',(-1.,0.,2.44929359829471E-16));
#22538=DIRECTION('',(-2.44929359829471E-16,0.,-1.));
#22539=DIRECTION('',(-2.44929359829471E-16,0.,-1.));
#22540=DIRECTION('center_axis',(-2.44929359829471E-16,0.,-1.));
#22541=DIRECTION('ref_axis',(-1.,0.,2.44929359829471E-16));
#22542=DIRECTION('',(-2.44929359829471E-16,0.,-1.));
#22543=DIRECTION('',(-2.44929359829471E-16,0.,-1.));
#22544=DIRECTION('center_axis',(-2.44929359829471E-16,0.,-1.));
#22545=DIRECTION('ref_axis',(-1.,0.,2.44929359829471E-16));
#22546=DIRECTION('',(-2.44929359829471E-16,0.,-1.));
#22547=DIRECTION('',(-2.44929359829471E-16,0.,-1.));
#22548=DIRECTION('center_axis',(-2.44929359829471E-16,0.,-1.));
#22549=DIRECTION('ref_axis',(-1.,0.,2.44929359829471E-16));
#22550=DIRECTION('',(-2.44929359829471E-16,0.,-1.));
#22551=DIRECTION('',(-2.44929359829471E-16,0.,-1.));
#22552=DIRECTION('center_axis',(-2.44929359829471E-16,0.,-1.));
#22553=DIRECTION('ref_axis',(-1.,0.,2.44929359829471E-16));
#22554=DIRECTION('',(-2.44929359829471E-16,0.,-1.));
#22555=DIRECTION('',(-2.44929359829471E-16,0.,-1.));
#22556=DIRECTION('center_axis',(-2.44929359829471E-16,0.,-1.));
#22557=DIRECTION('ref_axis',(-1.,0.,2.44929359829471E-16));
#22558=DIRECTION('',(-2.44929359829471E-16,0.,-1.));
#22559=DIRECTION('',(-2.44929359829471E-16,0.,-1.));
#22560=DIRECTION('center_axis',(-2.44929359829471E-16,0.,-1.));
#22561=DIRECTION('ref_axis',(-1.,0.,2.44929359829471E-16));
#22562=DIRECTION('',(-2.44929359829471E-16,0.,-1.));
#22563=DIRECTION('',(-2.44929359829471E-16,0.,-1.));
#22564=DIRECTION('center_axis',(-2.44929359829471E-16,0.,-1.));
#22565=DIRECTION('ref_axis',(-1.,0.,2.44929359829471E-16));
#22566=DIRECTION('',(-2.44929359829471E-16,0.,-1.));
#22567=DIRECTION('',(-2.44929359829471E-16,0.,-1.));
#22568=DIRECTION('center_axis',(-2.44929359829471E-16,0.,-1.));
#22569=DIRECTION('ref_axis',(-1.,0.,2.44929359829471E-16));
#22570=DIRECTION('',(-2.44929359829471E-16,0.,-1.));
#22571=DIRECTION('',(-2.44929359829471E-16,0.,-1.));
#22572=DIRECTION('center_axis',(-2.44929359829471E-16,0.,-1.));
#22573=DIRECTION('ref_axis',(-1.,0.,2.44929359829471E-16));
#22574=DIRECTION('',(-2.44929359829471E-16,0.,-1.));
#22575=DIRECTION('',(-2.44929359829471E-16,0.,-1.));
#22576=DIRECTION('center_axis',(-2.44929359829471E-16,0.,-1.));
#22577=DIRECTION('ref_axis',(-1.,0.,2.44929359829471E-16));
#22578=DIRECTION('',(-2.44929359829471E-16,0.,-1.));
#22579=DIRECTION('',(-2.44929359829471E-16,0.,-1.));
#22580=DIRECTION('center_axis',(-2.44929359829471E-16,0.,-1.));
#22581=DIRECTION('ref_axis',(-1.,0.,2.44929359829471E-16));
#22582=DIRECTION('',(-2.44929359829471E-16,0.,-1.));
#22583=DIRECTION('',(-2.44929359829471E-16,0.,-1.));
#22584=DIRECTION('center_axis',(-2.44929359829471E-16,0.,-1.));
#22585=DIRECTION('ref_axis',(-1.,0.,2.44929359829471E-16));
#22586=DIRECTION('',(-2.44929359829471E-16,0.,-1.));
#22587=DIRECTION('',(-2.44929359829471E-16,0.,-1.));
#22588=DIRECTION('center_axis',(-2.44929359829471E-16,0.,-1.));
#22589=DIRECTION('ref_axis',(-1.,0.,2.44929359829471E-16));
#22590=DIRECTION('',(-2.44929359829471E-16,0.,-1.));
#22591=DIRECTION('',(-2.44929359829471E-16,0.,-1.));
#22592=DIRECTION('center_axis',(-2.44929359829471E-16,0.,-1.));
#22593=DIRECTION('ref_axis',(-1.,0.,2.44929359829471E-16));
#22594=DIRECTION('',(-2.44929359829471E-16,0.,-1.));
#22595=DIRECTION('',(-2.44929359829471E-16,0.,-1.));
#22596=DIRECTION('center_axis',(-2.44929359829471E-16,0.,-1.));
#22597=DIRECTION('ref_axis',(-1.,0.,2.44929359829471E-16));
#22598=DIRECTION('',(-2.44929359829471E-16,0.,-1.));
#22599=DIRECTION('',(-2.44929359829471E-16,0.,-1.));
#22600=DIRECTION('center_axis',(-2.44929359829471E-16,0.,-1.));
#22601=DIRECTION('ref_axis',(-1.,0.,2.44929359829471E-16));
#22602=DIRECTION('',(-2.44929359829471E-16,0.,-1.));
#22603=DIRECTION('',(-2.44929359829471E-16,0.,-1.));
#22604=DIRECTION('center_axis',(-2.44929359829471E-16,0.,-1.));
#22605=DIRECTION('ref_axis',(-1.,0.,2.44929359829471E-16));
#22606=DIRECTION('',(-2.44929359829471E-16,0.,-1.));
#22607=DIRECTION('',(-2.44929359829471E-16,0.,-1.));
#22608=DIRECTION('center_axis',(-2.44929359829471E-16,0.,-1.));
#22609=DIRECTION('ref_axis',(-1.,0.,2.44929359829471E-16));
#22610=DIRECTION('',(-2.44929359829471E-16,0.,-1.));
#22611=DIRECTION('',(-2.44929359829471E-16,0.,-1.));
#22612=DIRECTION('center_axis',(-2.44929359829471E-16,0.,-1.));
#22613=DIRECTION('ref_axis',(-1.,0.,2.44929359829471E-16));
#22614=DIRECTION('',(-2.44929359829471E-16,0.,-1.));
#22615=DIRECTION('',(-2.44929359829471E-16,0.,-1.));
#22616=DIRECTION('center_axis',(-2.44929359829471E-16,0.,-1.));
#22617=DIRECTION('ref_axis',(-1.,0.,2.44929359829471E-16));
#22618=DIRECTION('',(-2.44929359829471E-16,0.,-1.));
#22619=DIRECTION('',(-2.44929359829471E-16,0.,-1.));
#22620=DIRECTION('center_axis',(-2.44929359829471E-16,0.,-1.));
#22621=DIRECTION('ref_axis',(-1.,0.,2.44929359829471E-16));
#22622=DIRECTION('',(-2.44929359829471E-16,0.,-1.));
#22623=DIRECTION('',(-2.44929359829471E-16,0.,-1.));
#22624=DIRECTION('center_axis',(-2.44929359829471E-16,0.,-1.));
#22625=DIRECTION('ref_axis',(-1.,0.,2.44929359829471E-16));
#22626=DIRECTION('',(-2.44929359829471E-16,0.,-1.));
#22627=DIRECTION('',(-2.44929359829471E-16,0.,-1.));
#22628=DIRECTION('center_axis',(-2.44929359829471E-16,0.,-1.));
#22629=DIRECTION('ref_axis',(-1.,0.,2.44929359829471E-16));
#22630=DIRECTION('',(-2.44929359829471E-16,0.,-1.));
#22631=DIRECTION('',(-2.44929359829471E-16,0.,-1.));
#22632=DIRECTION('center_axis',(-2.44929359829471E-16,0.,-1.));
#22633=DIRECTION('ref_axis',(-1.,0.,2.44929359829471E-16));
#22634=DIRECTION('',(-2.44929359829471E-16,0.,-1.));
#22635=DIRECTION('',(-2.44929359829471E-16,0.,-1.));
#22636=DIRECTION('center_axis',(-2.44929359829471E-16,0.,-1.));
#22637=DIRECTION('ref_axis',(-1.,0.,2.44929359829471E-16));
#22638=DIRECTION('',(-2.44929359829471E-16,0.,-1.));
#22639=DIRECTION('',(-2.44929359829471E-16,0.,-1.));
#22640=DIRECTION('center_axis',(-2.44929359829471E-16,0.,-1.));
#22641=DIRECTION('ref_axis',(-1.,0.,2.44929359829471E-16));
#22642=DIRECTION('',(-2.44929359829471E-16,0.,-1.));
#22643=DIRECTION('',(-2.44929359829471E-16,0.,-1.));
#22644=DIRECTION('center_axis',(-2.44929359829471E-16,0.,-1.));
#22645=DIRECTION('ref_axis',(-1.,0.,2.44929359829471E-16));
#22646=DIRECTION('',(-2.44929359829471E-16,0.,-1.));
#22647=DIRECTION('',(-2.44929359829471E-16,0.,-1.));
#22648=DIRECTION('center_axis',(-2.44929359829471E-16,0.,-1.));
#22649=DIRECTION('ref_axis',(-1.,0.,2.44929359829471E-16));
#22650=DIRECTION('',(-2.44929359829471E-16,0.,-1.));
#22651=DIRECTION('',(-2.44929359829471E-16,0.,-1.));
#22652=DIRECTION('center_axis',(-2.44929359829471E-16,0.,-1.));
#22653=DIRECTION('ref_axis',(-1.,0.,2.44929359829471E-16));
#22654=DIRECTION('',(-2.44929359829471E-16,0.,-1.));
#22655=DIRECTION('',(-2.44929359829471E-16,0.,-1.));
#22656=DIRECTION('center_axis',(-2.44929359829471E-16,0.,-1.));
#22657=DIRECTION('ref_axis',(-1.,0.,2.44929359829471E-16));
#22658=DIRECTION('',(-2.44929359829471E-16,0.,-1.));
#22659=DIRECTION('',(-2.44929359829471E-16,0.,-1.));
#22660=DIRECTION('center_axis',(-2.44929359829471E-16,0.,-1.));
#22661=DIRECTION('ref_axis',(-1.,0.,2.44929359829471E-16));
#22662=DIRECTION('',(-2.44929359829471E-16,0.,-1.));
#22663=DIRECTION('',(-2.44929359829471E-16,0.,-1.));
#22664=DIRECTION('center_axis',(-2.44929359829471E-16,0.,-1.));
#22665=DIRECTION('ref_axis',(-1.,0.,2.44929359829471E-16));
#22666=DIRECTION('',(-2.44929359829471E-16,0.,-1.));
#22667=DIRECTION('',(-2.44929359829471E-16,0.,-1.));
#22668=DIRECTION('center_axis',(-2.44929359829471E-16,0.,-1.));
#22669=DIRECTION('ref_axis',(-1.,0.,2.44929359829471E-16));
#22670=DIRECTION('',(-2.44929359829471E-16,0.,-1.));
#22671=DIRECTION('',(-2.44929359829471E-16,0.,-1.));
#22672=DIRECTION('center_axis',(-2.44929359829471E-16,0.,-1.));
#22673=DIRECTION('ref_axis',(-1.,0.,2.44929359829471E-16));
#22674=DIRECTION('',(-2.44929359829471E-16,0.,-1.));
#22675=DIRECTION('',(-2.44929359829471E-16,0.,-1.));
#22676=DIRECTION('center_axis',(-2.44929359829471E-16,0.,-1.));
#22677=DIRECTION('ref_axis',(-1.,0.,2.44929359829471E-16));
#22678=DIRECTION('',(-2.44929359829471E-16,0.,-1.));
#22679=DIRECTION('',(-2.44929359829471E-16,0.,-1.));
#22680=DIRECTION('center_axis',(-2.44929359829471E-16,0.,-1.));
#22681=DIRECTION('ref_axis',(-1.,0.,2.44929359829471E-16));
#22682=DIRECTION('',(-2.44929359829471E-16,0.,-1.));
#22683=DIRECTION('',(-2.44929359829471E-16,0.,-1.));
#22684=DIRECTION('center_axis',(-2.44929359829471E-16,0.,-1.));
#22685=DIRECTION('ref_axis',(-1.,0.,2.44929359829471E-16));
#22686=DIRECTION('',(-2.44929359829471E-16,0.,-1.));
#22687=DIRECTION('',(-2.44929359829471E-16,0.,-1.));
#22688=DIRECTION('center_axis',(-2.44929359829471E-16,0.,-1.));
#22689=DIRECTION('ref_axis',(-1.,0.,2.44929359829471E-16));
#22690=DIRECTION('',(-2.44929359829471E-16,0.,-1.));
#22691=DIRECTION('',(-2.44929359829471E-16,0.,-1.));
#22692=DIRECTION('center_axis',(-2.44929359829471E-16,0.,-1.));
#22693=DIRECTION('ref_axis',(-1.,0.,2.44929359829471E-16));
#22694=DIRECTION('',(-2.44929359829471E-16,0.,-1.));
#22695=DIRECTION('',(-2.44929359829471E-16,0.,-1.));
#22696=DIRECTION('center_axis',(-2.44929359829471E-16,0.,-1.));
#22697=DIRECTION('ref_axis',(-1.,0.,2.44929359829471E-16));
#22698=DIRECTION('',(-2.44929359829471E-16,0.,-1.));
#22699=DIRECTION('',(-2.44929359829471E-16,0.,-1.));
#22700=DIRECTION('center_axis',(-2.44929359829471E-16,0.,-1.));
#22701=DIRECTION('ref_axis',(-1.,0.,2.44929359829471E-16));
#22702=DIRECTION('',(-2.44929359829471E-16,0.,-1.));
#22703=DIRECTION('',(-2.44929359829471E-16,0.,-1.));
#22704=DIRECTION('center_axis',(-2.44929359829471E-16,0.,-1.));
#22705=DIRECTION('ref_axis',(-1.,0.,2.44929359829471E-16));
#22706=DIRECTION('',(-2.44929359829471E-16,0.,-1.));
#22707=DIRECTION('',(-2.44929359829471E-16,0.,-1.));
#22708=DIRECTION('center_axis',(-2.44929359829471E-16,0.,-1.));
#22709=DIRECTION('ref_axis',(-1.,0.,2.44929359829471E-16));
#22710=DIRECTION('',(-2.44929359829471E-16,0.,-1.));
#22711=DIRECTION('',(-2.44929359829471E-16,0.,-1.));
#22712=DIRECTION('center_axis',(-2.44929359829471E-16,0.,-1.));
#22713=DIRECTION('ref_axis',(-1.,0.,2.44929359829471E-16));
#22714=DIRECTION('',(-2.44929359829471E-16,0.,-1.));
#22715=DIRECTION('',(-2.44929359829471E-16,0.,-1.));
#22716=DIRECTION('center_axis',(-2.44929359829471E-16,0.,-1.));
#22717=DIRECTION('ref_axis',(-1.,0.,2.44929359829471E-16));
#22718=DIRECTION('',(-2.44929359829471E-16,0.,-1.));
#22719=DIRECTION('',(-2.44929359829471E-16,0.,-1.));
#22720=DIRECTION('center_axis',(-2.44929359829471E-16,0.,-1.));
#22721=DIRECTION('ref_axis',(-1.,0.,2.44929359829471E-16));
#22722=DIRECTION('',(-2.44929359829471E-16,0.,-1.));
#22723=DIRECTION('',(-2.44929359829471E-16,0.,-1.));
#22724=DIRECTION('center_axis',(-2.44929359829471E-16,0.,-1.));
#22725=DIRECTION('ref_axis',(-1.,0.,2.44929359829471E-16));
#22726=DIRECTION('',(-2.44929359829471E-16,0.,-1.));
#22727=DIRECTION('',(-2.44929359829471E-16,0.,-1.));
#22728=DIRECTION('center_axis',(-2.44929359829471E-16,0.,-1.));
#22729=DIRECTION('ref_axis',(-1.,0.,2.44929359829471E-16));
#22730=DIRECTION('',(-2.44929359829471E-16,0.,-1.));
#22731=DIRECTION('',(-2.44929359829471E-16,0.,-1.));
#22732=DIRECTION('center_axis',(-2.44929359829471E-16,0.,-1.));
#22733=DIRECTION('ref_axis',(-1.,0.,2.44929359829471E-16));
#22734=DIRECTION('',(-2.44929359829471E-16,0.,-1.));
#22735=DIRECTION('',(-2.44929359829471E-16,0.,-1.));
#22736=DIRECTION('center_axis',(-2.44929359829471E-16,0.,-1.));
#22737=DIRECTION('ref_axis',(-1.,0.,2.44929359829471E-16));
#22738=DIRECTION('',(-2.44929359829471E-16,0.,-1.));
#22739=DIRECTION('',(-2.44929359829471E-16,0.,-1.));
#22740=DIRECTION('center_axis',(-2.44929359829471E-16,0.,-1.));
#22741=DIRECTION('ref_axis',(-1.,0.,2.44929359829471E-16));
#22742=DIRECTION('',(-2.44929359829471E-16,0.,-1.));
#22743=DIRECTION('',(-2.44929359829471E-16,0.,-1.));
#22744=DIRECTION('center_axis',(-2.44929359829471E-16,0.,-1.));
#22745=DIRECTION('ref_axis',(-1.,0.,2.44929359829471E-16));
#22746=DIRECTION('',(-2.44929359829471E-16,0.,-1.));
#22747=DIRECTION('',(-2.44929359829471E-16,0.,-1.));
#22748=DIRECTION('center_axis',(-2.44929359829471E-16,0.,-1.));
#22749=DIRECTION('ref_axis',(-1.,0.,2.44929359829471E-16));
#22750=DIRECTION('',(-2.44929359829471E-16,0.,-1.));
#22751=DIRECTION('',(-2.44929359829471E-16,0.,-1.));
#22752=DIRECTION('center_axis',(-2.44929359829471E-16,0.,-1.));
#22753=DIRECTION('ref_axis',(-1.,0.,2.44929359829471E-16));
#22754=DIRECTION('',(-2.44929359829471E-16,0.,-1.));
#22755=DIRECTION('',(-2.44929359829471E-16,0.,-1.));
#22756=DIRECTION('center_axis',(-2.44929359829471E-16,0.,-1.));
#22757=DIRECTION('ref_axis',(-1.,0.,2.44929359829471E-16));
#22758=DIRECTION('',(-2.44929359829471E-16,0.,-1.));
#22759=DIRECTION('',(-2.44929359829471E-16,0.,-1.));
#22760=DIRECTION('center_axis',(-2.44929359829471E-16,0.,-1.));
#22761=DIRECTION('ref_axis',(-1.,0.,2.44929359829471E-16));
#22762=DIRECTION('',(-2.44929359829471E-16,0.,-1.));
#22763=DIRECTION('',(-2.44929359829471E-16,0.,-1.));
#22764=DIRECTION('center_axis',(-2.44929359829471E-16,0.,-1.));
#22765=DIRECTION('ref_axis',(-1.,0.,2.44929359829471E-16));
#22766=DIRECTION('',(-2.44929359829471E-16,0.,-1.));
#22767=DIRECTION('',(-2.44929359829471E-16,0.,-1.));
#22768=DIRECTION('center_axis',(-2.44929359829471E-16,0.,-1.));
#22769=DIRECTION('ref_axis',(-1.,0.,2.44929359829471E-16));
#22770=DIRECTION('',(-2.44929359829471E-16,0.,-1.));
#22771=DIRECTION('',(-2.44929359829471E-16,0.,-1.));
#22772=DIRECTION('center_axis',(-2.44929359829471E-16,0.,-1.));
#22773=DIRECTION('ref_axis',(-1.,0.,2.44929359829471E-16));
#22774=DIRECTION('',(-2.44929359829471E-16,0.,-1.));
#22775=DIRECTION('',(-2.44929359829471E-16,0.,-1.));
#22776=DIRECTION('center_axis',(-2.44929359829471E-16,0.,-1.));
#22777=DIRECTION('ref_axis',(-1.,0.,2.44929359829471E-16));
#22778=DIRECTION('',(-2.44929359829471E-16,0.,-1.));
#22779=DIRECTION('',(-2.44929359829471E-16,0.,-1.));
#22780=DIRECTION('center_axis',(-2.44929359829471E-16,0.,-1.));
#22781=DIRECTION('ref_axis',(-1.,0.,2.44929359829471E-16));
#22782=DIRECTION('',(-2.44929359829471E-16,0.,-1.));
#22783=DIRECTION('',(-2.44929359829471E-16,0.,-1.));
#22784=DIRECTION('center_axis',(-2.44929359829471E-16,0.,-1.));
#22785=DIRECTION('ref_axis',(-1.,0.,2.44929359829471E-16));
#22786=DIRECTION('',(-2.44929359829471E-16,0.,-1.));
#22787=DIRECTION('',(-2.44929359829471E-16,0.,-1.));
#22788=DIRECTION('center_axis',(-2.44929359829471E-16,0.,-1.));
#22789=DIRECTION('ref_axis',(-1.,0.,2.44929359829471E-16));
#22790=DIRECTION('',(-2.44929359829471E-16,0.,-1.));
#22791=DIRECTION('',(-2.44929359829471E-16,0.,-1.));
#22792=DIRECTION('center_axis',(-2.44929359829471E-16,0.,-1.));
#22793=DIRECTION('ref_axis',(-1.,0.,2.44929359829471E-16));
#22794=DIRECTION('',(-2.44929359829471E-16,0.,-1.));
#22795=DIRECTION('',(-2.44929359829471E-16,0.,-1.));
#22796=DIRECTION('center_axis',(-2.44929359829471E-16,0.,-1.));
#22797=DIRECTION('ref_axis',(-1.,0.,2.44929359829471E-16));
#22798=DIRECTION('',(-2.44929359829471E-16,0.,-1.));
#22799=DIRECTION('',(-2.44929359829471E-16,0.,-1.));
#22800=DIRECTION('center_axis',(-2.44929359829471E-16,0.,-1.));
#22801=DIRECTION('ref_axis',(-1.,0.,2.44929359829471E-16));
#22802=DIRECTION('',(-2.44929359829471E-16,0.,-1.));
#22803=DIRECTION('',(-2.44929359829471E-16,0.,-1.));
#22804=DIRECTION('center_axis',(-2.44929359829471E-16,0.,-1.));
#22805=DIRECTION('ref_axis',(-1.,0.,2.44929359829471E-16));
#22806=DIRECTION('',(-2.44929359829471E-16,0.,-1.));
#22807=DIRECTION('',(-2.44929359829471E-16,0.,-1.));
#22808=DIRECTION('center_axis',(-2.44929359829471E-16,0.,-1.));
#22809=DIRECTION('ref_axis',(-1.,0.,2.44929359829471E-16));
#22810=DIRECTION('',(-2.44929359829471E-16,0.,-1.));
#22811=DIRECTION('',(-2.44929359829471E-16,0.,-1.));
#22812=DIRECTION('center_axis',(-2.44929359829471E-16,0.,-1.));
#22813=DIRECTION('ref_axis',(-1.,0.,2.44929359829471E-16));
#22814=DIRECTION('',(-2.44929359829471E-16,0.,-1.));
#22815=DIRECTION('',(-2.44929359829471E-16,0.,-1.));
#22816=DIRECTION('center_axis',(-2.44929359829471E-16,0.,-1.));
#22817=DIRECTION('ref_axis',(-1.,0.,2.44929359829471E-16));
#22818=DIRECTION('center_axis',(-2.44929359829471E-16,0.,-1.));
#22819=DIRECTION('ref_axis',(-1.,0.,2.44929359829471E-16));
#22820=DIRECTION('',(-2.44929359829471E-16,0.,-1.));
#22821=DIRECTION('',(-2.44929359829471E-16,0.,-1.));
#22822=DIRECTION('center_axis',(-2.44929359829471E-16,0.,-1.));
#22823=DIRECTION('ref_axis',(-1.,0.,2.44929359829471E-16));
#22824=DIRECTION('center_axis',(2.44929359829471E-16,0.,1.));
#22825=DIRECTION('ref_axis',(1.,0.,-2.44929359829471E-16));
#22826=DIRECTION('center_axis',(0.866025403784439,-0.499999999999999,-2.12115047744982E-16));
#22827=DIRECTION('ref_axis',(0.499999999999999,0.866025403784439,-1.22464679914735E-16));
#22828=DIRECTION('',(-2.44929359829471E-16,0.,-1.));
#22829=DIRECTION('center_axis',(-0.866025403784438,-0.500000000000001,2.12115047744981E-16));
#22830=DIRECTION('ref_axis',(0.500000000000001,-0.866025403784438,-1.22464679914736E-16));
#22831=DIRECTION('center_axis',(0.903898417468945,-0.427747181051069,-2.2139126074154E-16));
#22832=DIRECTION('ref_axis',(0.427747181051069,0.903898417468945,-1.04767843223699E-16));
#22833=DIRECTION('',(-2.44929359829471E-16,0.,-1.));
#22834=DIRECTION('center_axis',(-0.82238913392188,-0.568925401443124,2.01427244102199E-16));
#22835=DIRECTION('ref_axis',(0.568925401443124,-0.82238913392188,-1.39346534366189E-16));
#22836=DIRECTION('center_axis',(0.82238913392189,-0.56892540144311,-2.01427244102201E-16));
#22837=DIRECTION('ref_axis',(0.56892540144311,0.82238913392189,-1.39346534366186E-16));
#22838=DIRECTION('',(-2.44929359829471E-16,0.,-1.));
#22839=DIRECTION('center_axis',(-0.903898417468938,-0.427747181051084,2.21391260741539E-16));
#22840=DIRECTION('ref_axis',(0.427747181051084,-0.903898417468938,-1.04767843223703E-16));
#22841=DIRECTION('center_axis',(0.773280000057739,-0.634064698205714,-1.89398975383075E-16));
#22842=DIRECTION('ref_axis',(0.634064698205714,0.773280000057739,-1.55301060621992E-16));
#22843=DIRECTION('',(-2.44929359829471E-16,0.,-1.));
#22844=DIRECTION('center_axis',(-0.935756136317931,-0.352647775185578,2.2919415142485E-16));
#22845=DIRECTION('ref_axis',(0.352647775185578,-0.935756136317931,-8.63737938214907E-17));
#22846=DIRECTION('center_axis',(0.719024815375424,-0.694984399015069,-1.76110287731406E-16));
#22847=DIRECTION('ref_axis',(0.694984399015069,0.719024815375425,-1.7022208394223E-16));
#22848=DIRECTION('',(-2.44929359829471E-16,0.,-1.));
#22849=DIRECTION('center_axis',(-0.961386552468623,-0.275201556558999,2.35471792844802E-16));
#22850=DIRECTION('ref_axis',(0.275201556558999,-0.961386552468623,-6.74049410720695E-17));
#22851=DIRECTION('center_axis',(0.65998463917753,-0.751279093313334,-1.61649615171037E-16));
#22852=DIRECTION('ref_axis',(0.751279093313334,0.65998463917753,-1.840103073785E-16));
#22853=DIRECTION('',(-2.44929359829471E-16,0.,-1.));
#22854=DIRECTION('center_axis',(-0.980619099730252,-0.195923916978581,2.40182408333483E-16));
#22855=DIRECTION('ref_axis',(0.195923916978581,-0.980619099730252,-4.79875195608462E-17));
#22856=DIRECTION('center_axis',(0.59655237409571,-0.802574149197924,-1.46113191092013E-16));
#22857=DIRECTION('ref_axis',(0.802574149197924,0.59655237409571,-1.9657397257873E-16));
#22858=DIRECTION('',(-2.44929359829471E-16,0.,-1.));
#22859=DIRECTION('center_axis',(-0.99332578867394,-0.115342436055841,2.43294649522012E-16));
#22860=DIRECTION('ref_axis',(0.115342436055841,-0.99332578867394,-2.82507490243288E-17));
#22861=DIRECTION('center_axis',(0.529150151388497,-0.848528206535016,-1.29604407833252E-16));
#22862=DIRECTION('ref_axis',(0.848528206535016,0.529150151388497,-2.0782947042387E-16));
#22863=DIRECTION('',(-2.44929359829471E-16,0.,-1.));
#22864=DIRECTION('center_axis',(-0.999422058381221,-0.033993370251312,2.44787804958764E-16));
#22865=DIRECTION('ref_axis',(0.033993370251312,-0.999422058381221,-8.32597441410003E-18));
#22866=DIRECTION('center_axis',(0.458226521727423,-0.888835448654917,-1.12233128623583E-16));
#22867=DIRECTION('ref_axis',(0.888835448654917,0.458226521727423,-2.17701897432789E-16));
#22868=DIRECTION('',(-2.44929359829471E-16,0.,-1.));
#22869=DIRECTION('center_axis',(-0.998867339183009,0.047581915823728,2.44651937940661E-16));
#22870=DIRECTION('ref_axis',(-0.047581915823728,-0.998867339183009,1.16542081821655E-17));
#22871=DIRECTION('center_axis',(0.384253470166307,-0.923227637511546,-9.41149564600862E-17));
#22872=DIRECTION('ref_axis',(0.923227637511546,0.384253470166307,-2.26125554232578E-16));
#22873=DIRECTION('',(-2.44929359829471E-16,0.,-1.));
#22874=DIRECTION('center_axis',(-0.991665322644044,0.128840552099425,2.42887952640291E-16));
#22875=DIRECTION('ref_axis',(-0.128840552099425,-0.991665322644044,3.15568339457877E-17));
#22876=DIRECTION('center_axis',(0.307723275158594,-0.951475898762374,-7.53704647892225E-17));
#22877=DIRECTION('ref_axis',(0.951475898762374,0.307723275158594,-2.33044382777039E-16));
#22878=DIRECTION('',(-2.44929359829471E-16,0.,-1.));
#22879=DIRECTION('center_axis',(-0.977863936996144,0.209241775758096,2.39507588088791E-16));
#22880=DIRECTION('ref_axis',(-0.209241775758096,-0.977863936996144,5.1249454186012E-17));
#22881=DIRECTION('center_axis',(0.229145232525468,-0.973392244889412,-5.61243951104381E-17));
#22882=DIRECTION('ref_axis',(0.973392244889412,0.229145232525468,-2.38412339403735E-16));
#22883=DIRECTION('',(-2.44929359829471E-16,0.,-1.));
#22884=DIRECTION('center_axis',(-0.957555028183728,0.288250529921558,2.34533340054531E-16));
#22885=DIRECTION('ref_axis',(-0.288250529921558,-0.957555028183729,7.06010177641929E-17));
#22886=DIRECTION('center_axis',(0.149042266176187,-0.988830826225127,-3.6504826842067E-17));
#22887=DIRECTION('ref_axis',(0.988830826225127,0.149042266176187,-2.42193701246967E-16));
#22888=DIRECTION('',(-2.44929359829471E-16,0.,-1.));
#22889=DIRECTION('center_axis',(-0.930873748644209,0.365341024366383,2.27998311337486E-16));
#22890=DIRECTION('ref_axis',(-0.365341024366383,-0.930873748644209,8.94827432175012E-17));
#22891=DIRECTION('center_axis',(0.0679474481357467,-0.997688901557916,-1.66423249739346E-17));
#22892=DIRECTION('ref_axis',(0.997688901557916,0.0679474481357467,-2.44363303967548E-16));
#22893=DIRECTION('',(-2.44929359829471E-16,0.,-1.));
#22894=DIRECTION('center_axis',(-0.89799765789082,0.440000234571075,2.19945991475563E-16));
#22895=DIRECTION('ref_axis',(-0.440000234571075,-0.89799765789082,1.0776897577831E-16));
#22896=DIRECTION('center_axis',(-0.0135995489614973,-0.999907521857919,
3.33092882110907E-18));
#22897=DIRECTION('ref_axis',(0.999907521857919,-0.0135995489614973,-2.44906709217332E-16));
#22898=DIRECTION('',(-2.44929359829471E-16,0.,-1.));
#22899=DIRECTION('center_axis',(-0.859145540883353,0.511731315809626,2.10429967328904E-16));
#22900=DIRECTION('ref_axis',(-0.511731315809626,-0.859145540883353,1.25338023585944E-16));
#22901=DIRECTION('center_axis',(-0.0950560433041702,-0.995471922573086,
2.32820158344128E-17));
#22902=DIRECTION('ref_axis',(0.995471922573086,-0.0950560433041702,-2.43820300724038E-16));
#22903=DIRECTION('',(-2.44929359829471E-16,0.,-1.));
#22904=DIRECTION('center_axis',(-0.814575952050343,0.580056909571188,1.99513566468172E-16));
#22905=DIRECTION('ref_axis',(-0.580056909571188,-0.814575952050343,1.42072967525932E-16));
#22906=DIRECTION('center_axis',(-0.175879955361797,-0.984411621884836,4.30781648736008E-17));
#22907=DIRECTION('ref_axis',(0.984411621884836,-0.175879955361797,-2.41111308356944E-16));
#22908=DIRECTION('',(-2.44929359829471E-16,0.,-1.));
#22909=DIRECTION('center_axis',(-0.76458549465201,0.644522320302207,1.87269435740016E-16));
#22910=DIRECTION('ref_axis',(-0.644522320302207,-0.76458549465201,1.57862439307425E-16));
#22911=DIRECTION('center_axis',(-0.255533415334641,-0.966800224269427,6.25876358329519E-17));
#22912=DIRECTION('ref_axis',(0.966800224269427,-0.255533415334641,-2.36797760013299E-16));
#22913=DIRECTION('',(-2.44929359829471E-16,0.,-1.));
#22914=DIRECTION('center_axis',(-0.709506846934496,0.704698541330312,1.73779057814292E-16));
#22915=DIRECTION('ref_axis',(-0.704698541330313,-0.709506846934496,1.72601362600795E-16));
#22916=DIRECTION('center_axis',(-0.333486342588479,-0.942754930672314,8.16805964020677E-17));
#22917=DIRECTION('ref_axis',(0.942754930672314,-0.333486342588479,-2.30908361645647E-16));
#22918=DIRECTION('',(-2.44929359829471E-16,0.,-1.));
#22919=DIRECTION('center_axis',(-0.649706548211022,0.76018510983294,1.59132208930341E-16));
#22920=DIRECTION('ref_axis',(-0.76018510983294,-0.649706548211022,1.86191652303278E-16));
#22921=DIRECTION('center_axis',(-0.409219973253765,-0.912435758555192,1.00229986078478E-16));
#22922=DIRECTION('ref_axis',(0.912435758555192,-0.409219973253765,-2.23482306228441E-16));
#22923=DIRECTION('',(-2.44929359829471E-16,0.,-1.));
#22924=DIRECTION('center_axis',(-0.585582559603238,0.810612771851345,1.43426361450924E-16));
#22925=DIRECTION('ref_axis',(-0.810612771851345,-0.585582559603238,1.98542867279143E-16));
#22926=DIRECTION('center_axis',(-0.48223031251359,-0.876044477006188,1.18112361734319E-16));
#22927=DIRECTION('ref_axis',(0.876044477006188,-0.48223031251359,-2.14569012935269E-16));
#22928=DIRECTION('',(-2.44929359829471E-16,0.,-1.));
#22929=DIRECTION('center_axis',(-0.517561615675617,0.855645939614771,1.26766035199735E-16));
#22930=DIRECTION('ref_axis',(-0.855645939614771,-0.517561615675617,2.09572812230532E-16));
#22931=DIRECTION('center_axis',(-0.552031488606037,-0.833823263999873,1.35208719109986E-16));
#22932=DIRECTION('ref_axis',(0.833823263999873,-0.552031488606037,-2.04227798262409E-16));
#22933=DIRECTION('',(-2.44929359829471E-16,0.,-1.));
#22934=DIRECTION('center_axis',(-0.446096384587331,0.894984924821705,1.09262101899216E-16));
#22935=DIRECTION('ref_axis',(-0.894984924821705,-0.446096384587331,2.19208084693607E-16));
#22936=DIRECTION('center_axis',(-0.618158986220597,-0.786053094742794,1.51405284767845E-16));
#22937=DIRECTION('ref_axis',(0.786053094742794,-0.618158986220597,-1.92527481287327E-16));
#22938=DIRECTION('',(-2.44929359829471E-16,0.,-1.));
#22939=DIRECTION('center_axis',(-0.371662455660338,0.928367933016068,9.10310473375357E-17));
#22940=DIRECTION('ref_axis',(-0.928367933016068,-0.371662455660338,2.27384563519835E-16));
#22941=DIRECTION('center_axis',(-0.680172737770911,-0.733051871829834,1.66594273235688E-16));
#22942=DIRECTION('ref_axis',(0.733051871829834,-0.680172737770911,-1.79545925689076E-16));
#22943=DIRECTION('',(-2.44929359829471E-16,0.,-1.));
#22944=DIRECTION('center_axis',(-0.294755174410915,0.955572805786137,7.21941961748894E-17));
#22945=DIRECTION('ref_axis',(-0.955572805786137,-0.294755174410915,2.3404783559165E-16));
#22946=DIRECTION('center_axis',(-0.737660051971963,-0.675172309654892,1.80674604301267E-16));
#22947=DIRECTION('ref_axis',(0.675172309654892,-0.737660051971963,-1.65369521578358E-16));
#22948=DIRECTION('',(-2.44929359829471E-16,0.,-1.));
#22949=DIRECTION('center_axis',(-0.215886346106968,0.976418499192115,5.28769045479032E-17));
#22950=DIRECTION('ref_axis',(-0.976418499192115,-0.215886346106968,2.39153557932777E-16));
#22951=DIRECTION('center_axis',(-0.790238360232484,-0.612799587154786,1.93552575684433E-16));
#22952=DIRECTION('ref_axis',(0.612799587154786,-0.790238360232484,-1.50092610585586E-16));
#22953=DIRECTION('',(-2.44929359829471E-16,0.,-1.));
#22954=DIRECTION('center_axis',(-0.135580829788419,0.990766288583682,3.32077258452259E-17));
#22955=DIRECTION('ref_axis',(-0.990766288583682,-0.135580829788419,2.42667752803422E-16));
#22956=DIRECTION('center_axis',(-0.837557762585809,-0.54634878450698,2.05142486610346E-16));
#22957=DIRECTION('ref_axis',(0.54634878450698,-0.837557762585809,-1.33816858032904E-16));
#22958=DIRECTION('',(-2.44929359829471E-16,0.,-1.));
#22959=DIRECTION('center_axis',(-0.0543730454168903,0.998520691789656,1.33175552059377E-17));
#22960=DIRECTION('ref_axis',(-0.998520691789656,-0.0543730454168903,2.44567033816521E-16));
#22961=DIRECTION('center_axis',(-0.879303356216429,-0.476262120839485,2.15367208133995E-16));
#22962=DIRECTION('ref_axis',(0.476262120839484,-0.879303356216429,-1.16650576368241E-16));
#22963=DIRECTION('',(-2.44929359829471E-16,0.,-1.));
#22964=DIRECTION('center_axis',(0.0271965826009666,0.999630104536087,-6.66124156600408E-18));
#22965=DIRECTION('ref_axis',(-0.999630104536087,0.0271965826009666,2.44838761570291E-16));
#22966=DIRECTION('center_axis',(-0.915197331086271,-0.40300601133552,2.24158696420601E-16));
#22967=DIRECTION('ref_axis',(0.40300601133552,-0.915197331086272,-9.87080043638374E-17));
#22968=DIRECTION('',(-2.44929359829471E-16,0.,-1.));
#22969=DIRECTION('center_axis',(0.108585221848735,0.994087143864189,-2.65957088743518E-17));
#22970=DIRECTION('ref_axis',(-0.994087143864189,0.108585221848735,2.43481127761363E-16));
#22971=DIRECTION('center_axis',(-0.945000818714665,-0.327067963317431,2.31458445566109E-16));
#22972=DIRECTION('ref_axis',(0.327067963317431,-0.945000818714665,-8.01085468760672E-17));
#22973=DIRECTION('',(-2.44929359829471E-16,0.,-1.));
#22974=DIRECTION('center_axis',(0.1892512443604,0.981928697262709,-4.63531861281235E-17));
#22975=DIRECTION('ref_axis',(-0.981928697262709,0.1892512443604,2.40503167218741E-16));
#22976=DIRECTION('center_axis',(-0.968515481808673,-0.248953331965879,2.3721787694433E-16));
#22977=DIRECTION('ref_axis',(0.248953331965879,-0.968515481808673,-6.09759802258165E-17));
#22978=DIRECTION('',(-2.44929359829471E-16,0.,-1.));
#22979=DIRECTION('center_axis',(0.268657831065104,0.963235677187776,-6.58021905759501E-17));
#22980=DIRECTION('ref_axis',(-0.963235677187776,0.268657831065104,2.35924697778509E-16));
#22981=DIRECTION('center_axis',(-0.985584834165051,-0.169181957264503,2.41398662489681E-16));
#22982=DIRECTION('ref_axis',(0.169181957264503,-0.985584834165051,-4.14376284874917E-17));
#22983=DIRECTION('',(-2.44929359829471E-16,0.,-1.));
#22984=DIRECTION('center_axis',(0.346276544229492,0.938132482603859,-8.48132923020909E-17));
#22985=DIRECTION('ref_axis',(-0.93813248260386,0.346276544229492,2.29776188399395E-16));
#22986=DIRECTION('center_axis',(-0.996095282060112,-0.0882847045505903,
2.43972979764139E-16));
#22987=DIRECTION('ref_axis',(0.0882847045505904,-0.996095282060113,-2.16235161683101E-17));
#22988=DIRECTION('',(-2.44929359829471E-16,0.,-1.));
#22989=DIRECTION('center_axis',(0.421590844123641,0.906786171129178,-1.0325997556117E-16));
#22990=DIRECTION('ref_axis',(-0.906786171129178,0.421590844123641,2.22098556396887E-16));
#22991=DIRECTION('center_axis',(-0.999976880197217,-0.00679993169384408,
2.44923697110976E-16));
#22992=DIRECTION('ref_axis',(0.00679993169384408,-0.999976880197217,-1.66550291665736E-18));
#22993=DIRECTION('',(-2.44929359829471E-16,0.,-1.));
#22994=DIRECTION('center_axis',(0.49409952650774,0.86940534729482,-1.21019480719585E-16));
#22995=DIRECTION('ref_axis',(-0.86940534729482,0.49409952650774,2.12942895145239E-16));
#22996=DIRECTION('center_axis',(-0.997203797181181,0.074730093586415,2.44244487663104E-16));
#22997=DIRECTION('ref_axis',(-0.074730093586415,-0.997203797181181,1.83035939821171E-17));
#22998=DIRECTION('',(-2.44929359829471E-16,0.,-1.));
#22999=DIRECTION('center_axis',(0.563320058063614,0.826238774316,-1.37973621200621E-16));
#23000=DIRECTION('ref_axis',(-0.826238774316,0.563320058063614,2.02370134059504E-16));
#23001=DIRECTION('center_axis',(-0.98779448742195,0.155762802423454,2.41939871447338E-16));
#23002=DIRECTION('ref_axis',(-0.155762802423454,-0.98779448742195,3.8150883482821E-17));
#23003=DIRECTION('',(-2.44929359829471E-16,0.,-1.));
#23004=DIRECTION('center_axis',(0.628791787574343,0.777573718613909,-1.54009569996612E-16));
#23005=DIRECTION('ref_axis',(-0.777573718613909,0.628791787574343,1.90450633120326E-16));
#23006=DIRECTION('center_axis',(-0.971811568323544,0.235758935509419,2.38025185304359E-16));
#23007=DIRECTION('ref_axis',(-0.235758935509419,-0.971811568323544,5.77442851483994E-17));
#23008=DIRECTION('',(-2.44929359829471E-16,0.,-1.));
#23009=DIRECTION('center_axis',(0.690079011482106,0.723734038105076,-1.69020610514066E-16));
#23010=DIRECTION('ref_axis',(-0.723734038105076,0.690079011482105,1.77263714639874E-16));
#23011=DIRECTION('center_axis',(-0.949361403575568,0.314186131777054,2.32526480824571E-16));
#23012=DIRECTION('ref_axis',(-0.314186131777054,-0.949361403575568,7.69534081234516E-17));
#23013=DIRECTION('',(-2.44929359829471E-16,0.,-1.));
#23014=DIRECTION('center_axis',(0.746773873423478,0.665078026980365,-1.82906846754987E-16));
#23015=DIRECTION('ref_axis',(-0.665078026980365,0.746773873423478,1.62897135384948E-16));
#23016=DIRECTION('center_axis',(-0.920593395320402,0.390522471174776,2.25480350979065E-16));
#23017=DIRECTION('ref_axis',(-0.390522471174777,-0.920593395320402,9.56504188638609E-17));
#23018=DIRECTION('',(-2.44929359829471E-16,0.,-1.));
#23019=DIRECTION('center_axis',(0.798499078446234,0.60199603131625,-1.95575868108258E-16));
#23020=DIRECTION('ref_axis',(-0.60199603131625,0.798499078446233,1.47446502570171E-16));
#23021=DIRECTION('center_axis',(-0.885698989906598,0.464259947958503,2.16933686599432E-16));
#23022=DIRECTION('ref_axis',(-0.464259947958503,-0.885698989906598,1.13710891847939E-16));
#23023=DIRECTION('',(-2.44929359829471E-16,0.,-1.));
#23024=DIRECTION('center_axis',(0.844910403845004,0.53490785138608,-2.06943364327016E-16));
#23025=DIRECTION('ref_axis',(-0.53490785138608,0.844910403845004,1.3101463760775E-16));
#23026=DIRECTION('center_axis',(-0.844910403845013,0.534907851386066,2.06943364327019E-16));
#23027=DIRECTION('ref_axis',(-0.534907851386066,-0.844910403845013,1.31014637607747E-16));
#23028=DIRECTION('',(-2.44929359829471E-16,0.,-1.));
#23029=DIRECTION('center_axis',(0.88569898990659,0.464259947958518,-2.1693368659943E-16));
#23030=DIRECTION('ref_axis',(-0.464259947958518,0.88569898990659,1.13710891847943E-16));
#23031=DIRECTION('center_axis',(-0.798499078446244,0.601996031316237,1.95575868108261E-16));
#23032=DIRECTION('ref_axis',(-0.601996031316237,-0.798499078446243,1.47446502570168E-16));
#23033=DIRECTION('',(-2.44929359829471E-16,0.,-1.));
#23034=DIRECTION('center_axis',(0.920593395320395,0.390522471174792,-2.25480350979063E-16));
#23035=DIRECTION('ref_axis',(-0.390522471174792,0.920593395320395,9.56504188638647E-17));
#23036=DIRECTION('center_axis',(-0.746773873423489,0.665078026980353,1.82906846754989E-16));
#23037=DIRECTION('ref_axis',(-0.665078026980353,-0.746773873423489,1.62897135384945E-16));
#23038=DIRECTION('',(-2.44929359829471E-16,0.,-1.));
#23039=DIRECTION('center_axis',(0.949361403575562,0.31418613177707,-2.3252648082457E-16));
#23040=DIRECTION('ref_axis',(-0.31418613177707,0.949361403575562,7.69534081234555E-17));
#23041=DIRECTION('center_axis',(-0.690079011482118,0.723734038105065,1.69020610514069E-16));
#23042=DIRECTION('ref_axis',(-0.723734038105065,-0.690079011482118,1.77263714639871E-16));
#23043=DIRECTION('',(-2.44929359829471E-16,0.,-1.));
#23044=DIRECTION('center_axis',(0.97181156832354,0.235758935509435,-2.38025185304359E-16));
#23045=DIRECTION('ref_axis',(-0.235758935509435,0.97181156832354,5.77442851484034E-17));
#23046=DIRECTION('center_axis',(-0.628791787574355,0.777573718613899,1.54009569996615E-16));
#23047=DIRECTION('ref_axis',(-0.777573718613899,-0.628791787574355,1.90450633120323E-16));
#23048=DIRECTION('',(-2.44929359829471E-16,0.,-1.));
#23049=DIRECTION('center_axis',(0.987794487421947,0.15576280242347,-2.41939871447338E-16));
#23050=DIRECTION('ref_axis',(-0.15576280242347,0.987794487421947,3.81508834828249E-17));
#23051=DIRECTION('center_axis',(-0.563320058063628,0.826238774315991,1.37973621200625E-16));
#23052=DIRECTION('ref_axis',(-0.826238774315991,-0.563320058063628,2.02370134059502E-16));
#23053=DIRECTION('',(-2.44929359829471E-16,0.,-1.));
#23054=DIRECTION('center_axis',(0.99720379718118,0.0747300935864316,-2.44244487663104E-16));
#23055=DIRECTION('ref_axis',(-0.0747300935864316,0.99720379718118,1.83035939821211E-17));
#23056=DIRECTION('center_axis',(-0.494099526507755,0.869405347294812,1.21019480719589E-16));
#23057=DIRECTION('ref_axis',(-0.869405347294812,-0.494099526507755,2.12942895145237E-16));
#23058=DIRECTION('',(-2.44929359829471E-16,0.,-1.));
#23059=DIRECTION('center_axis',(0.999976880197217,-0.00679993169382737,
-2.44923697110976E-16));
#23060=DIRECTION('ref_axis',(0.00679993169382737,0.999976880197217,-1.66550291665327E-18));
#23061=DIRECTION('center_axis',(-0.421590844123656,0.906786171129171,1.03259975561173E-16));
#23062=DIRECTION('ref_axis',(-0.906786171129171,-0.421590844123656,2.22098556396885E-16));
#23063=DIRECTION('',(-2.44929359829471E-16,0.,-1.));
#23064=DIRECTION('center_axis',(0.996095282060114,-0.0882847045505736,-2.4397297976414E-16));
#23065=DIRECTION('ref_axis',(0.0882847045505736,0.996095282060114,-2.1623516168306E-17));
#23066=DIRECTION('center_axis',(-0.346276544229508,0.938132482603854,8.48132923020948E-17));
#23067=DIRECTION('ref_axis',(-0.938132482603854,-0.346276544229508,2.29776188399394E-16));
#23068=DIRECTION('',(-2.44929359829471E-16,0.,-1.));
#23069=DIRECTION('center_axis',(0.985584834165054,-0.169181957264487,-2.41398662489682E-16));
#23070=DIRECTION('ref_axis',(0.169181957264487,0.985584834165054,-4.14376284874876E-17));
#23071=DIRECTION('center_axis',(-0.26865783106512,0.963235677187772,6.58021905759539E-17));
#23072=DIRECTION('ref_axis',(-0.963235677187772,-0.26865783106512,2.35924697778508E-16));
#23073=DIRECTION('',(-2.44929359829471E-16,0.,-1.));
#23074=DIRECTION('center_axis',(0.968515481808677,-0.248953331965864,-2.37217876944331E-16));
#23075=DIRECTION('ref_axis',(0.248953331965864,0.968515481808677,-6.09759802258127E-17));
#23076=DIRECTION('center_axis',(-0.189251244360416,0.981928697262706,4.63531861281275E-17));
#23077=DIRECTION('ref_axis',(-0.981928697262706,-0.189251244360416,2.40503167218741E-16));
#23078=DIRECTION('',(-2.44929359829471E-16,0.,-1.));
#23079=DIRECTION('center_axis',(0.945000818714671,-0.327067963317415,-2.3145844556611E-16));
#23080=DIRECTION('ref_axis',(0.327067963317415,0.945000818714671,-8.01085468760634E-17));
#23081=DIRECTION('center_axis',(-0.108585221848752,0.994087143864187,2.65957088743558E-17));
#23082=DIRECTION('ref_axis',(-0.994087143864187,-0.108585221848752,2.43481127761362E-16));
#23083=DIRECTION('',(-2.44929359829471E-16,0.,-1.));
#23084=DIRECTION('center_axis',(0.915197331086278,-0.403006011335506,-2.24158696420602E-16));
#23085=DIRECTION('ref_axis',(0.403006011335506,0.915197331086278,-9.87080043638338E-17));
#23086=DIRECTION('center_axis',(-0.0271965826009838,0.999630104536087,6.66124156600828E-18));
#23087=DIRECTION('ref_axis',(-0.999630104536087,-0.0271965826009838,2.44838761570291E-16));
#23088=DIRECTION('',(-2.44929359829471E-16,0.,-1.));
#23089=DIRECTION('center_axis',(0.879303356216437,-0.476262120839469,-2.15367208133997E-16));
#23090=DIRECTION('ref_axis',(0.476262120839469,0.879303356216437,-1.16650576368237E-16));
#23091=DIRECTION('center_axis',(0.0543730454168737,0.998520691789657,-1.33175552059336E-17));
#23092=DIRECTION('ref_axis',(-0.998520691789657,0.0543730454168737,2.44567033816521E-16));
#23093=DIRECTION('',(-2.44929359829471E-16,0.,-1.));
#23094=DIRECTION('center_axis',(0.837557762585818,-0.546348784506966,-2.05142486610348E-16));
#23095=DIRECTION('ref_axis',(0.546348784506966,0.837557762585818,-1.33816858032901E-16));
#23096=DIRECTION('center_axis',(0.135580829788402,0.990766288583684,-3.32077258452218E-17));
#23097=DIRECTION('ref_axis',(-0.990766288583684,0.135580829788402,2.42667752803422E-16));
#23098=DIRECTION('',(-2.44929359829471E-16,0.,-1.));
#23099=DIRECTION('center_axis',(0.790238360232494,-0.612799587154772,-1.93552575684435E-16));
#23100=DIRECTION('ref_axis',(0.612799587154772,0.790238360232494,-1.50092610585582E-16));
#23101=DIRECTION('center_axis',(0.215886346106952,0.976418499192119,-5.28769045478992E-17));
#23102=DIRECTION('ref_axis',(-0.976418499192119,0.215886346106952,2.39153557932778E-16));
#23103=DIRECTION('',(-2.44929359829471E-16,0.,-1.));
#23104=DIRECTION('center_axis',(0.737660051971974,-0.675172309654879,-1.8067460430127E-16));
#23105=DIRECTION('ref_axis',(0.675172309654879,0.737660051971974,-1.65369521578355E-16));
#23106=DIRECTION('center_axis',(0.294755174410899,0.955572805786142,-7.21941961748855E-17));
#23107=DIRECTION('ref_axis',(-0.955572805786142,0.294755174410899,2.34047835591651E-16));
#23108=DIRECTION('',(-2.44929359829471E-16,0.,-1.));
#23109=DIRECTION('center_axis',(0.680172737770924,-0.733051871829822,-1.66594273235691E-16));
#23110=DIRECTION('ref_axis',(0.733051871829822,0.680172737770924,-1.79545925689074E-16));
#23111=DIRECTION('center_axis',(0.371662455660323,0.928367933016075,-9.10310473375319E-17));
#23112=DIRECTION('ref_axis',(-0.928367933016075,0.371662455660323,2.27384563519836E-16));
#23113=DIRECTION('',(-2.44929359829471E-16,0.,-1.));
#23114=DIRECTION('center_axis',(0.618158986220609,-0.786053094742784,-1.51405284767848E-16));
#23115=DIRECTION('ref_axis',(0.786053094742784,0.618158986220609,-1.92527481287324E-16));
#23116=DIRECTION('center_axis',(0.446096384587316,0.894984924821712,-1.09262101899213E-16));
#23117=DIRECTION('ref_axis',(-0.894984924821712,0.446096384587316,2.19208084693609E-16));
#23118=DIRECTION('',(-2.44929359829471E-16,0.,-1.));
#23119=DIRECTION('center_axis',(0.552031488606051,-0.833823263999864,-1.3520871910999E-16));
#23120=DIRECTION('ref_axis',(0.833823263999864,0.552031488606051,-2.04227798262407E-16));
#23121=DIRECTION('center_axis',(0.517561615675603,0.85564593961478,-1.26766035199732E-16));
#23122=DIRECTION('ref_axis',(-0.85564593961478,0.517561615675603,2.09572812230534E-16));
#23123=DIRECTION('',(-2.44929359829471E-16,0.,-1.));
#23124=DIRECTION('center_axis',(0.482230312513604,-0.87604447700618,-1.18112361734323E-16));
#23125=DIRECTION('ref_axis',(0.87604447700618,0.482230312513604,-2.14569012935267E-16));
#23126=DIRECTION('center_axis',(0.585582559603225,0.810612771851354,-1.43426361450921E-16));
#23127=DIRECTION('ref_axis',(-0.810612771851354,0.585582559603225,1.98542867279145E-16));
#23128=DIRECTION('',(-2.44929359829471E-16,0.,-1.));
#23129=DIRECTION('center_axis',(0.40921997325378,-0.912435758555185,-1.00229986078481E-16));
#23130=DIRECTION('ref_axis',(0.912435758555185,0.40921997325378,-2.23482306228439E-16));
#23131=DIRECTION('center_axis',(0.649706548211009,0.760185109832951,-1.59132208930338E-16));
#23132=DIRECTION('ref_axis',(-0.760185109832951,0.649706548211009,1.86191652303281E-16));
#23133=DIRECTION('',(-2.44929359829471E-16,0.,-1.));
#23134=DIRECTION('center_axis',(0.333486342588495,-0.942754930672308,-8.16805964020716E-17));
#23135=DIRECTION('ref_axis',(0.942754930672308,0.333486342588495,-2.30908361645646E-16));
#23136=DIRECTION('center_axis',(0.709506846934484,0.704698541330324,-1.73779057814289E-16));
#23137=DIRECTION('ref_axis',(-0.704698541330324,0.709506846934484,1.72601362600798E-16));
#23138=DIRECTION('',(-2.44929359829471E-16,0.,-1.));
#23139=DIRECTION('center_axis',(0.255533415334658,-0.966800224269422,-6.25876358329559E-17));
#23140=DIRECTION('ref_axis',(0.966800224269422,0.255533415334658,-2.36797760013298E-16));
#23141=DIRECTION('center_axis',(0.764585494652,0.64452232030222,-1.87269435740013E-16));
#23142=DIRECTION('ref_axis',(-0.64452232030222,0.764585494652,1.57862439307428E-16));
#23143=DIRECTION('',(-2.44929359829471E-16,0.,-1.));
#23144=DIRECTION('center_axis',(0.175879955361814,-0.984411621884833,-4.30781648736049E-17));
#23145=DIRECTION('ref_axis',(0.984411621884833,0.175879955361814,-2.41111308356943E-16));
#23146=DIRECTION('center_axis',(0.814575952050334,0.580056909571201,-1.9951356646817E-16));
#23147=DIRECTION('ref_axis',(-0.580056909571201,0.814575952050333,1.42072967525936E-16));
#23148=DIRECTION('',(-2.44929359829471E-16,0.,-1.));
#23149=DIRECTION('center_axis',(0.0950560433041868,-0.995471922573084,-2.32820158344169E-17));
#23150=DIRECTION('ref_axis',(0.995471922573084,0.0950560433041868,-2.43820300724038E-16));
#23151=DIRECTION('center_axis',(0.859145540883344,0.51173131580964,-2.10429967328902E-16));
#23152=DIRECTION('ref_axis',(-0.51173131580964,0.859145540883344,1.25338023585948E-16));
#23153=DIRECTION('',(-2.44929359829471E-16,0.,-1.));
#23154=DIRECTION('center_axis',(0.013599548961514,-0.999907521857918,-3.33092882111317E-18));
#23155=DIRECTION('ref_axis',(0.999907521857918,0.013599548961514,-2.44906709217332E-16));
#23156=DIRECTION('center_axis',(0.897997657890813,0.44000023457109,-2.19945991475561E-16));
#23157=DIRECTION('ref_axis',(-0.44000023457109,0.897997657890813,1.07768975778314E-16));
#23158=DIRECTION('',(-2.44929359829471E-16,0.,-1.));
#23159=DIRECTION('center_axis',(-0.0679474481357302,-0.997688901557917,
1.66423249739306E-17));
#23160=DIRECTION('ref_axis',(0.997688901557917,-0.0679474481357302,-2.44363303967548E-16));
#23161=DIRECTION('center_axis',(0.930873748644203,0.365341024366398,-2.27998311337484E-16));
#23162=DIRECTION('ref_axis',(-0.365341024366398,0.930873748644203,8.94827432175049E-17));
#23163=DIRECTION('',(-2.44929359829471E-16,0.,-1.));
#23164=DIRECTION('center_axis',(-0.149042266176171,-0.988830826225129,3.65048268420631E-17));
#23165=DIRECTION('ref_axis',(0.988830826225129,-0.149042266176171,-2.42193701246967E-16));
#23166=DIRECTION('center_axis',(0.957555028183724,0.288250529921574,-2.3453334005453E-16));
#23167=DIRECTION('ref_axis',(-0.288250529921574,0.957555028183724,7.06010177641968E-17));
#23168=DIRECTION('',(-2.44929359829471E-16,0.,-1.));
#23169=DIRECTION('center_axis',(-0.229145232525452,-0.973392244889416,5.61243951104342E-17));
#23170=DIRECTION('ref_axis',(0.973392244889416,-0.229145232525452,-2.38412339403736E-16));
#23171=DIRECTION('center_axis',(0.977863936996141,0.209241775758112,-2.39507588088791E-16));
#23172=DIRECTION('ref_axis',(-0.209241775758112,0.977863936996141,5.12494541860159E-17));
#23173=DIRECTION('',(-2.44929359829471E-16,0.,-1.));
#23174=DIRECTION('center_axis',(-0.307723275158579,-0.951475898762379,7.53704647892187E-17));
#23175=DIRECTION('ref_axis',(0.951475898762379,-0.307723275158579,-2.3304438277704E-16));
#23176=DIRECTION('center_axis',(0.991665322644042,0.128840552099442,-2.42887952640291E-16));
#23177=DIRECTION('ref_axis',(-0.128840552099442,0.991665322644042,3.15568339457918E-17));
#23178=DIRECTION('',(-2.44929359829471E-16,0.,-1.));
#23179=DIRECTION('center_axis',(-0.384253470166292,-0.923227637511553,9.41149564600824E-17));
#23180=DIRECTION('ref_axis',(0.923227637511553,-0.384253470166292,-2.26125554232579E-16));
#23181=DIRECTION('center_axis',(0.998867339183008,0.0475819158237449,-2.44651937940661E-16));
#23182=DIRECTION('ref_axis',(-0.0475819158237449,0.998867339183008,1.16542081821696E-17));
#23183=DIRECTION('',(-2.44929359829471E-16,0.,-1.));
#23184=DIRECTION('center_axis',(-0.458226521727408,-0.888835448654925,1.12233128623579E-16));
#23185=DIRECTION('ref_axis',(0.888835448654925,-0.458226521727408,-2.17701897432791E-16));
#23186=DIRECTION('center_axis',(0.999422058381222,-0.0339933702512953,-2.44787804958765E-16));
#23187=DIRECTION('ref_axis',(0.0339933702512953,0.999422058381222,-8.32597441409594E-18));
#23188=DIRECTION('',(-2.44929359829471E-16,0.,-1.));
#23189=DIRECTION('center_axis',(-0.529150151388483,-0.848528206535025,1.29604407833249E-16));
#23190=DIRECTION('ref_axis',(0.848528206535025,-0.529150151388483,-2.07829470423873E-16));
#23191=DIRECTION('center_axis',(0.993325788673942,-0.115342436055824,-2.43294649522013E-16));
#23192=DIRECTION('ref_axis',(0.115342436055824,0.993325788673942,-2.82507490243247E-17));
#23193=DIRECTION('',(-2.44929359829471E-16,0.,-1.));
#23194=DIRECTION('center_axis',(-0.596552374095697,-0.802574149197934,1.4611319109201E-16));
#23195=DIRECTION('ref_axis',(0.802574149197934,-0.596552374095697,-1.96573972578732E-16));
#23196=DIRECTION('center_axis',(0.980619099730256,-0.195923916978565,-2.40182408333483E-16));
#23197=DIRECTION('ref_axis',(0.195923916978565,0.980619099730256,-4.79875195608422E-17));
#23198=DIRECTION('',(-2.44929359829471E-16,0.,-1.));
#23199=DIRECTION('center_axis',(-0.659984639177518,-0.751279093313345,1.61649615171034E-16));
#23200=DIRECTION('ref_axis',(0.751279093313345,-0.659984639177518,-1.84010307378503E-16));
#23201=DIRECTION('center_axis',(0.961386552468627,-0.275201556558983,-2.35471792844803E-16));
#23202=DIRECTION('ref_axis',(0.275201556558983,0.961386552468627,-6.74049410720656E-17));
#23203=DIRECTION('',(-2.44929359829471E-16,0.,-1.));
#23204=DIRECTION('center_axis',(-0.719024815375413,-0.694984399015081,1.76110287731403E-16));
#23205=DIRECTION('ref_axis',(0.694984399015081,-0.719024815375413,-1.70222083942233E-16));
#23206=DIRECTION('center_axis',(0.935756136317937,-0.352647775185563,-2.29194151424851E-16));
#23207=DIRECTION('ref_axis',(0.352647775185563,0.935756136317937,-8.6373793821487E-17));
#23208=DIRECTION('',(-2.44929359829471E-16,0.,-1.));
#23209=DIRECTION('center_axis',(-0.773280000057729,-0.634064698205726,1.89398975383073E-16));
#23210=DIRECTION('ref_axis',(0.634064698205726,-0.773280000057729,-1.55301060621995E-16));
#23211=DIRECTION('center_axis',(0.,0.,1.));
#23212=DIRECTION('ref_axis',(1.,0.,0.));
#23213=DIRECTION('center_axis',(0.,0.,-1.));
#23214=DIRECTION('ref_axis',(1.,-2.57442419626753E-15,0.));
#23215=DIRECTION('center_axis',(0.,0.,1.));
#23216=DIRECTION('ref_axis',(1.,0.,0.));
#23217=DIRECTION('center_axis',(0.,0.,-1.));
#23218=DIRECTION('ref_axis',(1.,0.,0.));
#23219=DIRECTION('center_axis',(0.,-1.,0.));
#23220=DIRECTION('ref_axis',(-1.,0.,0.));
#23221=DIRECTION('center_axis',(0.,0.,-1.));
#23222=DIRECTION('ref_axis',(1.,0.,0.));
#23223=DIRECTION('center_axis',(0.,0.,-1.));
#23224=DIRECTION('ref_axis',(1.,0.,0.));
#23225=DIRECTION('center_axis',(0.,0.,-1.));
#23226=DIRECTION('ref_axis',(1.,0.,0.));
#23227=DIRECTION('center_axis',(0.,0.,1.));
#23228=DIRECTION('ref_axis',(1.,0.,0.));
#23229=DIRECTION('center_axis',(0.,0.,-1.));
#23230=DIRECTION('ref_axis',(-1.,0.,0.));
#23231=DIRECTION('center_axis',(0.,0.,1.));
#23232=DIRECTION('ref_axis',(1.,0.,0.));
#23233=DIRECTION('',(-0.0871557427476585,1.0673500138323E-17,0.996194698091746));
#23234=DIRECTION('center_axis',(0.,0.,1.));
#23235=DIRECTION('ref_axis',(1.,0.,0.));
#23236=DIRECTION('center_axis',(0.,0.,1.));
#23237=DIRECTION('ref_axis',(1.,0.,0.));
#23238=DIRECTION('',(0.,0.,-1.));
#23239=DIRECTION('center_axis',(0.,0.,1.));
#23240=DIRECTION('ref_axis',(1.,0.,0.));
#23241=DIRECTION('center_axis',(0.,0.,1.));
#23242=DIRECTION('ref_axis',(1.,0.,0.));
#23243=DIRECTION('',(-1.,0.,0.));
#23244=DIRECTION('center_axis',(0.,0.,-1.));
#23245=DIRECTION('ref_axis',(-1.,0.,0.));
#23246=DIRECTION('center_axis',(0.,0.,1.));
#23247=DIRECTION('ref_axis',(1.,0.,0.));
#23248=DIRECTION('',(1.,-1.25844895020639E-16,0.));
#23249=DIRECTION('center_axis',(0.,0.,1.));
#23250=DIRECTION('ref_axis',(1.,0.,0.));
#23251=DIRECTION('center_axis',(0.,1.,0.));
#23252=DIRECTION('ref_axis',(1.,0.,0.));
#23253=DIRECTION('',(-1.,0.,0.));
#23254=DIRECTION('center_axis',(-1.25844895020639E-16,-1.,0.));
#23255=DIRECTION('ref_axis',(-1.,1.25844895020639E-16,0.));
#23256=DIRECTION('',(1.,-1.25844895020639E-16,0.));
#23257=DIRECTION('center_axis',(0.,0.,1.));
#23258=DIRECTION('ref_axis',(1.,0.,0.));
#23259=DIRECTION('center_axis',(-1.22460635382238E-16,-1.,-2.46519032881566E-32));
#23260=DIRECTION('ref_axis',(0.,0.,1.));
#23261=DIRECTION('center_axis',(-1.22460635382238E-16,-1.,-2.46519032881566E-32));
#23262=DIRECTION('ref_axis',(-3.01888774004913E-48,-2.46519032881566E-32,
1.));
#23263=DIRECTION('center_axis',(-1.,1.22460635382238E-16,0.));
#23264=DIRECTION('ref_axis',(0.,0.,-1.));
#23265=DIRECTION('center_axis',(1.22460635382238E-16,1.,2.46519032881566E-32));
#23266=DIRECTION('ref_axis',(-3.01888774004913E-48,-2.46519032881566E-32,
1.));
#23267=DIRECTION('center_axis',(-1.22460635382238E-16,-1.,-2.46519032881566E-32));
#23268=DIRECTION('ref_axis',(-3.01888774004913E-48,-2.46519032881566E-32,
1.));
#23269=DIRECTION('center_axis',(0.,-1.,-2.46519032881566E-32));
#23270=DIRECTION('ref_axis',(-1.,0.,0.));
#23271=DIRECTION('center_axis',(0.,-1.,-2.46519032881566E-32));
#23272=DIRECTION('ref_axis',(-1.,0.,0.));
#23273=DIRECTION('',(-2.85991635543547E-21,0.707106781186549,0.707106781186546));
#23274=DIRECTION('center_axis',(-1.22460635382238E-16,-1.,-2.46519032881566E-32));
#23275=DIRECTION('ref_axis',(-3.01888774004913E-48,-2.46519032881566E-32,
1.));
#23276=DIRECTION('center_axis',(0.,-1.,-2.46519032881566E-32));
#23277=DIRECTION('ref_axis',(1.,0.,0.));
#23278=DIRECTION('center_axis',(0.,-1.,-2.46519032881566E-32));
#23279=DIRECTION('ref_axis',(1.,0.,0.));
#23280=DIRECTION('center_axis',(0.,-1.,-2.46519032881566E-32));
#23281=DIRECTION('ref_axis',(1.,0.,0.));
#23282=DIRECTION('',(0.81915204428899,0.573576436351049,1.00317192905352E-16));
#23283=DIRECTION('center_axis',(0.,-1.,-2.46519032881566E-32));
#23284=DIRECTION('ref_axis',(1.,0.,0.));
#23285=DIRECTION('center_axis',(0.,-1.,-2.46519032881566E-32));
#23286=DIRECTION('ref_axis',(1.,0.,0.));
#23287=DIRECTION('center_axis',(0.,1.,2.46519032881566E-32));
#23288=DIRECTION('ref_axis',(-1.,0.,0.));
#23289=DIRECTION('',(-0.819152044288993,-0.573576436351044,1.00317192905353E-16));
#23290=DIRECTION('center_axis',(-1.22460635382238E-16,-1.,-2.46519032881566E-32));
#23291=DIRECTION('ref_axis',(-3.01888774004913E-48,-2.46519032881566E-32,
1.));
#23292=DIRECTION('center_axis',(0.,-1.,-2.46519032881566E-32));
#23293=DIRECTION('ref_axis',(1.,0.,0.));
#23294=DIRECTION('center_axis',(0.,-1.,-2.46519032881566E-32));
#23295=DIRECTION('ref_axis',(1.,0.,0.));
#23296=DIRECTION('',(1.22460635382238E-16,1.,2.46519032881566E-32));
#23297=DIRECTION('center_axis',(0.,-1.,-2.46519032881566E-32));
#23298=DIRECTION('ref_axis',(1.,0.,0.));
#23299=DIRECTION('center_axis',(0.,-1.,-2.46519032881566E-32));
#23300=DIRECTION('ref_axis',(1.,0.,0.));
#23301=DIRECTION('center_axis',(0.,-1.,-2.46519032881566E-32));
#23302=DIRECTION('ref_axis',(1.,0.,0.));
#23303=DIRECTION('',(0.81915204428899,0.573576436351049,1.00317192905352E-16));
#23304=DIRECTION('center_axis',(0.,-1.,-2.46519032881566E-32));
#23305=DIRECTION('ref_axis',(1.,0.,0.));
#23306=DIRECTION('center_axis',(0.,-1.,-2.46519032881566E-32));
#23307=DIRECTION('ref_axis',(1.,0.,0.));
#23308=DIRECTION('center_axis',(0.,1.,2.46519032881566E-32));
#23309=DIRECTION('ref_axis',(-1.,0.,0.));
#23310=DIRECTION('',(-0.819152044288993,-0.573576436351044,1.00317192905353E-16));
#23311=DIRECTION('center_axis',(-1.22460635382238E-16,-1.,-2.46519032881566E-32));
#23312=DIRECTION('ref_axis',(-3.01888774004913E-48,-2.46519032881566E-32,
1.));
#23313=DIRECTION('center_axis',(0.,-1.,-2.46519032881566E-32));
#23314=DIRECTION('ref_axis',(1.,0.,0.));
#23315=DIRECTION('center_axis',(0.,-1.,-2.46519032881566E-32));
#23316=DIRECTION('ref_axis',(1.,0.,0.));
#23317=DIRECTION('',(1.22460635382238E-16,1.,2.46519032881566E-32));
#23318=DIRECTION('center_axis',(0.,-1.,-2.46519032881566E-32));
#23319=DIRECTION('ref_axis',(1.,0.,0.));
#23320=DIRECTION('center_axis',(0.,-1.,-2.46519032881566E-32));
#23321=DIRECTION('ref_axis',(1.,0.,0.));
#23322=DIRECTION('center_axis',(0.,-1.,-2.46519032881566E-32));
#23323=DIRECTION('ref_axis',(1.,0.,0.));
#23324=DIRECTION('',(0.81915204428899,0.573576436351049,1.00317192905352E-16));
#23325=DIRECTION('center_axis',(0.,-1.,-2.46519032881566E-32));
#23326=DIRECTION('ref_axis',(1.,0.,0.));
#23327=DIRECTION('center_axis',(0.,-1.,-2.46519032881566E-32));
#23328=DIRECTION('ref_axis',(1.,0.,0.));
#23329=DIRECTION('center_axis',(0.,1.,2.46519032881566E-32));
#23330=DIRECTION('ref_axis',(-1.,0.,0.));
#23331=DIRECTION('',(-0.819152044288993,-0.573576436351044,1.00317192905353E-16));
#23332=DIRECTION('center_axis',(-1.22460635382238E-16,-1.,-2.46519032881566E-32));
#23333=DIRECTION('ref_axis',(-3.01888774004913E-48,-2.46519032881566E-32,
1.));
#23334=DIRECTION('center_axis',(0.,-1.,-2.46519032881566E-32));
#23335=DIRECTION('ref_axis',(1.,0.,0.));
#23336=DIRECTION('center_axis',(0.,-1.,-2.46519032881566E-32));
#23337=DIRECTION('ref_axis',(1.,0.,0.));
#23338=DIRECTION('',(1.22460635382238E-16,1.,2.46519032881566E-32));
#23339=DIRECTION('center_axis',(0.,-1.,-2.46519032881566E-32));
#23340=DIRECTION('ref_axis',(1.,0.,0.));
#23341=DIRECTION('center_axis',(0.,-1.,-2.46519032881566E-32));
#23342=DIRECTION('ref_axis',(1.,0.,0.));
#23343=DIRECTION('center_axis',(0.,-1.,-2.46519032881566E-32));
#23344=DIRECTION('ref_axis',(1.,0.,0.));
#23345=DIRECTION('',(0.81915204428899,0.573576436351049,1.00317192905352E-16));
#23346=DIRECTION('center_axis',(0.,-1.,-2.46519032881566E-32));
#23347=DIRECTION('ref_axis',(1.,0.,0.));
#23348=DIRECTION('center_axis',(0.,-1.,-2.46519032881566E-32));
#23349=DIRECTION('ref_axis',(1.,0.,0.));
#23350=DIRECTION('center_axis',(0.,1.,2.46519032881566E-32));
#23351=DIRECTION('ref_axis',(-1.,0.,0.));
#23352=DIRECTION('',(-0.819152044288993,-0.573576436351044,1.00317192905353E-16));
#23353=DIRECTION('center_axis',(-1.22460635382238E-16,-1.,-2.46519032881566E-32));
#23354=DIRECTION('ref_axis',(-3.01888774004913E-48,-2.46519032881566E-32,
1.));
#23355=DIRECTION('center_axis',(0.,-1.,-2.46519032881566E-32));
#23356=DIRECTION('ref_axis',(1.,0.,0.));
#23357=DIRECTION('center_axis',(0.,-1.,-2.46519032881566E-32));
#23358=DIRECTION('ref_axis',(1.,0.,0.));
#23359=DIRECTION('',(1.22460635382238E-16,1.,2.46519032881566E-32));
#23360=DIRECTION('center_axis',(0.,-1.,-2.46519032881566E-32));
#23361=DIRECTION('ref_axis',(1.,0.,0.));
#23362=DIRECTION('center_axis',(0.,-1.,-2.46519032881566E-32));
#23363=DIRECTION('ref_axis',(1.,0.,0.));
#23364=DIRECTION('center_axis',(0.,-1.,-2.46519032881566E-32));
#23365=DIRECTION('ref_axis',(1.,0.,0.));
#23366=DIRECTION('',(0.81915204428899,0.573576436351049,1.00317192905352E-16));
#23367=DIRECTION('center_axis',(0.,-1.,-2.46519032881566E-32));
#23368=DIRECTION('ref_axis',(1.,0.,0.));
#23369=DIRECTION('center_axis',(0.,-1.,-2.46519032881566E-32));
#23370=DIRECTION('ref_axis',(1.,0.,0.));
#23371=DIRECTION('center_axis',(0.,1.,2.46519032881566E-32));
#23372=DIRECTION('ref_axis',(-1.,0.,0.));
#23373=DIRECTION('',(-0.819152044288993,-0.573576436351044,1.00317192905353E-16));
#23374=DIRECTION('center_axis',(-1.22460635382238E-16,-1.,-2.46519032881566E-32));
#23375=DIRECTION('ref_axis',(-3.01888774004913E-48,-2.46519032881566E-32,
1.));
#23376=DIRECTION('center_axis',(0.,-1.,-2.46519032881566E-32));
#23377=DIRECTION('ref_axis',(1.,0.,0.));
#23378=DIRECTION('center_axis',(0.,-1.,-2.46519032881566E-32));
#23379=DIRECTION('ref_axis',(1.,0.,0.));
#23380=DIRECTION('',(1.22460635382238E-16,1.,2.46519032881566E-32));
#23381=DIRECTION('center_axis',(0.,-1.,-2.46519032881566E-32));
#23382=DIRECTION('ref_axis',(1.,0.,0.));
#23383=DIRECTION('center_axis',(0.,-1.,-2.46519032881566E-32));
#23384=DIRECTION('ref_axis',(1.,0.,0.));
#23385=DIRECTION('center_axis',(0.,-1.,-2.46519032881566E-32));
#23386=DIRECTION('ref_axis',(1.,0.,0.));
#23387=DIRECTION('',(0.81915204428899,0.573576436351049,1.00317192905352E-16));
#23388=DIRECTION('center_axis',(0.,-1.,-2.46519032881566E-32));
#23389=DIRECTION('ref_axis',(1.,0.,0.));
#23390=DIRECTION('center_axis',(0.,-1.,-2.46519032881566E-32));
#23391=DIRECTION('ref_axis',(1.,0.,0.));
#23392=DIRECTION('center_axis',(0.,1.,2.46519032881566E-32));
#23393=DIRECTION('ref_axis',(-1.,0.,0.));
#23394=DIRECTION('',(-0.819152044288993,-0.573576436351044,1.00317192905353E-16));
#23395=DIRECTION('center_axis',(-1.22460635382238E-16,-1.,-2.46519032881566E-32));
#23396=DIRECTION('ref_axis',(-3.01888774004913E-48,-2.46519032881566E-32,
1.));
#23397=DIRECTION('center_axis',(0.,-1.,-2.46519032881566E-32));
#23398=DIRECTION('ref_axis',(1.,0.,0.));
#23399=DIRECTION('center_axis',(0.,-1.,-2.46519032881566E-32));
#23400=DIRECTION('ref_axis',(1.,0.,0.));
#23401=DIRECTION('',(1.22460635382238E-16,1.,2.46519032881566E-32));
#23402=DIRECTION('center_axis',(0.,-1.,-2.46519032881566E-32));
#23403=DIRECTION('ref_axis',(1.,0.,0.));
#23404=DIRECTION('center_axis',(0.,-1.,-2.46519032881566E-32));
#23405=DIRECTION('ref_axis',(1.,0.,0.));
#23406=DIRECTION('center_axis',(0.,-1.,-2.46519032881566E-32));
#23407=DIRECTION('ref_axis',(1.,0.,0.));
#23408=DIRECTION('',(0.81915204428899,0.573576436351049,1.00317192905352E-16));
#23409=DIRECTION('center_axis',(0.,-1.,-2.46519032881566E-32));
#23410=DIRECTION('ref_axis',(1.,0.,0.));
#23411=DIRECTION('center_axis',(0.,-1.,-2.46519032881566E-32));
#23412=DIRECTION('ref_axis',(1.,0.,0.));
#23413=DIRECTION('center_axis',(0.,1.,2.46519032881566E-32));
#23414=DIRECTION('ref_axis',(-1.,0.,0.));
#23415=DIRECTION('',(-0.819152044288993,-0.573576436351044,1.00317192905353E-16));
#23416=DIRECTION('center_axis',(-1.22460635382238E-16,-1.,-2.46519032881566E-32));
#23417=DIRECTION('ref_axis',(-3.01888774004913E-48,-2.46519032881566E-32,
1.));
#23418=DIRECTION('center_axis',(0.,-1.,-2.46519032881566E-32));
#23419=DIRECTION('ref_axis',(1.,0.,0.));
#23420=DIRECTION('center_axis',(0.,-1.,-2.46519032881566E-32));
#23421=DIRECTION('ref_axis',(1.,0.,0.));
#23422=DIRECTION('',(1.22460635382238E-16,1.,2.46519032881566E-32));
#23423=DIRECTION('center_axis',(0.,-1.,-2.46519032881566E-32));
#23424=DIRECTION('ref_axis',(1.,0.,0.));
#23425=DIRECTION('center_axis',(0.,-1.,-2.46519032881566E-32));
#23426=DIRECTION('ref_axis',(1.,0.,0.));
#23427=DIRECTION('center_axis',(0.,-1.,-2.46519032881566E-32));
#23428=DIRECTION('ref_axis',(1.,0.,0.));
#23429=DIRECTION('',(0.81915204428899,0.573576436351049,1.00317192905352E-16));
#23430=DIRECTION('center_axis',(0.,-1.,-2.46519032881566E-32));
#23431=DIRECTION('ref_axis',(1.,0.,0.));
#23432=DIRECTION('center_axis',(0.,-1.,-2.46519032881566E-32));
#23433=DIRECTION('ref_axis',(1.,0.,0.));
#23434=DIRECTION('center_axis',(0.,1.,2.46519032881566E-32));
#23435=DIRECTION('ref_axis',(-1.,0.,0.));
#23436=DIRECTION('',(-0.819152044288993,-0.573576436351044,1.00317192905353E-16));
#23437=DIRECTION('center_axis',(-1.22460635382238E-16,-1.,-2.46519032881566E-32));
#23438=DIRECTION('ref_axis',(-3.01888774004913E-48,-2.46519032881566E-32,
1.));
#23439=DIRECTION('center_axis',(0.,-1.,-2.46519032881566E-32));
#23440=DIRECTION('ref_axis',(1.,0.,0.));
#23441=DIRECTION('center_axis',(0.,-1.,-2.46519032881566E-32));
#23442=DIRECTION('ref_axis',(1.,0.,0.));
#23443=DIRECTION('',(1.22460635382238E-16,1.,2.46519032881566E-32));
#23444=DIRECTION('center_axis',(0.,-1.,-2.46519032881566E-32));
#23445=DIRECTION('ref_axis',(1.,0.,0.));
#23446=DIRECTION('center_axis',(0.,-1.,-2.46519032881566E-32));
#23447=DIRECTION('ref_axis',(1.,0.,0.));
#23448=DIRECTION('center_axis',(0.,-1.,-2.46519032881566E-32));
#23449=DIRECTION('ref_axis',(1.,0.,0.));
#23450=DIRECTION('',(0.81915204428899,0.573576436351049,1.00317192905352E-16));
#23451=DIRECTION('center_axis',(0.,-1.,-2.46519032881566E-32));
#23452=DIRECTION('ref_axis',(1.,0.,0.));
#23453=DIRECTION('center_axis',(0.,-1.,-2.46519032881566E-32));
#23454=DIRECTION('ref_axis',(1.,0.,0.));
#23455=DIRECTION('center_axis',(0.,1.,2.46519032881566E-32));
#23456=DIRECTION('ref_axis',(-1.,0.,0.));
#23457=DIRECTION('',(-0.819152044288993,-0.573576436351044,1.00317192905353E-16));
#23458=DIRECTION('center_axis',(-1.22460635382238E-16,-1.,-2.46519032881566E-32));
#23459=DIRECTION('ref_axis',(-3.01888774004913E-48,-2.46519032881566E-32,
1.));
#23460=DIRECTION('center_axis',(0.,-1.,-2.46519032881566E-32));
#23461=DIRECTION('ref_axis',(1.,0.,0.));
#23462=DIRECTION('center_axis',(0.,-1.,-2.46519032881566E-32));
#23463=DIRECTION('ref_axis',(1.,0.,0.));
#23464=DIRECTION('',(1.22460635382238E-16,1.,2.46519032881566E-32));
#23465=DIRECTION('center_axis',(0.,-1.,-2.46519032881566E-32));
#23466=DIRECTION('ref_axis',(1.,0.,0.));
#23467=DIRECTION('center_axis',(0.,-1.,-2.46519032881566E-32));
#23468=DIRECTION('ref_axis',(1.,0.,0.));
#23469=DIRECTION('center_axis',(0.,-1.,-2.46519032881566E-32));
#23470=DIRECTION('ref_axis',(1.,0.,0.));
#23471=DIRECTION('',(0.81915204428899,0.573576436351049,1.00317192905352E-16));
#23472=DIRECTION('center_axis',(0.,-1.,-2.46519032881566E-32));
#23473=DIRECTION('ref_axis',(1.,0.,0.));
#23474=DIRECTION('center_axis',(0.,-1.,-2.46519032881566E-32));
#23475=DIRECTION('ref_axis',(1.,0.,0.));
#23476=DIRECTION('center_axis',(0.,1.,2.46519032881566E-32));
#23477=DIRECTION('ref_axis',(-1.,0.,0.));
#23478=DIRECTION('',(-0.819152044288993,-0.573576436351044,1.00317192905353E-16));
#23479=DIRECTION('center_axis',(-1.22460635382238E-16,-1.,-2.46519032881566E-32));
#23480=DIRECTION('ref_axis',(-3.01888774004913E-48,-2.46519032881566E-32,
1.));
#23481=DIRECTION('center_axis',(0.,-1.,-2.46519032881566E-32));
#23482=DIRECTION('ref_axis',(1.,0.,0.));
#23483=DIRECTION('center_axis',(0.,-1.,-2.46519032881566E-32));
#23484=DIRECTION('ref_axis',(1.,0.,0.));
#23485=DIRECTION('',(1.22460635382238E-16,1.,2.46519032881566E-32));
#23486=DIRECTION('center_axis',(0.,-1.,-2.46519032881566E-32));
#23487=DIRECTION('ref_axis',(1.,0.,0.));
#23488=DIRECTION('center_axis',(0.,-1.,-2.46519032881566E-32));
#23489=DIRECTION('ref_axis',(1.,0.,0.));
#23490=DIRECTION('center_axis',(0.,-1.,-2.46519032881566E-32));
#23491=DIRECTION('ref_axis',(1.,0.,0.));
#23492=DIRECTION('',(0.81915204428899,0.573576436351049,1.00317192905352E-16));
#23493=DIRECTION('center_axis',(0.,-1.,-2.46519032881566E-32));
#23494=DIRECTION('ref_axis',(1.,0.,0.));
#23495=DIRECTION('center_axis',(0.,-1.,-2.46519032881566E-32));
#23496=DIRECTION('ref_axis',(1.,0.,0.));
#23497=DIRECTION('center_axis',(0.,1.,2.46519032881566E-32));
#23498=DIRECTION('ref_axis',(-1.,0.,0.));
#23499=DIRECTION('',(-0.819152044288993,-0.573576436351044,1.00317192905353E-16));
#23500=DIRECTION('center_axis',(-1.22460635382238E-16,-1.,-2.46519032881566E-32));
#23501=DIRECTION('ref_axis',(-3.01888774004913E-48,-2.46519032881566E-32,
1.));
#23502=DIRECTION('center_axis',(0.,-1.,-2.46519032881566E-32));
#23503=DIRECTION('ref_axis',(1.,0.,0.));
#23504=DIRECTION('center_axis',(0.,-1.,-2.46519032881566E-32));
#23505=DIRECTION('ref_axis',(1.,0.,0.));
#23506=DIRECTION('',(1.22460635382238E-16,1.,2.46519032881566E-32));
#23507=DIRECTION('center_axis',(0.,-1.,-2.46519032881566E-32));
#23508=DIRECTION('ref_axis',(1.,0.,0.));
#23509=DIRECTION('center_axis',(0.,-1.,-2.46519032881566E-32));
#23510=DIRECTION('ref_axis',(1.,0.,0.));
#23511=DIRECTION('center_axis',(0.,-1.,-2.46519032881566E-32));
#23512=DIRECTION('ref_axis',(1.,0.,0.));
#23513=DIRECTION('',(0.81915204428899,0.573576436351049,1.00317192905352E-16));
#23514=DIRECTION('center_axis',(0.,-1.,-2.46519032881566E-32));
#23515=DIRECTION('ref_axis',(1.,0.,0.));
#23516=DIRECTION('center_axis',(0.,-1.,-2.46519032881566E-32));
#23517=DIRECTION('ref_axis',(1.,0.,0.));
#23518=DIRECTION('center_axis',(0.,1.,2.46519032881566E-32));
#23519=DIRECTION('ref_axis',(-1.,0.,0.));
#23520=DIRECTION('',(-0.819152044288993,-0.573576436351044,1.00317192905353E-16));
#23521=DIRECTION('center_axis',(-1.22460635382238E-16,-1.,-2.46519032881566E-32));
#23522=DIRECTION('ref_axis',(-3.01888774004913E-48,-2.46519032881566E-32,
1.));
#23523=DIRECTION('center_axis',(0.,-1.,-2.46519032881566E-32));
#23524=DIRECTION('ref_axis',(1.,0.,0.));
#23525=DIRECTION('center_axis',(0.,-1.,-2.46519032881566E-32));
#23526=DIRECTION('ref_axis',(1.,0.,0.));
#23527=DIRECTION('',(1.22460635382238E-16,1.,2.46519032881566E-32));
#23528=DIRECTION('center_axis',(0.,-1.,-2.46519032881566E-32));
#23529=DIRECTION('ref_axis',(1.,0.,0.));
#23530=DIRECTION('center_axis',(0.,-1.,-2.46519032881566E-32));
#23531=DIRECTION('ref_axis',(1.,0.,0.));
#23532=DIRECTION('center_axis',(0.,-1.,-2.46519032881566E-32));
#23533=DIRECTION('ref_axis',(1.,0.,0.));
#23534=DIRECTION('',(0.81915204428899,0.573576436351049,1.00317192905352E-16));
#23535=DIRECTION('center_axis',(0.,-1.,-2.46519032881566E-32));
#23536=DIRECTION('ref_axis',(1.,0.,0.));
#23537=DIRECTION('center_axis',(0.,-1.,-2.46519032881566E-32));
#23538=DIRECTION('ref_axis',(1.,0.,0.));
#23539=DIRECTION('center_axis',(0.,1.,2.46519032881566E-32));
#23540=DIRECTION('ref_axis',(-1.,0.,0.));
#23541=DIRECTION('',(-0.819152044288993,-0.573576436351044,1.00317192905353E-16));
#23542=DIRECTION('center_axis',(-1.22460635382238E-16,-1.,-2.46519032881566E-32));
#23543=DIRECTION('ref_axis',(-3.01888774004913E-48,-2.46519032881566E-32,
1.));
#23544=DIRECTION('',(1.22460635382238E-16,1.,2.46519032881566E-32));
#23545=DIRECTION('center_axis',(-1.22460635382238E-16,-1.,-2.46519032881566E-32));
#23546=DIRECTION('ref_axis',(-3.01888774004913E-48,-2.46519032881566E-32,
1.));
#23547=DIRECTION('center_axis',(-1.22460635382238E-16,-1.,-2.46519032881566E-32));
#23548=DIRECTION('ref_axis',(-3.01888774004913E-48,-2.46519032881566E-32,
1.));
#23549=DIRECTION('center_axis',(-1.22460635382238E-16,-1.,-2.46519032881566E-32));
#23550=DIRECTION('ref_axis',(-3.01888774004913E-48,-2.46519032881566E-32,
1.));
#23551=DIRECTION('center_axis',(-1.22460635382238E-16,-1.,-2.46519032881566E-32));
#23552=DIRECTION('ref_axis',(-3.01888774004913E-48,-2.46519032881566E-32,
1.));
#23553=DIRECTION('center_axis',(-1.22460635382238E-16,-1.,-2.46519032881566E-32));
#23554=DIRECTION('ref_axis',(-3.01888774004913E-48,-2.46519032881566E-32,
1.));
#23555=DIRECTION('center_axis',(-1.22460635382238E-16,-1.,-2.46519032881566E-32));
#23556=DIRECTION('ref_axis',(-3.01888774004913E-48,-2.46519032881566E-32,
1.));
#23557=DIRECTION('center_axis',(-1.22460635382238E-16,-1.,-2.46519032881566E-32));
#23558=DIRECTION('ref_axis',(-3.01888774004913E-48,-2.46519032881566E-32,
1.));
#23559=DIRECTION('center_axis',(-1.22460635382238E-16,-1.,-2.46519032881566E-32));
#23560=DIRECTION('ref_axis',(-3.01888774004913E-48,-2.46519032881566E-32,
1.));
#23561=DIRECTION('center_axis',(-1.22460635382238E-16,-1.,-2.46519032881566E-32));
#23562=DIRECTION('ref_axis',(-3.01888774004913E-48,-2.46519032881566E-32,
1.));
#23563=DIRECTION('center_axis',(-1.22460635382238E-16,-1.,-2.46519032881566E-32));
#23564=DIRECTION('ref_axis',(-3.01888774004913E-48,-2.46519032881566E-32,
1.));
#23565=DIRECTION('center_axis',(-1.22460635382238E-16,-1.,-2.46519032881566E-32));
#23566=DIRECTION('ref_axis',(-3.01888774004913E-48,-2.46519032881566E-32,
1.));
#23567=DIRECTION('center_axis',(-1.22460635382238E-16,-1.,-2.46519032881566E-32));
#23568=DIRECTION('ref_axis',(-3.01888774004913E-48,-2.46519032881566E-32,
1.));
#23569=DIRECTION('center_axis',(-1.22460635382238E-16,-1.,-2.46519032881566E-32));
#23570=DIRECTION('ref_axis',(-3.01888774004913E-48,-2.46519032881566E-32,
1.));
#23571=DIRECTION('center_axis',(-1.22460635382238E-16,-1.,-2.46519032881566E-32));
#23572=DIRECTION('ref_axis',(-3.01888774004913E-48,-2.46519032881566E-32,
1.));
#23573=DIRECTION('center_axis',(-1.22460635382238E-16,-1.,-2.46519032881566E-32));
#23574=DIRECTION('ref_axis',(-3.01888774004913E-48,-2.46519032881566E-32,
1.));
#23575=DIRECTION('center_axis',(-1.22460635382238E-16,-1.,-2.46519032881566E-32));
#23576=DIRECTION('ref_axis',(-3.01888774004913E-48,-2.46519032881566E-32,
1.));
#23577=DIRECTION('center_axis',(-1.22460635382238E-16,-1.,-2.46519032881566E-32));
#23578=DIRECTION('ref_axis',(-3.01888774004913E-48,-2.46519032881566E-32,
1.));
#23579=DIRECTION('center_axis',(-1.22460635382238E-16,-1.,-2.46519032881566E-32));
#23580=DIRECTION('ref_axis',(-3.01888774004913E-48,-2.46519032881566E-32,
1.));
#23581=DIRECTION('center_axis',(-1.22460635382238E-16,-1.,-2.46519032881566E-32));
#23582=DIRECTION('ref_axis',(-3.01888774004913E-48,-2.46519032881566E-32,
1.));
#23583=DIRECTION('center_axis',(-1.22460635382238E-16,-1.,-2.46519032881566E-32));
#23584=DIRECTION('ref_axis',(-3.01888774004913E-48,-2.46519032881566E-32,
1.));
#23585=DIRECTION('center_axis',(-1.22460635382238E-16,-1.,-2.46519032881566E-32));
#23586=DIRECTION('ref_axis',(-3.01888774004913E-48,-2.46519032881566E-32,
1.));
#23587=DIRECTION('center_axis',(-1.22460635382238E-16,-1.,-2.46519032881566E-32));
#23588=DIRECTION('ref_axis',(-3.01888774004913E-48,-2.46519032881566E-32,
1.));
#23589=DIRECTION('center_axis',(-1.22460635382238E-16,-1.,-2.46519032881566E-32));
#23590=DIRECTION('ref_axis',(-3.01888774004913E-48,-2.46519032881566E-32,
1.));
#23591=DIRECTION('center_axis',(-1.22460635382238E-16,-1.,-2.46519032881566E-32));
#23592=DIRECTION('ref_axis',(-3.01888774004913E-48,-2.46519032881566E-32,
1.));
#23593=DIRECTION('center_axis',(-1.22460635382238E-16,-1.,-2.46519032881566E-32));
#23594=DIRECTION('ref_axis',(-3.01888774004913E-48,-2.46519032881566E-32,
1.));
#23595=DIRECTION('center_axis',(-1.22460635382238E-16,-1.,-2.46519032881566E-32));
#23596=DIRECTION('ref_axis',(-3.01888774004913E-48,-2.46519032881566E-32,
1.));
#23597=DIRECTION('center_axis',(-1.22460635382238E-16,-1.,-2.46519032881566E-32));
#23598=DIRECTION('ref_axis',(-3.01888774004913E-48,-2.46519032881566E-32,
1.));
#23599=DIRECTION('center_axis',(-1.22460635382238E-16,-1.,-2.46519032881566E-32));
#23600=DIRECTION('ref_axis',(-3.01888774004913E-48,-2.46519032881566E-32,
1.));
#23601=DIRECTION('center_axis',(-1.22460635382238E-16,-1.,-2.46519032881566E-32));
#23602=DIRECTION('ref_axis',(-3.01888774004913E-48,-2.46519032881566E-32,
1.));
#23603=DIRECTION('center_axis',(-1.22460635382238E-16,-1.,-2.46519032881566E-32));
#23604=DIRECTION('ref_axis',(-3.01888774004913E-48,-2.46519032881566E-32,
1.));
#23605=DIRECTION('center_axis',(-1.22460635382238E-16,-1.,-2.46519032881566E-32));
#23606=DIRECTION('ref_axis',(-3.01888774004913E-48,-2.46519032881566E-32,
1.));
#23607=DIRECTION('center_axis',(-1.22460635382238E-16,-1.,-2.46519032881566E-32));
#23608=DIRECTION('ref_axis',(-3.01888774004913E-48,-2.46519032881566E-32,
1.));
#23609=DIRECTION('center_axis',(-1.22460635382238E-16,-1.,-2.46519032881566E-32));
#23610=DIRECTION('ref_axis',(-3.01888774004913E-48,-2.46519032881566E-32,
1.));
#23611=DIRECTION('center_axis',(-1.22460635382238E-16,-1.,-2.46519032881566E-32));
#23612=DIRECTION('ref_axis',(-3.01888774004913E-48,-2.46519032881566E-32,
1.));
#23613=DIRECTION('center_axis',(-1.22460635382238E-16,-1.,-2.46519032881566E-32));
#23614=DIRECTION('ref_axis',(-3.01888774004913E-48,-2.46519032881566E-32,
1.));
#23615=DIRECTION('center_axis',(-1.22460635382238E-16,-1.,-2.46519032881566E-32));
#23616=DIRECTION('ref_axis',(-3.01888774004913E-48,-2.46519032881566E-32,
1.));
#23617=DIRECTION('center_axis',(-1.22460635382238E-16,-1.,-2.46519032881566E-32));
#23618=DIRECTION('ref_axis',(-3.01888774004913E-48,-2.46519032881566E-32,
1.));
#23619=DIRECTION('center_axis',(-1.22460635382238E-16,-1.,-2.46519032881566E-32));
#23620=DIRECTION('ref_axis',(-3.01888774004913E-48,-2.46519032881566E-32,
1.));
#23621=DIRECTION('center_axis',(-1.22460635382238E-16,-1.,-2.46519032881566E-32));
#23622=DIRECTION('ref_axis',(-3.01888774004913E-48,-2.46519032881566E-32,
1.));
#23623=DIRECTION('center_axis',(-1.22460635382238E-16,-1.,-2.46519032881566E-32));
#23624=DIRECTION('ref_axis',(-3.01888774004913E-48,-2.46519032881566E-32,
1.));
#23625=DIRECTION('center_axis',(-1.22460635382238E-16,-1.,-2.46519032881566E-32));
#23626=DIRECTION('ref_axis',(-3.01888774004913E-48,-2.46519032881566E-32,
1.));
#23627=DIRECTION('',(-2.85991635595236E-21,0.707106781186547,0.707106781186548));
#23628=DIRECTION('center_axis',(-1.22460635382238E-16,-1.,-2.46519032881566E-32));
#23629=DIRECTION('ref_axis',(-3.01888774004913E-48,-2.46519032881566E-32,
1.));
#23630=DIRECTION('center_axis',(-1.22460635382238E-16,-1.,-2.46519032881566E-32));
#23631=DIRECTION('ref_axis',(-3.01888774004913E-48,-2.46519032881566E-32,
1.));
#23632=DIRECTION('center_axis',(-1.22460635382238E-16,-1.,-2.46519032881566E-32));
#23633=DIRECTION('ref_axis',(-3.01888774004913E-48,-2.46519032881566E-32,
1.));
#23634=DIRECTION('center_axis',(-1.22460635382238E-16,-1.,-2.46519032881566E-32));
#23635=DIRECTION('ref_axis',(-3.01888774004913E-48,-2.46519032881566E-32,
1.));
#23636=DIRECTION('center_axis',(-1.22460635382238E-16,-1.,-2.46519032881566E-32));
#23637=DIRECTION('ref_axis',(-3.01888774004913E-48,-2.46519032881566E-32,
1.));
#23638=DIRECTION('center_axis',(-1.22460635382238E-16,-1.,-2.46519032881566E-32));
#23639=DIRECTION('ref_axis',(-3.01888774004913E-48,-2.46519032881566E-32,
1.));
#23640=DIRECTION('center_axis',(-1.22460635382238E-16,-1.,-2.46519032881566E-32));
#23641=DIRECTION('ref_axis',(-3.01888774004913E-48,-2.46519032881566E-32,
1.));
#23642=DIRECTION('center_axis',(-1.22460635382238E-16,-1.,-2.46519032881566E-32));
#23643=DIRECTION('ref_axis',(-3.01888774004913E-48,-2.46519032881566E-32,
1.));
#23644=DIRECTION('center_axis',(-1.22460635382238E-16,-1.,-2.46519032881566E-32));
#23645=DIRECTION('ref_axis',(-3.01888774004913E-48,-2.46519032881566E-32,
1.));
#23646=DIRECTION('center_axis',(-1.22460635382238E-16,-1.,-2.46519032881566E-32));
#23647=DIRECTION('ref_axis',(-3.01888774004913E-48,-2.46519032881566E-32,
1.));
#23648=DIRECTION('center_axis',(-1.22460635382238E-16,-1.,-2.46519032881566E-32));
#23649=DIRECTION('ref_axis',(-3.01888774004913E-48,-2.46519032881566E-32,
1.));
#23650=DIRECTION('center_axis',(-1.22460635382238E-16,-1.,-2.46519032881566E-32));
#23651=DIRECTION('ref_axis',(-3.01888774004913E-48,-2.46519032881566E-32,
1.));
#23652=DIRECTION('center_axis',(-1.22460635382238E-16,-1.,-2.46519032881566E-32));
#23653=DIRECTION('ref_axis',(-3.01888774004913E-48,-2.46519032881566E-32,
1.));
#23654=DIRECTION('center_axis',(-1.22460635382238E-16,-1.,-2.46519032881566E-32));
#23655=DIRECTION('ref_axis',(-3.01888774004913E-48,-2.46519032881566E-32,
1.));
#23656=DIRECTION('center_axis',(-1.22460635382238E-16,-1.,-2.46519032881566E-32));
#23657=DIRECTION('ref_axis',(-3.01888774004913E-48,-2.46519032881566E-32,
1.));
#23658=DIRECTION('center_axis',(-1.22460635382238E-16,-1.,-2.46519032881566E-32));
#23659=DIRECTION('ref_axis',(-3.01888774004913E-48,-2.46519032881566E-32,
1.));
#23660=DIRECTION('center_axis',(-1.22460635382238E-16,-1.,-2.46519032881566E-32));
#23661=DIRECTION('ref_axis',(-3.01888774004913E-48,-2.46519032881566E-32,
1.));
#23662=DIRECTION('center_axis',(-1.22460635382238E-16,-1.,-2.46519032881566E-32));
#23663=DIRECTION('ref_axis',(-3.01888774004913E-48,-2.46519032881566E-32,
1.));
#23664=DIRECTION('center_axis',(-1.22460635382238E-16,-1.,-2.46519032881566E-32));
#23665=DIRECTION('ref_axis',(-3.01888774004913E-48,-2.46519032881566E-32,
1.));
#23666=DIRECTION('center_axis',(-1.22460635382238E-16,-1.,-2.46519032881566E-32));
#23667=DIRECTION('ref_axis',(-3.01888774004913E-48,-2.46519032881566E-32,
1.));
#23668=DIRECTION('center_axis',(-1.22460635382238E-16,-1.,-2.46519032881566E-32));
#23669=DIRECTION('ref_axis',(-3.01888774004913E-48,-2.46519032881566E-32,
1.));
#23670=DIRECTION('center_axis',(-1.22460635382238E-16,-1.,-2.46519032881566E-32));
#23671=DIRECTION('ref_axis',(-3.01888774004913E-48,-2.46519032881566E-32,
1.));
#23672=DIRECTION('center_axis',(-1.22460635382238E-16,-1.,-2.46519032881566E-32));
#23673=DIRECTION('ref_axis',(-3.01888774004913E-48,-2.46519032881566E-32,
1.));
#23674=DIRECTION('center_axis',(-1.22460635382238E-16,-1.,-2.46519032881566E-32));
#23675=DIRECTION('ref_axis',(-3.01888774004913E-48,-2.46519032881566E-32,
1.));
#23676=DIRECTION('center_axis',(-1.22460635382238E-16,-1.,-2.46519032881566E-32));
#23677=DIRECTION('ref_axis',(-3.01888774004913E-48,-2.46519032881566E-32,
1.));
#23678=DIRECTION('center_axis',(-1.22460635382238E-16,-1.,-2.46519032881566E-32));
#23679=DIRECTION('ref_axis',(-3.01888774004913E-48,-2.46519032881566E-32,
1.));
#23680=DIRECTION('center_axis',(-1.22460635382238E-16,-1.,-2.46519032881566E-32));
#23681=DIRECTION('ref_axis',(-3.01888774004913E-48,-2.46519032881566E-32,
1.));
#23682=DIRECTION('center_axis',(-1.22460635382238E-16,-1.,-2.46519032881566E-32));
#23683=DIRECTION('ref_axis',(-3.01888774004913E-48,-2.46519032881566E-32,
1.));
#23684=DIRECTION('center_axis',(-1.22460635382238E-16,-1.,-2.46519032881566E-32));
#23685=DIRECTION('ref_axis',(-3.01888774004913E-48,-2.46519032881566E-32,
1.));
#23686=DIRECTION('center_axis',(-1.22460635382238E-16,-1.,-2.46519032881566E-32));
#23687=DIRECTION('ref_axis',(-3.01888774004913E-48,-2.46519032881566E-32,
1.));
#23688=DIRECTION('center_axis',(-1.22460635382238E-16,-1.,-2.46519032881566E-32));
#23689=DIRECTION('ref_axis',(-3.01888774004913E-48,-2.46519032881566E-32,
1.));
#23690=DIRECTION('center_axis',(-1.22460635382238E-16,-1.,-2.46519032881566E-32));
#23691=DIRECTION('ref_axis',(-3.01888774004913E-48,-2.46519032881566E-32,
1.));
#23692=DIRECTION('center_axis',(-1.22460635382238E-16,-1.,-2.46519032881566E-32));
#23693=DIRECTION('ref_axis',(-3.01888774004913E-48,-2.46519032881566E-32,
1.));
#23694=DIRECTION('center_axis',(-1.22460635382238E-16,-1.,-2.46519032881566E-32));
#23695=DIRECTION('ref_axis',(-3.01888774004913E-48,-2.46519032881566E-32,
1.));
#23696=DIRECTION('center_axis',(-1.22460635382238E-16,-1.,-2.46519032881566E-32));
#23697=DIRECTION('ref_axis',(-3.01888774004913E-48,-2.46519032881566E-32,
1.));
#23698=DIRECTION('center_axis',(-1.22460635382238E-16,-1.,-2.46519032881566E-32));
#23699=DIRECTION('ref_axis',(-3.01888774004913E-48,-2.46519032881566E-32,
1.));
#23700=DIRECTION('center_axis',(-1.22460635382238E-16,-1.,-2.46519032881566E-32));
#23701=DIRECTION('ref_axis',(-3.01888774004913E-48,-2.46519032881566E-32,
1.));
#23702=DIRECTION('center_axis',(-1.22460635382238E-16,-1.,-2.46519032881566E-32));
#23703=DIRECTION('ref_axis',(-3.01888774004913E-48,-2.46519032881566E-32,
1.));
#23704=DIRECTION('center_axis',(-1.22460635382238E-16,-1.,-2.46519032881566E-32));
#23705=DIRECTION('ref_axis',(-3.01888774004913E-48,-2.46519032881566E-32,
1.));
#23706=DIRECTION('center_axis',(1.22460635382238E-16,1.,2.46519032881566E-32));
#23707=DIRECTION('ref_axis',(3.01888774004913E-48,2.46519032881566E-32,
-1.));
#23708=DIRECTION('center_axis',(-1.22460635382238E-16,-1.,-2.46519032881566E-32));
#23709=DIRECTION('ref_axis',(-3.01888774004913E-48,-2.46519032881566E-32,
1.));
#23710=DIRECTION('center_axis',(-1.22460635382238E-16,-1.,-2.46519032881566E-32));
#23711=DIRECTION('ref_axis',(-3.01888774004913E-48,-2.46519032881566E-32,
1.));
#23712=DIRECTION('center_axis',(-1.22460635382238E-16,-1.,-2.46519032881566E-32));
#23713=DIRECTION('ref_axis',(-3.01888774004913E-48,-2.46519032881566E-32,
1.));
#23714=DIRECTION('center_axis',(-1.22460635382238E-16,-1.,-2.46519032881566E-32));
#23715=DIRECTION('ref_axis',(-3.01888774004913E-48,-2.46519032881566E-32,
1.));
#23716=DIRECTION('center_axis',(-1.22460635382238E-16,-1.,-2.46519032881566E-32));
#23717=DIRECTION('ref_axis',(-3.01888774004913E-48,-2.46519032881566E-32,
1.));
#23718=DIRECTION('center_axis',(-1.22460635382238E-16,-1.,-2.46519032881566E-32));
#23719=DIRECTION('ref_axis',(-3.01888774004913E-48,-2.46519032881566E-32,
1.));
#23720=DIRECTION('center_axis',(-1.22460635382238E-16,-1.,-2.46519032881566E-32));
#23721=DIRECTION('ref_axis',(-3.01888774004913E-48,-2.46519032881566E-32,
1.));
#23722=DIRECTION('center_axis',(-1.22460635382238E-16,-1.,-2.46519032881566E-32));
#23723=DIRECTION('ref_axis',(-3.01888774004913E-48,-2.46519032881566E-32,
1.));
#23724=DIRECTION('center_axis',(-1.22460635382238E-16,-1.,-2.46519032881566E-32));
#23725=DIRECTION('ref_axis',(-3.01888774004913E-48,-2.46519032881566E-32,
1.));
#23726=DIRECTION('center_axis',(-1.22460635382238E-16,-1.,-2.46519032881566E-32));
#23727=DIRECTION('ref_axis',(-3.01888774004913E-48,-2.46519032881566E-32,
1.));
#23728=DIRECTION('center_axis',(-1.22460635382238E-16,-1.,-2.46519032881566E-32));
#23729=DIRECTION('ref_axis',(-3.01888774004913E-48,-2.46519032881566E-32,
1.));
#23730=DIRECTION('center_axis',(-1.22460635382238E-16,-1.,-2.46519032881566E-32));
#23731=DIRECTION('ref_axis',(-3.01888774004913E-48,-2.46519032881566E-32,
1.));
#23732=DIRECTION('center_axis',(-1.22460635382238E-16,-1.,-2.46519032881566E-32));
#23733=DIRECTION('ref_axis',(-3.01888774004913E-48,-2.46519032881566E-32,
1.));
#23734=DIRECTION('center_axis',(-1.22460635382238E-16,-1.,-2.46519032881566E-32));
#23735=DIRECTION('ref_axis',(-3.01888774004913E-48,-2.46519032881566E-32,
1.));
#23736=DIRECTION('center_axis',(-1.22460635382238E-16,-1.,-2.46519032881566E-32));
#23737=DIRECTION('ref_axis',(-3.01888774004913E-48,-2.46519032881566E-32,
1.));
#23738=DIRECTION('center_axis',(-1.22460635382238E-16,-1.,-2.46519032881566E-32));
#23739=DIRECTION('ref_axis',(-3.01888774004913E-48,-2.46519032881566E-32,
1.));
#23740=DIRECTION('center_axis',(-1.22460635382238E-16,-1.,-2.46519032881566E-32));
#23741=DIRECTION('ref_axis',(-3.01888774004913E-48,-2.46519032881566E-32,
1.));
#23742=DIRECTION('center_axis',(-1.22460635382238E-16,-1.,-2.46519032881566E-32));
#23743=DIRECTION('ref_axis',(-3.01888774004913E-48,-2.46519032881566E-32,
1.));
#23744=DIRECTION('center_axis',(-1.22460635382238E-16,-1.,-2.46519032881566E-32));
#23745=DIRECTION('ref_axis',(-3.01888774004913E-48,-2.46519032881566E-32,
1.));
#23746=DIRECTION('center_axis',(-1.22460635382238E-16,-1.,-2.46519032881566E-32));
#23747=DIRECTION('ref_axis',(-3.01888774004913E-48,-2.46519032881566E-32,
1.));
#23748=DIRECTION('center_axis',(-1.22460635382238E-16,-1.,-2.46519032881566E-32));
#23749=DIRECTION('ref_axis',(-3.01888774004913E-48,-2.46519032881566E-32,
1.));
#23750=DIRECTION('center_axis',(-1.22460635382238E-16,-1.,-2.46519032881566E-32));
#23751=DIRECTION('ref_axis',(-3.01888774004913E-48,-2.46519032881566E-32,
1.));
#23752=DIRECTION('center_axis',(-1.22460635382238E-16,-1.,-2.46519032881566E-32));
#23753=DIRECTION('ref_axis',(-3.01888774004913E-48,-2.46519032881566E-32,
1.));
#23754=DIRECTION('center_axis',(-1.22460635382238E-16,-1.,-2.46519032881566E-32));
#23755=DIRECTION('ref_axis',(-3.01888774004913E-48,-2.46519032881566E-32,
1.));
#23756=DIRECTION('center_axis',(-1.22460635382238E-16,-1.,-2.46519032881566E-32));
#23757=DIRECTION('ref_axis',(-3.01888774004913E-48,-2.46519032881566E-32,
1.));
#23758=DIRECTION('center_axis',(-1.22460635382238E-16,-1.,-2.46519032881566E-32));
#23759=DIRECTION('ref_axis',(-3.01888774004913E-48,-2.46519032881566E-32,
1.));
#23760=DIRECTION('center_axis',(-1.22460635382238E-16,-1.,-2.46519032881566E-32));
#23761=DIRECTION('ref_axis',(-3.01888774004913E-48,-2.46519032881566E-32,
1.));
#23762=DIRECTION('center_axis',(-1.22460635382238E-16,-1.,-2.46519032881566E-32));
#23763=DIRECTION('ref_axis',(-3.01888774004913E-48,-2.46519032881566E-32,
1.));
#23764=DIRECTION('center_axis',(-1.22460635382238E-16,-1.,-2.46519032881566E-32));
#23765=DIRECTION('ref_axis',(-3.01888774004913E-48,-2.46519032881566E-32,
1.));
#23766=DIRECTION('center_axis',(-1.22460635382238E-16,-1.,-2.46519032881566E-32));
#23767=DIRECTION('ref_axis',(-3.01888774004913E-48,-2.46519032881566E-32,
1.));
#23768=DIRECTION('center_axis',(-1.22460635382238E-16,-1.,-2.46519032881566E-32));
#23769=DIRECTION('ref_axis',(-3.01888774004913E-48,-2.46519032881566E-32,
1.));
#23770=DIRECTION('center_axis',(-1.22460635382238E-16,-1.,-2.46519032881566E-32));
#23771=DIRECTION('ref_axis',(-3.01888774004913E-48,-2.46519032881566E-32,
1.));
#23772=DIRECTION('center_axis',(-1.22460635382238E-16,-1.,-2.46519032881566E-32));
#23773=DIRECTION('ref_axis',(-3.01888774004913E-48,-2.46519032881566E-32,
1.));
#23774=DIRECTION('center_axis',(-1.22460635382238E-16,-1.,-2.46519032881566E-32));
#23775=DIRECTION('ref_axis',(-3.01888774004913E-48,-2.46519032881566E-32,
1.));
#23776=DIRECTION('center_axis',(-1.22460635382238E-16,-1.,-2.46519032881566E-32));
#23777=DIRECTION('ref_axis',(-3.01888774004913E-48,-2.46519032881566E-32,
1.));
#23778=DIRECTION('center_axis',(-1.22460635382238E-16,-1.,-2.46519032881566E-32));
#23779=DIRECTION('ref_axis',(-3.01888774004913E-48,-2.46519032881566E-32,
1.));
#23780=DIRECTION('center_axis',(-1.22460635382238E-16,-1.,-2.46519032881566E-32));
#23781=DIRECTION('ref_axis',(-3.01888774004913E-48,-2.46519032881566E-32,
1.));
#23782=DIRECTION('center_axis',(-1.22460635382238E-16,-1.,-2.46519032881566E-32));
#23783=DIRECTION('ref_axis',(-3.01888774004913E-48,-2.46519032881566E-32,
1.));
#23784=DIRECTION('center_axis',(-1.22460635382238E-16,-1.,-2.46519032881566E-32));
#23785=DIRECTION('ref_axis',(-3.01888774004913E-48,-2.46519032881566E-32,
1.));
#23786=DIRECTION('',(-1.73188351330743E-16,-0.707106781186547,-0.707106781186548));
#23787=DIRECTION('center_axis',(-1.22460635382238E-16,-1.,-2.46519032881566E-32));
#23788=DIRECTION('ref_axis',(-3.01888774004913E-48,-2.46519032881566E-32,
1.));
#23789=DIRECTION('center_axis',(-1.22460635382238E-16,-1.,-2.46519032881566E-32));
#23790=DIRECTION('ref_axis',(-3.01888774004913E-48,-2.46519032881566E-32,
1.));
#23791=DIRECTION('center_axis',(-1.22460635382238E-16,-1.,-2.46519032881566E-32));
#23792=DIRECTION('ref_axis',(-3.01888774004913E-48,-2.46519032881566E-32,
1.));
#23793=DIRECTION('center_axis',(-1.22460635382238E-16,-1.,-2.46519032881566E-32));
#23794=DIRECTION('ref_axis',(-3.01888774004913E-48,-2.46519032881566E-32,
1.));
#23795=DIRECTION('center_axis',(-1.22460635382238E-16,-1.,-2.46519032881566E-32));
#23796=DIRECTION('ref_axis',(-3.01888774004913E-48,-2.46519032881566E-32,
1.));
#23797=DIRECTION('center_axis',(-1.22460635382238E-16,-1.,-2.46519032881566E-32));
#23798=DIRECTION('ref_axis',(-3.01888774004913E-48,-2.46519032881566E-32,
1.));
#23799=DIRECTION('center_axis',(-1.22460635382238E-16,-1.,-2.46519032881566E-32));
#23800=DIRECTION('ref_axis',(-3.01888774004913E-48,-2.46519032881566E-32,
1.));
#23801=DIRECTION('center_axis',(-1.22460635382238E-16,-1.,-2.46519032881566E-32));
#23802=DIRECTION('ref_axis',(-3.01888774004913E-48,-2.46519032881566E-32,
1.));
#23803=DIRECTION('center_axis',(-1.22460635382238E-16,-1.,-2.46519032881566E-32));
#23804=DIRECTION('ref_axis',(-3.01888774004913E-48,-2.46519032881566E-32,
1.));
#23805=DIRECTION('center_axis',(-1.22460635382238E-16,-1.,-2.46519032881566E-32));
#23806=DIRECTION('ref_axis',(-3.01888774004913E-48,-2.46519032881566E-32,
1.));
#23807=DIRECTION('center_axis',(-1.22460635382238E-16,-1.,-2.46519032881566E-32));
#23808=DIRECTION('ref_axis',(-3.01888774004913E-48,-2.46519032881566E-32,
1.));
#23809=DIRECTION('center_axis',(-1.22460635382238E-16,-1.,-2.46519032881566E-32));
#23810=DIRECTION('ref_axis',(-3.01888774004913E-48,-2.46519032881566E-32,
1.));
#23811=DIRECTION('center_axis',(-1.22460635382238E-16,-1.,-2.46519032881566E-32));
#23812=DIRECTION('ref_axis',(-3.01888774004913E-48,-2.46519032881566E-32,
1.));
#23813=DIRECTION('center_axis',(-1.22460635382238E-16,-1.,-2.46519032881566E-32));
#23814=DIRECTION('ref_axis',(-3.01888774004913E-48,-2.46519032881566E-32,
1.));
#23815=DIRECTION('center_axis',(-1.22460635382238E-16,-1.,-2.46519032881566E-32));
#23816=DIRECTION('ref_axis',(-3.01888774004913E-48,-2.46519032881566E-32,
1.));
#23817=DIRECTION('center_axis',(-1.22460635382238E-16,-1.,-2.46519032881566E-32));
#23818=DIRECTION('ref_axis',(-3.01888774004913E-48,-2.46519032881566E-32,
1.));
#23819=DIRECTION('center_axis',(-1.22460635382238E-16,-1.,-2.46519032881566E-32));
#23820=DIRECTION('ref_axis',(-3.01888774004913E-48,-2.46519032881566E-32,
1.));
#23821=DIRECTION('center_axis',(-1.22460635382238E-16,-1.,-2.46519032881566E-32));
#23822=DIRECTION('ref_axis',(-3.01888774004913E-48,-2.46519032881566E-32,
1.));
#23823=DIRECTION('center_axis',(-1.22460635382238E-16,-1.,-2.46519032881566E-32));
#23824=DIRECTION('ref_axis',(-3.01888774004913E-48,-2.46519032881566E-32,
1.));
#23825=DIRECTION('center_axis',(-1.22460635382238E-16,-1.,-2.46519032881566E-32));
#23826=DIRECTION('ref_axis',(-3.01888774004913E-48,-2.46519032881566E-32,
1.));
#23827=DIRECTION('center_axis',(-1.22460635382238E-16,-1.,-2.46519032881566E-32));
#23828=DIRECTION('ref_axis',(-3.01888774004913E-48,-2.46519032881566E-32,
1.));
#23829=DIRECTION('center_axis',(-1.22460635382238E-16,-1.,-2.46519032881566E-32));
#23830=DIRECTION('ref_axis',(-3.01888774004913E-48,-2.46519032881566E-32,
1.));
#23831=DIRECTION('center_axis',(-1.22460635382238E-16,-1.,-2.46519032881566E-32));
#23832=DIRECTION('ref_axis',(-3.01888774004913E-48,-2.46519032881566E-32,
1.));
#23833=DIRECTION('center_axis',(-1.22460635382238E-16,-1.,-2.46519032881566E-32));
#23834=DIRECTION('ref_axis',(-3.01888774004913E-48,-2.46519032881566E-32,
1.));
#23835=DIRECTION('center_axis',(-1.22460635382238E-16,-1.,-2.46519032881566E-32));
#23836=DIRECTION('ref_axis',(-3.01888774004913E-48,-2.46519032881566E-32,
1.));
#23837=DIRECTION('center_axis',(-1.22460635382238E-16,-1.,-2.46519032881566E-32));
#23838=DIRECTION('ref_axis',(-3.01888774004913E-48,-2.46519032881566E-32,
1.));
#23839=DIRECTION('center_axis',(-1.22460635382238E-16,-1.,-2.46519032881566E-32));
#23840=DIRECTION('ref_axis',(-3.01888774004913E-48,-2.46519032881566E-32,
1.));
#23841=DIRECTION('center_axis',(-1.22460635382238E-16,-1.,-2.46519032881566E-32));
#23842=DIRECTION('ref_axis',(-3.01888774004913E-48,-2.46519032881566E-32,
1.));
#23843=DIRECTION('center_axis',(-1.22460635382238E-16,-1.,-2.46519032881566E-32));
#23844=DIRECTION('ref_axis',(-3.01888774004913E-48,-2.46519032881566E-32,
1.));
#23845=DIRECTION('center_axis',(-1.22460635382238E-16,-1.,-2.46519032881566E-32));
#23846=DIRECTION('ref_axis',(-3.01888774004913E-48,-2.46519032881566E-32,
1.));
#23847=DIRECTION('center_axis',(-1.22460635382238E-16,-1.,-2.46519032881566E-32));
#23848=DIRECTION('ref_axis',(-3.01888774004913E-48,-2.46519032881566E-32,
1.));
#23849=DIRECTION('center_axis',(-1.22460635382238E-16,-1.,-2.46519032881566E-32));
#23850=DIRECTION('ref_axis',(-3.01888774004913E-48,-2.46519032881566E-32,
1.));
#23851=DIRECTION('center_axis',(-1.22460635382238E-16,-1.,-2.46519032881566E-32));
#23852=DIRECTION('ref_axis',(-3.01888774004913E-48,-2.46519032881566E-32,
1.));
#23853=DIRECTION('center_axis',(-1.22460635382238E-16,-1.,-2.46519032881566E-32));
#23854=DIRECTION('ref_axis',(-3.01888774004913E-48,-2.46519032881566E-32,
1.));
#23855=DIRECTION('center_axis',(-1.22460635382238E-16,-1.,-2.46519032881566E-32));
#23856=DIRECTION('ref_axis',(-3.01888774004913E-48,-2.46519032881566E-32,
1.));
#23857=DIRECTION('center_axis',(-1.22460635382238E-16,-1.,-2.46519032881566E-32));
#23858=DIRECTION('ref_axis',(-3.01888774004913E-48,-2.46519032881566E-32,
1.));
#23859=DIRECTION('center_axis',(-1.22460635382238E-16,-1.,-2.46519032881566E-32));
#23860=DIRECTION('ref_axis',(-3.01888774004913E-48,-2.46519032881566E-32,
1.));
#23861=DIRECTION('center_axis',(-1.22460635382238E-16,-1.,-2.46519032881566E-32));
#23862=DIRECTION('ref_axis',(-3.01888774004913E-48,-2.46519032881566E-32,
1.));
#23863=DIRECTION('center_axis',(-1.22460635382238E-16,-1.,-2.46519032881566E-32));
#23864=DIRECTION('ref_axis',(-3.01888774004913E-48,-2.46519032881566E-32,
1.));
#23865=DIRECTION('center_axis',(-1.22460635382238E-16,-1.,-2.46519032881566E-32));
#23866=DIRECTION('ref_axis',(-3.01888774004913E-48,-2.46519032881566E-32,
1.));
#23867=DIRECTION('center_axis',(-1.22460635382238E-16,-1.,-2.46519032881566E-32));
#23868=DIRECTION('ref_axis',(-3.01888774004913E-48,-2.46519032881566E-32,
1.));
#23869=DIRECTION('',(1.22460635382238E-16,1.,2.46519032881566E-32));
#23870=DIRECTION('center_axis',(-1.22460635382238E-16,-1.,-2.46519032881566E-32));
#23871=DIRECTION('ref_axis',(-3.01888774004913E-48,-2.46519032881566E-32,
1.));
#23872=DIRECTION('',(-1.22460635382238E-16,-1.,-2.46519032881566E-32));
#23873=DIRECTION('',(-1.22460635382238E-16,-1.,-2.46519032881566E-32));
#23874=DIRECTION('center_axis',(-1.22460635382238E-16,-1.,-2.46519032881566E-32));
#23875=DIRECTION('ref_axis',(-3.01888774004913E-48,-2.46519032881566E-32,
1.));
#23876=DIRECTION('',(-1.22460635382238E-16,-1.,-2.46519032881566E-32));
#23877=DIRECTION('',(-1.22460635382238E-16,-1.,-2.46519032881566E-32));
#23878=DIRECTION('center_axis',(-1.22460635382238E-16,-1.,-2.46519032881566E-32));
#23879=DIRECTION('ref_axis',(-3.01888774004913E-48,-2.46519032881566E-32,
1.));
#23880=DIRECTION('',(-1.22460635382238E-16,-1.,-2.46519032881566E-32));
#23881=DIRECTION('',(-1.22460635382238E-16,-1.,-2.46519032881566E-32));
#23882=DIRECTION('center_axis',(-1.22460635382238E-16,-1.,-2.46519032881566E-32));
#23883=DIRECTION('ref_axis',(-3.01888774004913E-48,-2.46519032881566E-32,
1.));
#23884=DIRECTION('',(-1.22460635382238E-16,-1.,-2.46519032881566E-32));
#23885=DIRECTION('',(-1.22460635382238E-16,-1.,-2.46519032881566E-32));
#23886=DIRECTION('center_axis',(-1.22460635382238E-16,-1.,-2.46519032881566E-32));
#23887=DIRECTION('ref_axis',(-3.01888774004913E-48,-2.46519032881566E-32,
1.));
#23888=DIRECTION('',(-1.22460635382238E-16,-1.,-2.46519032881566E-32));
#23889=DIRECTION('',(-1.22460635382238E-16,-1.,-2.46519032881566E-32));
#23890=DIRECTION('center_axis',(-1.22460635382238E-16,-1.,-2.46519032881566E-32));
#23891=DIRECTION('ref_axis',(-3.01888774004913E-48,-2.46519032881566E-32,
1.));
#23892=DIRECTION('',(-1.22460635382238E-16,-1.,-2.46519032881566E-32));
#23893=DIRECTION('',(-1.22460635382238E-16,-1.,-2.46519032881566E-32));
#23894=DIRECTION('center_axis',(-1.22460635382238E-16,-1.,-2.46519032881566E-32));
#23895=DIRECTION('ref_axis',(-3.01888774004913E-48,-2.46519032881566E-32,
1.));
#23896=DIRECTION('',(-1.22460635382238E-16,-1.,-2.46519032881566E-32));
#23897=DIRECTION('',(-1.22460635382238E-16,-1.,-2.46519032881566E-32));
#23898=DIRECTION('center_axis',(-1.22460635382238E-16,-1.,-2.46519032881566E-32));
#23899=DIRECTION('ref_axis',(-3.01888774004913E-48,-2.46519032881566E-32,
1.));
#23900=DIRECTION('',(-1.22460635382238E-16,-1.,-2.46519032881566E-32));
#23901=DIRECTION('',(-1.22460635382238E-16,-1.,-2.46519032881566E-32));
#23902=DIRECTION('center_axis',(-1.22460635382238E-16,-1.,-2.46519032881566E-32));
#23903=DIRECTION('ref_axis',(-3.01888774004913E-48,-2.46519032881566E-32,
1.));
#23904=DIRECTION('',(-1.22460635382238E-16,-1.,-2.46519032881566E-32));
#23905=DIRECTION('',(-1.22460635382238E-16,-1.,-2.46519032881566E-32));
#23906=DIRECTION('center_axis',(-1.22460635382238E-16,-1.,-2.46519032881566E-32));
#23907=DIRECTION('ref_axis',(-3.01888774004913E-48,-2.46519032881566E-32,
1.));
#23908=DIRECTION('',(-1.22460635382238E-16,-1.,-2.46519032881566E-32));
#23909=DIRECTION('',(-1.22460635382238E-16,-1.,-2.46519032881566E-32));
#23910=DIRECTION('center_axis',(-1.22460635382238E-16,-1.,-2.46519032881566E-32));
#23911=DIRECTION('ref_axis',(-3.01888774004913E-48,-2.46519032881566E-32,
1.));
#23912=DIRECTION('',(-1.22460635382238E-16,-1.,-2.46519032881566E-32));
#23913=DIRECTION('',(-1.22460635382238E-16,-1.,-2.46519032881566E-32));
#23914=DIRECTION('center_axis',(-1.22460635382238E-16,-1.,-2.46519032881566E-32));
#23915=DIRECTION('ref_axis',(-3.01888774004913E-48,-2.46519032881566E-32,
1.));
#23916=DIRECTION('',(-1.22460635382238E-16,-1.,-2.46519032881566E-32));
#23917=DIRECTION('',(-1.22460635382238E-16,-1.,-2.46519032881566E-32));
#23918=DIRECTION('center_axis',(-1.22460635382238E-16,-1.,-2.46519032881566E-32));
#23919=DIRECTION('ref_axis',(-3.01888774004913E-48,-2.46519032881566E-32,
1.));
#23920=DIRECTION('',(-1.22460635382238E-16,-1.,-2.46519032881566E-32));
#23921=DIRECTION('',(-1.22460635382238E-16,-1.,-2.46519032881566E-32));
#23922=DIRECTION('center_axis',(-1.22460635382238E-16,-1.,-2.46519032881566E-32));
#23923=DIRECTION('ref_axis',(-3.01888774004913E-48,-2.46519032881566E-32,
1.));
#23924=DIRECTION('',(-1.22460635382238E-16,-1.,-2.46519032881566E-32));
#23925=DIRECTION('',(-1.22460635382238E-16,-1.,-2.46519032881566E-32));
#23926=DIRECTION('center_axis',(-1.22460635382238E-16,-1.,-2.46519032881566E-32));
#23927=DIRECTION('ref_axis',(-3.01888774004913E-48,-2.46519032881566E-32,
1.));
#23928=DIRECTION('',(-1.22460635382238E-16,-1.,-2.46519032881566E-32));
#23929=DIRECTION('',(-1.22460635382238E-16,-1.,-2.46519032881566E-32));
#23930=DIRECTION('center_axis',(-1.22460635382238E-16,-1.,-2.46519032881566E-32));
#23931=DIRECTION('ref_axis',(-3.01888774004913E-48,-2.46519032881566E-32,
1.));
#23932=DIRECTION('',(-1.22460635382238E-16,-1.,-2.46519032881566E-32));
#23933=DIRECTION('',(-1.22460635382238E-16,-1.,-2.46519032881566E-32));
#23934=DIRECTION('center_axis',(-1.22460635382238E-16,-1.,-2.46519032881566E-32));
#23935=DIRECTION('ref_axis',(-3.01888774004913E-48,-2.46519032881566E-32,
1.));
#23936=DIRECTION('',(-1.22460635382238E-16,-1.,-2.46519032881566E-32));
#23937=DIRECTION('',(-1.22460635382238E-16,-1.,-2.46519032881566E-32));
#23938=DIRECTION('center_axis',(-1.22460635382238E-16,-1.,-2.46519032881566E-32));
#23939=DIRECTION('ref_axis',(-3.01888774004913E-48,-2.46519032881566E-32,
1.));
#23940=DIRECTION('',(-1.22460635382238E-16,-1.,-2.46519032881566E-32));
#23941=DIRECTION('',(-1.22460635382238E-16,-1.,-2.46519032881566E-32));
#23942=DIRECTION('center_axis',(-1.22460635382238E-16,-1.,-2.46519032881566E-32));
#23943=DIRECTION('ref_axis',(-3.01888774004913E-48,-2.46519032881566E-32,
1.));
#23944=DIRECTION('',(-1.22460635382238E-16,-1.,-2.46519032881566E-32));
#23945=DIRECTION('',(-1.22460635382238E-16,-1.,-2.46519032881566E-32));
#23946=DIRECTION('center_axis',(-1.22460635382238E-16,-1.,-2.46519032881566E-32));
#23947=DIRECTION('ref_axis',(-3.01888774004913E-48,-2.46519032881566E-32,
1.));
#23948=DIRECTION('',(-1.22460635382238E-16,-1.,-2.46519032881566E-32));
#23949=DIRECTION('',(-1.22460635382238E-16,-1.,-2.46519032881566E-32));
#23950=DIRECTION('center_axis',(-1.22460635382238E-16,-1.,-2.46519032881566E-32));
#23951=DIRECTION('ref_axis',(-3.01888774004913E-48,-2.46519032881566E-32,
1.));
#23952=DIRECTION('',(-1.22460635382238E-16,-1.,-2.46519032881566E-32));
#23953=DIRECTION('',(-1.22460635382238E-16,-1.,-2.46519032881566E-32));
#23954=DIRECTION('center_axis',(-1.22460635382238E-16,-1.,-2.46519032881566E-32));
#23955=DIRECTION('ref_axis',(-3.01888774004913E-48,-2.46519032881566E-32,
1.));
#23956=DIRECTION('',(-1.22460635382238E-16,-1.,-2.46519032881566E-32));
#23957=DIRECTION('',(-1.22460635382238E-16,-1.,-2.46519032881566E-32));
#23958=DIRECTION('center_axis',(-1.22460635382238E-16,-1.,-2.46519032881566E-32));
#23959=DIRECTION('ref_axis',(-3.01888774004913E-48,-2.46519032881566E-32,
1.));
#23960=DIRECTION('',(-1.22460635382238E-16,-1.,-2.46519032881566E-32));
#23961=DIRECTION('',(-1.22460635382238E-16,-1.,-2.46519032881566E-32));
#23962=DIRECTION('center_axis',(-1.22460635382238E-16,-1.,-2.46519032881566E-32));
#23963=DIRECTION('ref_axis',(-3.01888774004913E-48,-2.46519032881566E-32,
1.));
#23964=DIRECTION('',(-1.22460635382238E-16,-1.,-2.46519032881566E-32));
#23965=DIRECTION('',(-1.22460635382238E-16,-1.,-2.46519032881566E-32));
#23966=DIRECTION('center_axis',(-1.22460635382238E-16,-1.,-2.46519032881566E-32));
#23967=DIRECTION('ref_axis',(-3.01888774004913E-48,-2.46519032881566E-32,
1.));
#23968=DIRECTION('',(-1.22460635382238E-16,-1.,-2.46519032881566E-32));
#23969=DIRECTION('',(-1.22460635382238E-16,-1.,-2.46519032881566E-32));
#23970=DIRECTION('center_axis',(-1.22460635382238E-16,-1.,-2.46519032881566E-32));
#23971=DIRECTION('ref_axis',(-3.01888774004913E-48,-2.46519032881566E-32,
1.));
#23972=DIRECTION('',(-1.22460635382238E-16,-1.,-2.46519032881566E-32));
#23973=DIRECTION('',(-1.22460635382238E-16,-1.,-2.46519032881566E-32));
#23974=DIRECTION('center_axis',(-1.22460635382238E-16,-1.,-2.46519032881566E-32));
#23975=DIRECTION('ref_axis',(-3.01888774004913E-48,-2.46519032881566E-32,
1.));
#23976=DIRECTION('',(-1.22460635382238E-16,-1.,-2.46519032881566E-32));
#23977=DIRECTION('',(-1.22460635382238E-16,-1.,-2.46519032881566E-32));
#23978=DIRECTION('center_axis',(-1.22460635382238E-16,-1.,-2.46519032881566E-32));
#23979=DIRECTION('ref_axis',(-3.01888774004913E-48,-2.46519032881566E-32,
1.));
#23980=DIRECTION('',(-1.22460635382238E-16,-1.,-2.46519032881566E-32));
#23981=DIRECTION('',(-1.22460635382238E-16,-1.,-2.46519032881566E-32));
#23982=DIRECTION('center_axis',(-1.22460635382238E-16,-1.,-2.46519032881566E-32));
#23983=DIRECTION('ref_axis',(-3.01888774004913E-48,-2.46519032881566E-32,
1.));
#23984=DIRECTION('',(-1.22460635382238E-16,-1.,-2.46519032881566E-32));
#23985=DIRECTION('',(-1.22460635382238E-16,-1.,-2.46519032881566E-32));
#23986=DIRECTION('center_axis',(-1.22460635382238E-16,-1.,-2.46519032881566E-32));
#23987=DIRECTION('ref_axis',(-3.01888774004913E-48,-2.46519032881566E-32,
1.));
#23988=DIRECTION('',(-1.22460635382238E-16,-1.,-2.46519032881566E-32));
#23989=DIRECTION('',(-1.22460635382238E-16,-1.,-2.46519032881566E-32));
#23990=DIRECTION('center_axis',(-1.22460635382238E-16,-1.,-2.46519032881566E-32));
#23991=DIRECTION('ref_axis',(-3.01888774004913E-48,-2.46519032881566E-32,
1.));
#23992=DIRECTION('',(-1.22460635382238E-16,-1.,-2.46519032881566E-32));
#23993=DIRECTION('',(-1.22460635382238E-16,-1.,-2.46519032881566E-32));
#23994=DIRECTION('center_axis',(-1.22460635382238E-16,-1.,-2.46519032881566E-32));
#23995=DIRECTION('ref_axis',(-3.01888774004913E-48,-2.46519032881566E-32,
1.));
#23996=DIRECTION('',(-1.22460635382238E-16,-1.,-2.46519032881566E-32));
#23997=DIRECTION('',(-1.22460635382238E-16,-1.,-2.46519032881566E-32));
#23998=DIRECTION('center_axis',(-1.22460635382238E-16,-1.,-2.46519032881566E-32));
#23999=DIRECTION('ref_axis',(-3.01888774004913E-48,-2.46519032881566E-32,
1.));
#24000=DIRECTION('',(-1.22460635382238E-16,-1.,-2.46519032881566E-32));
#24001=DIRECTION('',(-1.22460635382238E-16,-1.,-2.46519032881566E-32));
#24002=DIRECTION('center_axis',(-1.22460635382238E-16,-1.,-2.46519032881566E-32));
#24003=DIRECTION('ref_axis',(-3.01888774004913E-48,-2.46519032881566E-32,
1.));
#24004=DIRECTION('',(-1.22460635382238E-16,-1.,-2.46519032881566E-32));
#24005=DIRECTION('',(-1.22460635382238E-16,-1.,-2.46519032881566E-32));
#24006=DIRECTION('center_axis',(-1.22460635382238E-16,-1.,-2.46519032881566E-32));
#24007=DIRECTION('ref_axis',(-3.01888774004913E-48,-2.46519032881566E-32,
1.));
#24008=DIRECTION('',(-1.22460635382238E-16,-1.,-2.46519032881566E-32));
#24009=DIRECTION('',(-1.22460635382238E-16,-1.,-2.46519032881566E-32));
#24010=DIRECTION('center_axis',(-1.22460635382238E-16,-1.,-2.46519032881566E-32));
#24011=DIRECTION('ref_axis',(-3.01888774004913E-48,-2.46519032881566E-32,
1.));
#24012=DIRECTION('',(-1.22460635382238E-16,-1.,-2.46519032881566E-32));
#24013=DIRECTION('',(-1.22460635382238E-16,-1.,-2.46519032881566E-32));
#24014=DIRECTION('center_axis',(-1.22460635382238E-16,-1.,-2.46519032881566E-32));
#24015=DIRECTION('ref_axis',(-3.01888774004913E-48,-2.46519032881566E-32,
1.));
#24016=DIRECTION('',(-1.22460635382238E-16,-1.,-2.46519032881566E-32));
#24017=DIRECTION('',(-1.22460635382238E-16,-1.,-2.46519032881566E-32));
#24018=DIRECTION('center_axis',(-1.22460635382238E-16,-1.,-2.46519032881566E-32));
#24019=DIRECTION('ref_axis',(-3.01888774004913E-48,-2.46519032881566E-32,
1.));
#24020=DIRECTION('',(-1.22460635382238E-16,-1.,-2.46519032881566E-32));
#24021=DIRECTION('',(-1.22460635382238E-16,-1.,-2.46519032881566E-32));
#24022=DIRECTION('center_axis',(-1.22460635382238E-16,-1.,-2.46519032881566E-32));
#24023=DIRECTION('ref_axis',(-3.01888774004913E-48,-2.46519032881566E-32,
1.));
#24024=DIRECTION('',(-1.22460635382238E-16,-1.,-2.46519032881566E-32));
#24025=DIRECTION('',(-1.22460635382238E-16,-1.,-2.46519032881566E-32));
#24026=DIRECTION('center_axis',(-1.22460635382238E-16,-1.,-2.46519032881566E-32));
#24027=DIRECTION('ref_axis',(-3.01888774004913E-48,-2.46519032881566E-32,
1.));
#24028=DIRECTION('',(-1.22460635382238E-16,-1.,-2.46519032881566E-32));
#24029=DIRECTION('',(-1.22460635382238E-16,-1.,-2.46519032881566E-32));
#24030=DIRECTION('center_axis',(-1.22460635382238E-16,-1.,-2.46519032881566E-32));
#24031=DIRECTION('ref_axis',(-3.01888774004913E-48,-2.46519032881566E-32,
1.));
#24032=DIRECTION('',(-1.22460635382238E-16,-1.,-2.46519032881566E-32));
#24033=DIRECTION('',(-1.22460635382238E-16,-1.,-2.46519032881566E-32));
#24034=DIRECTION('center_axis',(-1.22460635382238E-16,-1.,-2.46519032881566E-32));
#24035=DIRECTION('ref_axis',(-3.01888774004913E-48,-2.46519032881566E-32,
1.));
#24036=DIRECTION('',(-1.22460635382238E-16,-1.,-2.46519032881566E-32));
#24037=DIRECTION('',(-1.22460635382238E-16,-1.,-2.46519032881566E-32));
#24038=DIRECTION('center_axis',(-1.22460635382238E-16,-1.,-2.46519032881566E-32));
#24039=DIRECTION('ref_axis',(-3.01888774004913E-48,-2.46519032881566E-32,
1.));
#24040=DIRECTION('',(-1.22460635382238E-16,-1.,-2.46519032881566E-32));
#24041=DIRECTION('',(-1.22460635382238E-16,-1.,-2.46519032881566E-32));
#24042=DIRECTION('center_axis',(-1.22460635382238E-16,-1.,-2.46519032881566E-32));
#24043=DIRECTION('ref_axis',(-3.01888774004913E-48,-2.46519032881566E-32,
1.));
#24044=DIRECTION('',(-1.22460635382238E-16,-1.,-2.46519032881566E-32));
#24045=DIRECTION('',(-1.22460635382238E-16,-1.,-2.46519032881566E-32));
#24046=DIRECTION('center_axis',(-1.22460635382238E-16,-1.,-2.46519032881566E-32));
#24047=DIRECTION('ref_axis',(-3.01888774004913E-48,-2.46519032881566E-32,
1.));
#24048=DIRECTION('',(-1.22460635382238E-16,-1.,-2.46519032881566E-32));
#24049=DIRECTION('',(-1.22460635382238E-16,-1.,-2.46519032881566E-32));
#24050=DIRECTION('center_axis',(-1.22460635382238E-16,-1.,-2.46519032881566E-32));
#24051=DIRECTION('ref_axis',(-3.01888774004913E-48,-2.46519032881566E-32,
1.));
#24052=DIRECTION('',(-1.22460635382238E-16,-1.,-2.46519032881566E-32));
#24053=DIRECTION('',(-1.22460635382238E-16,-1.,-2.46519032881566E-32));
#24054=DIRECTION('center_axis',(-1.22460635382238E-16,-1.,-2.46519032881566E-32));
#24055=DIRECTION('ref_axis',(-3.01888774004913E-48,-2.46519032881566E-32,
1.));
#24056=DIRECTION('',(-1.22460635382238E-16,-1.,-2.46519032881566E-32));
#24057=DIRECTION('',(-1.22460635382238E-16,-1.,-2.46519032881566E-32));
#24058=DIRECTION('center_axis',(-1.22460635382238E-16,-1.,-2.46519032881566E-32));
#24059=DIRECTION('ref_axis',(-3.01888774004913E-48,-2.46519032881566E-32,
1.));
#24060=DIRECTION('',(-1.22460635382238E-16,-1.,-2.46519032881566E-32));
#24061=DIRECTION('',(-1.22460635382238E-16,-1.,-2.46519032881566E-32));
#24062=DIRECTION('center_axis',(-1.22460635382238E-16,-1.,-2.46519032881566E-32));
#24063=DIRECTION('ref_axis',(-3.01888774004913E-48,-2.46519032881566E-32,
1.));
#24064=DIRECTION('',(-1.22460635382238E-16,-1.,-2.46519032881566E-32));
#24065=DIRECTION('',(-1.22460635382238E-16,-1.,-2.46519032881566E-32));
#24066=DIRECTION('center_axis',(-1.22460635382238E-16,-1.,-2.46519032881566E-32));
#24067=DIRECTION('ref_axis',(-3.01888774004913E-48,-2.46519032881566E-32,
1.));
#24068=DIRECTION('',(-1.22460635382238E-16,-1.,-2.46519032881566E-32));
#24069=DIRECTION('',(-1.22460635382238E-16,-1.,-2.46519032881566E-32));
#24070=DIRECTION('center_axis',(-1.22460635382238E-16,-1.,-2.46519032881566E-32));
#24071=DIRECTION('ref_axis',(-3.01888774004913E-48,-2.46519032881566E-32,
1.));
#24072=DIRECTION('',(-1.22460635382238E-16,-1.,-2.46519032881566E-32));
#24073=DIRECTION('',(-1.22460635382238E-16,-1.,-2.46519032881566E-32));
#24074=DIRECTION('center_axis',(-1.22460635382238E-16,-1.,-2.46519032881566E-32));
#24075=DIRECTION('ref_axis',(-3.01888774004913E-48,-2.46519032881566E-32,
1.));
#24076=DIRECTION('',(-1.22460635382238E-16,-1.,-2.46519032881566E-32));
#24077=DIRECTION('',(-1.22460635382238E-16,-1.,-2.46519032881566E-32));
#24078=DIRECTION('center_axis',(-1.22460635382238E-16,-1.,-2.46519032881566E-32));
#24079=DIRECTION('ref_axis',(-3.01888774004913E-48,-2.46519032881566E-32,
1.));
#24080=DIRECTION('',(-1.22460635382238E-16,-1.,-2.46519032881566E-32));
#24081=DIRECTION('',(-1.22460635382238E-16,-1.,-2.46519032881566E-32));
#24082=DIRECTION('center_axis',(-1.22460635382238E-16,-1.,-2.46519032881566E-32));
#24083=DIRECTION('ref_axis',(-3.01888774004913E-48,-2.46519032881566E-32,
1.));
#24084=DIRECTION('',(-1.22460635382238E-16,-1.,-2.46519032881566E-32));
#24085=DIRECTION('',(-1.22460635382238E-16,-1.,-2.46519032881566E-32));
#24086=DIRECTION('center_axis',(-1.22460635382238E-16,-1.,-2.46519032881566E-32));
#24087=DIRECTION('ref_axis',(-3.01888774004913E-48,-2.46519032881566E-32,
1.));
#24088=DIRECTION('',(-1.22460635382238E-16,-1.,-2.46519032881566E-32));
#24089=DIRECTION('',(-1.22460635382238E-16,-1.,-2.46519032881566E-32));
#24090=DIRECTION('center_axis',(-1.22460635382238E-16,-1.,-2.46519032881566E-32));
#24091=DIRECTION('ref_axis',(-3.01888774004913E-48,-2.46519032881566E-32,
1.));
#24092=DIRECTION('',(-1.22460635382238E-16,-1.,-2.46519032881566E-32));
#24093=DIRECTION('',(-1.22460635382238E-16,-1.,-2.46519032881566E-32));
#24094=DIRECTION('center_axis',(-1.22460635382238E-16,-1.,-2.46519032881566E-32));
#24095=DIRECTION('ref_axis',(-3.01888774004913E-48,-2.46519032881566E-32,
1.));
#24096=DIRECTION('',(-1.22460635382238E-16,-1.,-2.46519032881566E-32));
#24097=DIRECTION('',(-1.22460635382238E-16,-1.,-2.46519032881566E-32));
#24098=DIRECTION('center_axis',(-1.22460635382238E-16,-1.,-2.46519032881566E-32));
#24099=DIRECTION('ref_axis',(-3.01888774004913E-48,-2.46519032881566E-32,
1.));
#24100=DIRECTION('',(-1.22460635382238E-16,-1.,-2.46519032881566E-32));
#24101=DIRECTION('',(-1.22460635382238E-16,-1.,-2.46519032881566E-32));
#24102=DIRECTION('center_axis',(-1.22460635382238E-16,-1.,-2.46519032881566E-32));
#24103=DIRECTION('ref_axis',(-3.01888774004913E-48,-2.46519032881566E-32,
1.));
#24104=DIRECTION('',(-1.22460635382238E-16,-1.,-2.46519032881566E-32));
#24105=DIRECTION('',(-1.22460635382238E-16,-1.,-2.46519032881566E-32));
#24106=DIRECTION('center_axis',(-1.22460635382238E-16,-1.,-2.46519032881566E-32));
#24107=DIRECTION('ref_axis',(-3.01888774004913E-48,-2.46519032881566E-32,
1.));
#24108=DIRECTION('',(-1.22460635382238E-16,-1.,-2.46519032881566E-32));
#24109=DIRECTION('',(-1.22460635382238E-16,-1.,-2.46519032881566E-32));
#24110=DIRECTION('center_axis',(-1.22460635382238E-16,-1.,-2.46519032881566E-32));
#24111=DIRECTION('ref_axis',(-3.01888774004913E-48,-2.46519032881566E-32,
1.));
#24112=DIRECTION('',(-1.22460635382238E-16,-1.,-2.46519032881566E-32));
#24113=DIRECTION('',(-1.22460635382238E-16,-1.,-2.46519032881566E-32));
#24114=DIRECTION('center_axis',(-1.22460635382238E-16,-1.,-2.46519032881566E-32));
#24115=DIRECTION('ref_axis',(-3.01888774004913E-48,-2.46519032881566E-32,
1.));
#24116=DIRECTION('',(-1.22460635382238E-16,-1.,-2.46519032881566E-32));
#24117=DIRECTION('',(-1.22460635382238E-16,-1.,-2.46519032881566E-32));
#24118=DIRECTION('center_axis',(-1.22460635382238E-16,-1.,-2.46519032881566E-32));
#24119=DIRECTION('ref_axis',(-3.01888774004913E-48,-2.46519032881566E-32,
1.));
#24120=DIRECTION('',(-1.22460635382238E-16,-1.,-2.46519032881566E-32));
#24121=DIRECTION('',(-1.22460635382238E-16,-1.,-2.46519032881566E-32));
#24122=DIRECTION('center_axis',(-1.22460635382238E-16,-1.,-2.46519032881566E-32));
#24123=DIRECTION('ref_axis',(-3.01888774004913E-48,-2.46519032881566E-32,
1.));
#24124=DIRECTION('',(-1.22460635382238E-16,-1.,-2.46519032881566E-32));
#24125=DIRECTION('',(-1.22460635382238E-16,-1.,-2.46519032881566E-32));
#24126=DIRECTION('center_axis',(-1.22460635382238E-16,-1.,-2.46519032881566E-32));
#24127=DIRECTION('ref_axis',(-3.01888774004913E-48,-2.46519032881566E-32,
1.));
#24128=DIRECTION('',(-1.22460635382238E-16,-1.,-2.46519032881566E-32));
#24129=DIRECTION('',(-1.22460635382238E-16,-1.,-2.46519032881566E-32));
#24130=DIRECTION('center_axis',(-1.22460635382238E-16,-1.,-2.46519032881566E-32));
#24131=DIRECTION('ref_axis',(-3.01888774004913E-48,-2.46519032881566E-32,
1.));
#24132=DIRECTION('',(-1.22460635382238E-16,-1.,-2.46519032881566E-32));
#24133=DIRECTION('',(-1.22460635382238E-16,-1.,-2.46519032881566E-32));
#24134=DIRECTION('center_axis',(-1.22460635382238E-16,-1.,-2.46519032881566E-32));
#24135=DIRECTION('ref_axis',(-3.01888774004913E-48,-2.46519032881566E-32,
1.));
#24136=DIRECTION('',(-1.22460635382238E-16,-1.,-2.46519032881566E-32));
#24137=DIRECTION('',(-1.22460635382238E-16,-1.,-2.46519032881566E-32));
#24138=DIRECTION('center_axis',(-1.22460635382238E-16,-1.,-2.46519032881566E-32));
#24139=DIRECTION('ref_axis',(-3.01888774004913E-48,-2.46519032881566E-32,
1.));
#24140=DIRECTION('',(-1.22460635382238E-16,-1.,-2.46519032881566E-32));
#24141=DIRECTION('',(-1.22460635382238E-16,-1.,-2.46519032881566E-32));
#24142=DIRECTION('center_axis',(-1.22460635382238E-16,-1.,-2.46519032881566E-32));
#24143=DIRECTION('ref_axis',(-3.01888774004913E-48,-2.46519032881566E-32,
1.));
#24144=DIRECTION('',(-1.22460635382238E-16,-1.,-2.46519032881566E-32));
#24145=DIRECTION('',(-1.22460635382238E-16,-1.,-2.46519032881566E-32));
#24146=DIRECTION('center_axis',(-1.22460635382238E-16,-1.,-2.46519032881566E-32));
#24147=DIRECTION('ref_axis',(-3.01888774004913E-48,-2.46519032881566E-32,
1.));
#24148=DIRECTION('',(-1.22460635382238E-16,-1.,-2.46519032881566E-32));
#24149=DIRECTION('',(-1.22460635382238E-16,-1.,-2.46519032881566E-32));
#24150=DIRECTION('center_axis',(-1.22460635382238E-16,-1.,-2.46519032881566E-32));
#24151=DIRECTION('ref_axis',(-3.01888774004913E-48,-2.46519032881566E-32,
1.));
#24152=DIRECTION('',(-1.22460635382238E-16,-1.,-2.46519032881566E-32));
#24153=DIRECTION('',(-1.22460635382238E-16,-1.,-2.46519032881566E-32));
#24154=DIRECTION('center_axis',(-1.22460635382238E-16,-1.,-2.46519032881566E-32));
#24155=DIRECTION('ref_axis',(-3.01888774004913E-48,-2.46519032881566E-32,
1.));
#24156=DIRECTION('',(-1.22460635382238E-16,-1.,-2.46519032881566E-32));
#24157=DIRECTION('',(-1.22460635382238E-16,-1.,-2.46519032881566E-32));
#24158=DIRECTION('center_axis',(-1.22460635382238E-16,-1.,-2.46519032881566E-32));
#24159=DIRECTION('ref_axis',(-3.01888774004913E-48,-2.46519032881566E-32,
1.));
#24160=DIRECTION('',(-1.22460635382238E-16,-1.,-2.46519032881566E-32));
#24161=DIRECTION('',(-1.22460635382238E-16,-1.,-2.46519032881566E-32));
#24162=DIRECTION('center_axis',(-1.22460635382238E-16,-1.,-2.46519032881566E-32));
#24163=DIRECTION('ref_axis',(-3.01888774004913E-48,-2.46519032881566E-32,
1.));
#24164=DIRECTION('',(-1.22460635382238E-16,-1.,-2.46519032881566E-32));
#24165=DIRECTION('',(-1.22460635382238E-16,-1.,-2.46519032881566E-32));
#24166=DIRECTION('center_axis',(-1.22460635382238E-16,-1.,-2.46519032881566E-32));
#24167=DIRECTION('ref_axis',(-3.01888774004913E-48,-2.46519032881566E-32,
1.));
#24168=DIRECTION('',(-1.22460635382238E-16,-1.,-2.46519032881566E-32));
#24169=DIRECTION('',(-1.22460635382238E-16,-1.,-2.46519032881566E-32));
#24170=DIRECTION('center_axis',(-1.22460635382238E-16,-1.,-2.46519032881566E-32));
#24171=DIRECTION('ref_axis',(-3.01888774004913E-48,-2.46519032881566E-32,
1.));
#24172=DIRECTION('',(-1.22460635382238E-16,-1.,-2.46519032881566E-32));
#24173=DIRECTION('',(-1.22460635382238E-16,-1.,-2.46519032881566E-32));
#24174=DIRECTION('center_axis',(-1.22460635382238E-16,-1.,-2.46519032881566E-32));
#24175=DIRECTION('ref_axis',(2.46519032881566E-32,-2.46519032881566E-32,
1.));
#24176=DIRECTION('center_axis',(-1.22460635382238E-16,-1.,-2.46519032881566E-32));
#24177=DIRECTION('ref_axis',(-3.01888774004913E-48,-2.46519032881566E-32,
1.));
#24178=DIRECTION('',(-1.22460635382238E-16,-1.,-2.46519032881566E-32));
#24179=DIRECTION('',(-1.22460635382238E-16,-1.,-2.46519032881566E-32));
#24180=DIRECTION('center_axis',(-1.22460635382238E-16,-1.,-2.46519032881566E-32));
#24181=DIRECTION('ref_axis',(2.46519032881566E-32,-2.46519032881566E-32,
1.));
#24182=DIRECTION('center_axis',(1.22460635382238E-16,1.,2.46519032881566E-32));
#24183=DIRECTION('ref_axis',(-2.46519032881566E-32,2.46519032881566E-32,
-1.));
#24184=DIRECTION('center_axis',(1.22460635382238E-16,1.,2.46519032881566E-32));
#24185=DIRECTION('ref_axis',(-2.46519032881566E-32,2.46519032881566E-32,
-1.));
#24186=DIRECTION('center_axis',(0.499999999999999,-6.12303176911187E-17,
-0.866025403784439));
#24187=DIRECTION('ref_axis',(-0.866025403784439,1.06054021204601E-16,-0.499999999999999));
#24188=DIRECTION('',(-1.22460635382238E-16,-1.,-2.46519032881566E-32));
#24189=DIRECTION('center_axis',(0.500000000000002,-6.12303176911191E-17,
0.866025403784438));
#24190=DIRECTION('ref_axis',(0.866025403784438,-1.06054021204601E-16,-0.500000000000002));
#24191=DIRECTION('center_axis',(0.427747181051069,-5.2382191574475E-17,
-0.903898417468945));
#24192=DIRECTION('ref_axis',(-0.903898417468945,1.10691974524246E-16,-0.427747181051069));
#24193=DIRECTION('',(-1.22460635382238E-16,-1.,-2.46519032881566E-32));
#24194=DIRECTION('center_axis',(0.568925401443124,-6.96709661458196E-17,
0.82238913392188));
#24195=DIRECTION('ref_axis',(0.82238913392188,-1.00710295871522E-16,-0.568925401443124));
#24196=DIRECTION('center_axis',(0.568925401443111,-6.9670966145818E-17,
-0.82238913392189));
#24197=DIRECTION('ref_axis',(-0.82238913392189,1.00710295871523E-16,-0.568925401443111));
#24198=DIRECTION('',(-1.22460635382238E-16,-1.,-2.46519032881566E-32));
#24199=DIRECTION('center_axis',(0.427747181051084,-5.23821915744769E-17,
0.903898417468938));
#24200=DIRECTION('ref_axis',(0.903898417468938,-1.10691974524245E-16,-0.427747181051084));
#24201=DIRECTION('center_axis',(0.634064698205714,-7.76479658157185E-17,
-0.773280000057739));
#24202=DIRECTION('ref_axis',(-0.773280000057739,9.46963601354476E-17,-0.634064698205714));
#24203=DIRECTION('',(-1.22460635382238E-16,-1.,-2.46519032881566E-32));
#24204=DIRECTION('center_axis',(0.352647775185578,-4.31854706153584E-17,
0.935756136317931));
#24205=DIRECTION('ref_axis',(0.935756136317931,-1.14593291016322E-16,-0.352647775185578));
#24206=DIRECTION('center_axis',(0.694984399015069,-8.5108231084128E-17,
-0.719024815375425));
#24207=DIRECTION('ref_axis',(-0.719024815375425,8.80522357464707E-17,-0.694984399015069));
#24208=DIRECTION('',(-1.22460635382238E-16,-1.,-2.46519032881566E-32));
#24209=DIRECTION('center_axis',(0.275201556558999,-3.37013574743959E-17,
0.961386552468623));
#24210=DIRECTION('ref_axis',(0.961386552468623,-1.17732008063247E-16,-0.275201556558999));
#24211=DIRECTION('center_axis',(0.751279093313334,-9.20021151165424E-17,
-0.65998463917753));
#24212=DIRECTION('ref_axis',(-0.65998463917753,8.08221382561973E-17,-0.751279093313334));
#24213=DIRECTION('',(-1.22460635382238E-16,-1.,-2.46519032881566E-32));
#24214=DIRECTION('center_axis',(0.195923916978581,-2.39929673597738E-17,
0.980619099730252));
#24215=DIRECTION('ref_axis',(0.980619099730252,-1.20087238020925E-16,-0.195923916978581));
#24216=DIRECTION('center_axis',(0.802574149197924,-9.82837402521366E-17,
-0.59655237409571));
#24217=DIRECTION('ref_axis',(-0.59655237409571,7.3054182770543E-17,-0.802574149197924));
#24218=DIRECTION('',(-1.22460635382238E-16,-1.,-2.46519032881566E-32));
#24219=DIRECTION('center_axis',(0.115342436055841,-1.41249080059334E-17,
0.99332578867394));
#24220=DIRECTION('ref_axis',(0.99332578867394,-1.21643307222573E-16,-0.115342436055841));
#24221=DIRECTION('center_axis',(0.848528206535016,-1.03911303312029E-16,
-0.529150151388497));
#24222=DIRECTION('ref_axis',(-0.529150151388497,6.48000637516426E-17,-0.848528206535016));
#24223=DIRECTION('',(-1.22460635382238E-16,-1.,-2.46519032881566E-32));
#24224=DIRECTION('center_axis',(0.033993370251312,-4.16284971975936E-18,
0.999422058381221));
#24225=DIRECTION('ref_axis',(0.999422058381221,-1.22389860284388E-16,-0.033993370251312));
#24226=DIRECTION('center_axis',(0.888835448654917,-1.08847353792537E-16,
-0.458226521727423));
#24227=DIRECTION('ref_axis',(-0.458226521727423,5.6114710999733E-17,-0.888835448654917));
#24228=DIRECTION('',(-1.22460635382238E-16,-1.,-2.46519032881566E-32));
#24229=DIRECTION('center_axis',(-0.047581915823728,5.82691164447786E-18,
0.998867339183009));
#24230=DIRECTION('ref_axis',(0.998867339183009,-1.22321929018916E-16,0.047581915823728));
#24231=DIRECTION('center_axis',(0.923227637511546,-1.13059043092106E-16,
-0.384253470166307));
#24232=DIRECTION('ref_axis',(-0.384253470166307,4.70559241043957E-17,-0.923227637511546));
#24233=DIRECTION('',(-1.22460635382238E-16,-1.,-2.46519032881566E-32));
#24234=DIRECTION('center_axis',(-0.128840552099425,1.57778958730938E-17,
0.991665322644044));
#24235=DIRECTION('ref_axis',(0.991665322644044,-1.21439965497521E-16,0.128840552099425));
#24236=DIRECTION('center_axis',(0.951475898762374,-1.16518343113326E-16,
-0.307723275158594));
#24237=DIRECTION('ref_axis',(-0.307723275158594,3.76839877978246E-17,-0.951475898762374));
#24238=DIRECTION('',(-1.22460635382238E-16,-1.,-2.46519032881566E-32));
#24239=DIRECTION('center_axis',(-0.209241775758096,2.56238808078441E-17,
0.977863936996144));
#24240=DIRECTION('ref_axis',(0.977863936996144,-1.19749839041924E-16,0.209241775758096));
#24241=DIRECTION('center_axis',(0.973392244889412,-1.192022327853E-16,-0.229145232525468));
#24242=DIRECTION('ref_axis',(-0.229145232525468,2.80612707698795E-17,-0.973392244889412));
#24243=DIRECTION('',(-1.22460635382238E-16,-1.,-2.46519032881566E-32));
#24244=DIRECTION('center_axis',(-0.288250529921558,3.52993430434607E-17,
0.957555028183728));
#24245=DIRECTION('ref_axis',(0.957555028183729,-1.17262797164836E-16,0.288250529921558));
#24246=DIRECTION('center_axis',(0.988830826225127,-1.21092851265072E-16,
-0.149042266176187));
#24247=DIRECTION('ref_axis',(-0.149042266176187,1.82518106147445E-17,-0.988830826225127));
#24248=DIRECTION('',(-1.22460635382238E-16,-1.,-2.46519032881566E-32));
#24249=DIRECTION('center_axis',(-0.365341024366383,4.47398939751048E-17,
0.930873748644209));
#24250=DIRECTION('ref_axis',(0.930873748644209,-1.13995390719615E-16,0.365341024366383));
#24251=DIRECTION('center_axis',(0.997688901557916,-1.22177616798589E-16,
-0.0679474481357467));
#24252=DIRECTION('ref_axis',(-0.0679474481357467,8.32088767130521E-18,-0.997688901557916));
#24253=DIRECTION('',(-1.22460635382238E-16,-1.,-2.46519032881566E-32));
#24254=DIRECTION('center_axis',(-0.440000234571075,5.38827082939075E-17,
0.89799765789082));
#24255=DIRECTION('ref_axis',(0.89799765789082,-1.09969363757071E-16,0.440000234571075));
#24256=DIRECTION('center_axis',(0.999907521857919,-1.22449310450199E-16,
0.0135995489614973));
#24257=DIRECTION('ref_axis',(0.0135995489614973,-1.66540940673678E-18,-0.999907521857919));
#24258=DIRECTION('',(-1.22460635382238E-16,-1.,-2.46519032881566E-32));
#24259=DIRECTION('center_axis',(-0.511731315809626,6.26669420790353E-17,
0.859145540883353));
#24260=DIRECTION('ref_axis',(0.859145540883353,-1.05211508822392E-16,0.511731315809626));
#24261=DIRECTION('center_axis',(0.995471922573086,-1.21906124143478E-16,
0.0950560433041702));
#24262=DIRECTION('ref_axis',(0.0950560433041702,-1.16406234599502E-17,-0.995471922573086));
#24263=DIRECTION('',(-1.22460635382238E-16,-1.,-2.46519032881566E-32));
#24264=DIRECTION('center_axis',(-0.580056909571188,7.10341377039448E-17,
0.814575952050343));
#24265=DIRECTION('ref_axis',(0.814575952050343,-9.97534886551763E-17,0.580056909571188));
#24266=DIRECTION('center_axis',(0.984411621884836,-1.20551672693676E-16,
0.175879955361797));
#24267=DIRECTION('ref_axis',(0.175879955361797,-2.15383710846052E-17,-0.984411621884836));
#24268=DIRECTION('',(-1.22460635382238E-16,-1.,-2.46519032881566E-32));
#24269=DIRECTION('center_axis',(-0.644522320302207,7.89286128622424E-17,
0.76458549465201));
#24270=DIRECTION('ref_axis',(0.76458549465201,-9.36316254791277E-17,0.644522320302207));
#24271=DIRECTION('center_axis',(0.966800224269427,-1.18394969751724E-16,
0.255533415334641));
#24272=DIRECTION('ref_axis',(0.255533415334641,-3.12927844032734E-17,-0.966800224269427));
#24273=DIRECTION('',(-1.22460635382238E-16,-1.,-2.46519032881566E-32));
#24274=DIRECTION('center_axis',(-0.704698541330313,8.62978311242462E-17,
0.709506846934496));
#24275=DIRECTION('ref_axis',(0.709506846934496,-8.68866592836464E-17,0.704698541330313));
#24276=DIRECTION('center_axis',(0.942754930672314,-1.15450367819869E-16,
0.333486342588479));
#24277=DIRECTION('ref_axis',(0.333486342588479,-4.08389494046837E-17,-0.942754930672314));
#24278=DIRECTION('',(-1.22460635382238E-16,-1.,-2.46519032881566E-32));
#24279=DIRECTION('center_axis',(-0.76018510983294,9.3092751558258E-17,0.649706548211022));
#24280=DIRECTION('ref_axis',(0.649706548211022,-7.95634767059223E-17,0.76018510983294));
#24281=DIRECTION('center_axis',(0.912435758555192,-1.11737462738143E-16,
0.409219973253765));
#24282=DIRECTION('ref_axis',(0.409219973253765,-5.01133379357584E-17,-0.912435758555192));
#24283=DIRECTION('',(-1.22460635382238E-16,-1.,-2.46519032881566E-32));
#24284=DIRECTION('center_axis',(-0.810612771851345,9.92681550898726E-17,
0.585582559603238));
#24285=DIRECTION('ref_axis',(0.585582559603238,-7.17108123177697E-17,0.810612771851345));
#24286=DIRECTION('center_axis',(0.876044477006188,-1.07280963277278E-16,
0.48223031251359));
#24287=DIRECTION('ref_axis',(0.48223031251359,-5.90542304709892E-17,-0.876044477006188));
#24288=DIRECTION('',(-1.22460635382238E-16,-1.,-2.46519032881566E-32));
#24289=DIRECTION('center_axis',(-0.855645939614771,1.04782945427457E-16,
0.517561615675617));
#24290=DIRECTION('ref_axis',(0.517561615675617,-6.33809243050936E-17,0.855645939614771));
#24291=DIRECTION('center_axis',(0.833823263999873,-1.02110526705916E-16,
0.552031488606037));
#24292=DIRECTION('ref_axis',(0.552031488606037,-6.76021268456979E-17,-0.833823263999873));
#24293=DIRECTION('',(-1.22460635382238E-16,-1.,-2.46519032881566E-32));
#24294=DIRECTION('center_axis',(-0.894984924821705,1.0960042255119E-16,
0.44609638458733));
#24295=DIRECTION('ref_axis',(0.446096384587331,-5.46292466982836E-17,0.894984924821705));
#24296=DIRECTION('center_axis',(0.786053094742794,-9.62605614263769E-17,
0.618158986220596));
#24297=DIRECTION('ref_axis',(0.618158986220596,-7.57001422198142E-17,-0.786053094742795));
#24298=DIRECTION('',(-1.22460635382238E-16,-1.,-2.46519032881566E-32));
#24299=DIRECTION('center_axis',(-0.928367933016068,1.13688526945642E-16,
0.371662455660338));
#24300=DIRECTION('ref_axis',(0.371662455660338,-4.55140204678878E-17,0.928367933016068));
#24301=DIRECTION('center_axis',(0.733051871829834,-8.97699979924202E-17,
0.680172737770911));
#24302=DIRECTION('ref_axis',(0.680172737770911,-8.3294385637102E-17,-0.733051871829834));
#24303=DIRECTION('',(-1.22460635382238E-16,-1.,-2.46519032881566E-32));
#24304=DIRECTION('center_axis',(-0.955572805786137,1.17020052950558E-16,
0.294755174410915));
#24305=DIRECTION('ref_axis',(0.294755174410915,-3.6095905940563E-17,0.955572805786137));
#24306=DIRECTION('center_axis',(0.675172309654891,-8.2682030032831E-17,
0.737660051971963));
#24307=DIRECTION('ref_axis',(0.737660051971963,-9.03343186605811E-17,-0.675172309654891));
#24308=DIRECTION('',(-1.22460635382238E-16,-1.,-2.46519032881566E-32));
#24309=DIRECTION('center_axis',(-0.976418499192115,1.19572829810037E-16,
0.215886346106968));
#24310=DIRECTION('ref_axis',(0.215886346106968,-2.6437579114609E-17,0.976418499192115));
#24311=DIRECTION('center_axis',(0.612799587154786,-7.5043826804948E-17,
0.790238360232484));
#24312=DIRECTION('ref_axis',(0.790238360232484,-9.67730916974876E-17,-0.612799587154786));
#24313=DIRECTION('',(-1.22460635382238E-16,-1.,-2.46519032881566E-32));
#24314=DIRECTION('center_axis',(-0.990766288583682,1.21329869215259E-16,
0.135580829788419));
#24315=DIRECTION('ref_axis',(0.135580829788419,-1.66033145615408E-17,0.990766288583682));
#24316=DIRECTION('center_axis',(0.54634878450698,-6.69062192910381E-17,
0.837557762585809));
#24317=DIRECTION('ref_axis',(0.837557762585809,-1.02567855775584E-16,-0.54634878450698));
#24318=DIRECTION('',(-1.22460635382238E-16,-1.,-2.46519032881566E-32));
#24319=DIRECTION('center_axis',(-0.998520691789656,1.22279478358873E-16,
0.0543730454168903));
#24320=DIRECTION('ref_axis',(0.0543730454168903,-6.65855768941968E-18,0.998520691789656));
#24321=DIRECTION('center_axis',(0.476262120839485,-5.83233619264954E-17,
0.879303356216429));
#24322=DIRECTION('ref_axis',(0.879303356216429,-1.07680047695998E-16,-0.476262120839484));
#24323=DIRECTION('',(-1.22460635382238E-16,-1.,-2.46519032881566E-32));
#24324=DIRECTION('center_axis',(-0.999630104536087,1.22415337748702E-16,
-0.0271965826009666));
#24325=DIRECTION('ref_axis',(-0.0271965826009666,3.33051078553986E-18,0.999630104536087));
#24326=DIRECTION('center_axis',(0.40300601133552,-4.93523722110092E-17,
0.915197331086271));
#24327=DIRECTION('ref_axis',(0.915197331086272,-1.12075646664953E-16,-0.40300601133552));
#24328=DIRECTION('',(-1.22460635382238E-16,-1.,-2.46519032881566E-32));
#24329=DIRECTION('center_axis',(-0.994087143864189,1.21736543262923E-16,
-0.108585221848735));
#24330=DIRECTION('ref_axis',(-0.108585221848735,1.32974152607173E-17,0.994087143864189));
#24331=DIRECTION('center_axis',(0.327067963317431,-4.00529506010271E-17,
0.945000818714665));
#24332=DIRECTION('ref_axis',(0.945000818714665,-1.15725400696533E-16,-0.327067963317431));
#24333=DIRECTION('',(-1.22460635382238E-16,-1.,-2.46519032881566E-32));
#24334=DIRECTION('center_axis',(-0.981928697262709,1.20247612166844E-16,
-0.1892512443604));
#24335=DIRECTION('ref_axis',(-0.1892512443604,2.31758276312537E-17,0.981928697262709));
#24336=DIRECTION('center_axis',(0.248953331965879,-3.04869832130668E-17,
0.968515481808673));
#24337=DIRECTION('ref_axis',(0.968515481808673,-1.18605021279824E-16,-0.248953331965879));
#24338=DIRECTION('',(-1.22460635382238E-16,-1.,-2.46519032881566E-32));
#24339=DIRECTION('center_axis',(-0.963235677187776,1.17958453051255E-16,
-0.268657831065104));
#24340=DIRECTION('ref_axis',(-0.268657831065104,3.29000086926465E-17,0.963235677187776));
#24341=DIRECTION('center_axis',(0.169181957264503,-2.07181299818217E-17,
0.985584834165051));
#24342=DIRECTION('ref_axis',(0.985584834165051,-1.2069534501495E-16,-0.169181957264503));
#24343=DIRECTION('',(-1.22460635382238E-16,-1.,-2.46519032881566E-32));
#24344=DIRECTION('center_axis',(-0.938132482603859,1.14884299892385E-16,
-0.346276544229492));
#24345=DIRECTION('ref_axis',(-0.346276544229492,4.24052456243092E-17,0.93813248260386));
#24346=DIRECTION('center_axis',(0.0882847045505903,-1.08114010137985E-17,
0.996095282060112));
#24347=DIRECTION('ref_axis',(0.996095282060113,-1.21982461142331E-16,-0.0882847045505903));
#24348=DIRECTION('',(-1.22460635382238E-16,-1.,-2.46519032881566E-32));
#24349=DIRECTION('center_axis',(-0.906786171129178,1.11045610672306E-16,
-0.421590844123641));
#24350=DIRECTION('ref_axis',(-0.421590844123641,5.1628282642715E-17,0.906786171129178));
#24351=DIRECTION('center_axis',(0.00679993169384408,-8.32723955783986E-19,
0.999976880197217));
#24352=DIRECTION('ref_axis',(0.999976880197217,-1.22457804116499E-16,-0.00679993169384408));
#24353=DIRECTION('',(-1.22460635382238E-16,-1.,-2.46519032881566E-32));
#24354=DIRECTION('center_axis',(-0.86940534729482,1.06467931234439E-16,
-0.49409952650774));
#24355=DIRECTION('ref_axis',(-0.49409952650774,6.05077419582007E-17,0.86940534729482));
#24356=DIRECTION('center_axis',(-0.074730093586415,9.15149474276644E-18,
0.997203797181181));
#24357=DIRECTION('ref_axis',(0.997203797181181,-1.22118210608388E-16,0.074730093586415));
#24358=DIRECTION('',(-1.22460635382238E-16,-1.,-2.46519032881566E-32));
#24359=DIRECTION('center_axis',(-0.826238774316,1.01181725280179E-16,-0.563320058063614));
#24360=DIRECTION('ref_axis',(-0.563320058063614,6.89845322340292E-17,0.826238774316));
#24361=DIRECTION('center_axis',(-0.155762802423454,1.90748117536942E-17,
0.98779448742195));
#24362=DIRECTION('ref_axis',(0.98779448742195,-1.20965940556764E-16,0.155762802423454));
#24363=DIRECTION('',(-1.22460635382238E-16,-1.,-2.46519032881566E-32));
#24364=DIRECTION('center_axis',(-0.777573718613909,9.52221716379887E-17,
-0.628791787574343));
#24365=DIRECTION('ref_axis',(-0.628791787574343,7.7002241829487E-17,0.777573718613909));
#24366=DIRECTION('center_axis',(-0.235758935509419,2.88711890395234E-17,
0.971811568323544));
#24367=DIRECTION('ref_axis',(0.971811568323544,-1.1900866212871E-16,0.235758935509419));
#24368=DIRECTION('',(-1.22460635382238E-16,-1.,-2.46519032881566E-32));
#24369=DIRECTION('center_axis',(-0.723734038105076,8.86289301541003E-17,
-0.690079011482106));
#24370=DIRECTION('ref_axis',(-0.690079011482105,8.45075142100451E-17,0.723734038105076));
#24371=DIRECTION('center_axis',(-0.314186131777054,3.84754333257055E-17,
0.949361403575568));
#24372=DIRECTION('ref_axis',(0.949361403575568,-1.16259400689237E-16,0.314186131777054));
#24373=DIRECTION('',(-1.22460635382238E-16,-1.,-2.46519032881566E-32));
#24374=DIRECTION('center_axis',(-0.665078026980365,8.14458777627806E-17,
-0.746773873423478));
#24375=DIRECTION('ref_axis',(-0.746773873423478,9.14504030262939E-17,0.665078026980365));
#24376=DIRECTION('center_axis',(-0.390522471174776,4.78236299511047E-17,
0.920593395320402));
#24377=DIRECTION('ref_axis',(0.920593395320402,-1.12736452119628E-16,0.390522471174777));
#24378=DIRECTION('',(-1.22460635382238E-16,-1.,-2.46519032881566E-32));
#24379=DIRECTION('center_axis',(-0.60199603131625,7.37208164925735E-17,
-0.798499078446234));
#24380=DIRECTION('ref_axis',(-0.798499078446233,9.7784704498657E-17,0.60199603131625));
#24381=DIRECTION('center_axis',(-0.464259947958503,5.68535682095229E-17,
0.885698989906598));
#24382=DIRECTION('ref_axis',(0.885698989906598,-1.08463261061368E-16,0.464259947958503));
#24383=DIRECTION('',(-1.22460635382238E-16,-1.,-2.46519032881566E-32));
#24384=DIRECTION('center_axis',(-0.53490785138608,6.55051553516869E-17,
-0.844910403845004));
#24385=DIRECTION('ref_axis',(-0.844910403845004,1.03468264895922E-16,0.53490785138608));
#24386=DIRECTION('center_axis',(-0.534907851386066,6.55051553516852E-17,
0.844910403845013));
#24387=DIRECTION('ref_axis',(0.844910403845013,-1.03468264895923E-16,0.534907851386066));
#24388=DIRECTION('',(-1.22460635382238E-16,-1.,-2.46519032881566E-32));
#24389=DIRECTION('center_axis',(-0.464259947958518,5.68535682095247E-17,
-0.88569898990659));
#24390=DIRECTION('ref_axis',(-0.88569898990659,1.08463261061367E-16,0.464259947958518));
#24391=DIRECTION('center_axis',(-0.601996031316237,7.37208164925719E-17,
0.798499078446243));
#24392=DIRECTION('ref_axis',(0.798499078446244,-9.77847044986583E-17,0.601996031316237));
#24393=DIRECTION('',(-1.22460635382238E-16,-1.,-2.46519032881566E-32));
#24394=DIRECTION('center_axis',(-0.390522471174792,4.78236299511067E-17,
-0.920593395320395));
#24395=DIRECTION('ref_axis',(-0.920593395320395,1.12736452119627E-16,0.390522471174792));
#24396=DIRECTION('center_axis',(-0.665078026980353,8.1445877762779E-17,
0.746773873423489));
#24397=DIRECTION('ref_axis',(0.746773873423489,-9.14504030262952E-17,0.665078026980353));
#24398=DIRECTION('',(-1.22460635382238E-16,-1.,-2.46519032881566E-32));
#24399=DIRECTION('center_axis',(-0.31418613177707,3.84754333257075E-17,
-0.949361403575562));
#24400=DIRECTION('ref_axis',(-0.949361403575562,1.16259400689236E-16,0.31418613177707));
#24401=DIRECTION('center_axis',(-0.723734038105065,8.86289301540989E-17,
0.690079011482118));
#24402=DIRECTION('ref_axis',(0.690079011482118,-8.45075142100467E-17,0.723734038105065));
#24403=DIRECTION('',(-1.22460635382238E-16,-1.,-2.46519032881566E-32));
#24404=DIRECTION('center_axis',(-0.235758935509435,2.88711890395255E-17,
-0.97181156832354));
#24405=DIRECTION('ref_axis',(-0.97181156832354,1.1900866212871E-16,0.235758935509435));
#24406=DIRECTION('center_axis',(-0.777573718613899,9.52221716379874E-17,
0.628791787574355));
#24407=DIRECTION('ref_axis',(0.628791787574355,-7.70022418294886E-17,0.777573718613899));
#24408=DIRECTION('',(-1.22460635382238E-16,-1.,-2.46519032881566E-32));
#24409=DIRECTION('center_axis',(-0.15576280242347,1.90748117536962E-17,
-0.987794487421947));
#24410=DIRECTION('ref_axis',(-0.987794487421947,1.20965940556763E-16,0.15576280242347));
#24411=DIRECTION('center_axis',(-0.826238774315991,1.01181725280178E-16,
0.563320058063628));
#24412=DIRECTION('ref_axis',(0.563320058063628,-6.89845322340309E-17,0.826238774315991));
#24413=DIRECTION('',(-1.22460635382238E-16,-1.,-2.46519032881566E-32));
#24414=DIRECTION('center_axis',(-0.0747300935864316,9.15149474276852E-18,
-0.99720379718118));
#24415=DIRECTION('ref_axis',(-0.99720379718118,1.22118210608387E-16,0.0747300935864316));
#24416=DIRECTION('center_axis',(-0.869405347294812,1.06467931234438E-16,
0.494099526507755));
#24417=DIRECTION('ref_axis',(0.494099526507755,-6.05077419582025E-17,0.869405347294812));
#24418=DIRECTION('',(-1.22460635382238E-16,-1.,-2.46519032881566E-32));
#24419=DIRECTION('center_axis',(0.00679993169382737,-8.32723955781891E-19,
-0.999976880197217));
#24420=DIRECTION('ref_axis',(-0.999976880197217,1.22457804116499E-16,-0.00679993169382737));
#24421=DIRECTION('center_axis',(-0.906786171129171,1.11045610672305E-16,
0.421590844123656));
#24422=DIRECTION('ref_axis',(0.421590844123656,-5.16282826427169E-17,0.906786171129171));
#24423=DIRECTION('',(-1.22460635382238E-16,-1.,-2.46519032881566E-32));
#24424=DIRECTION('center_axis',(0.0882847045505736,-1.08114010137964E-17,
-0.996095282060114));
#24425=DIRECTION('ref_axis',(-0.996095282060114,1.21982461142331E-16,-0.0882847045505736));
#24426=DIRECTION('center_axis',(-0.938132482603854,1.14884299892384E-16,
0.346276544229508));
#24427=DIRECTION('ref_axis',(0.346276544229508,-4.24052456243111E-17,0.938132482603854));
#24428=DIRECTION('',(-1.22460635382238E-16,-1.,-2.46519032881566E-32));
#24429=DIRECTION('center_axis',(0.169181957264487,-2.07181299818196E-17,
-0.985584834165054));
#24430=DIRECTION('ref_axis',(-0.985584834165054,1.2069534501495E-16,-0.169181957264487));
#24431=DIRECTION('center_axis',(-0.963235677187772,1.17958453051255E-16,
0.26865783106512));
#24432=DIRECTION('ref_axis',(0.26865783106512,-3.29000086926485E-17,0.963235677187772));
#24433=DIRECTION('',(-1.22460635382238E-16,-1.,-2.46519032881566E-32));
#24434=DIRECTION('center_axis',(0.248953331965864,-3.04869832130648E-17,
-0.968515481808677));
#24435=DIRECTION('ref_axis',(-0.968515481808677,1.18605021279825E-16,-0.248953331965864));
#24436=DIRECTION('center_axis',(-0.981928697262705,1.20247612166844E-16,
0.189251244360416));
#24437=DIRECTION('ref_axis',(0.189251244360416,-2.31758276312558E-17,0.981928697262706));
#24438=DIRECTION('',(-1.22460635382238E-16,-1.,-2.46519032881566E-32));
#24439=DIRECTION('center_axis',(0.327067963317415,-4.00529506010251E-17,
-0.945000818714671));
#24440=DIRECTION('ref_axis',(-0.945000818714671,1.15725400696533E-16,-0.327067963317415));
#24441=DIRECTION('center_axis',(-0.994087143864187,1.21736543262922E-16,
0.108585221848752));
#24442=DIRECTION('ref_axis',(0.108585221848752,-1.32974152607194E-17,0.994087143864187));
#24443=DIRECTION('',(-1.22460635382238E-16,-1.,-2.46519032881566E-32));
#24444=DIRECTION('center_axis',(0.403006011335506,-4.93523722110073E-17,
-0.915197331086278));
#24445=DIRECTION('ref_axis',(-0.915197331086278,1.12075646664954E-16,-0.403006011335505));
#24446=DIRECTION('center_axis',(-0.999630104536087,1.22415337748702E-16,
0.0271965826009838));
#24447=DIRECTION('ref_axis',(0.0271965826009838,-3.33051078554201E-18,0.999630104536087));
#24448=DIRECTION('',(-1.22460635382238E-16,-1.,-2.46519032881566E-32));
#24449=DIRECTION('center_axis',(0.476262120839469,-5.83233619264935E-17,
-0.879303356216437));
#24450=DIRECTION('ref_axis',(-0.879303356216437,1.07680047695999E-16,-0.476262120839469));
#24451=DIRECTION('center_axis',(-0.998520691789657,1.22279478358873E-16,
-0.0543730454168737));
#24452=DIRECTION('ref_axis',(-0.0543730454168737,6.65855768941759E-18,0.998520691789657));
#24453=DIRECTION('',(-1.22460635382238E-16,-1.,-2.46519032881566E-32));
#24454=DIRECTION('center_axis',(0.546348784506966,-6.69062192910363E-17,
-0.837557762585818));
#24455=DIRECTION('ref_axis',(-0.837557762585818,1.02567855775585E-16,-0.546348784506966));
#24456=DIRECTION('center_axis',(-0.990766288583684,1.2132986921526E-16,
-0.135580829788402));
#24457=DIRECTION('ref_axis',(-0.135580829788402,1.66033145615388E-17,0.990766288583684));
#24458=DIRECTION('',(-1.22460635382238E-16,-1.,-2.46519032881566E-32));
#24459=DIRECTION('center_axis',(0.612799587154772,-7.50438268049464E-17,
-0.790238360232494));
#24460=DIRECTION('ref_axis',(-0.790238360232494,9.67730916974889E-17,-0.612799587154772));
#24461=DIRECTION('center_axis',(-0.976418499192119,1.19572829810038E-16,
-0.215886346106952));
#24462=DIRECTION('ref_axis',(-0.215886346106952,2.6437579114607E-17,0.976418499192119));
#24463=DIRECTION('',(-1.22460635382238E-16,-1.,-2.46519032881566E-32));
#24464=DIRECTION('center_axis',(0.675172309654879,-8.26820300328295E-17,
-0.737660051971974));
#24465=DIRECTION('ref_axis',(-0.737660051971974,9.03343186605825E-17,-0.675172309654879));
#24466=DIRECTION('center_axis',(-0.955572805786142,1.17020052950559E-16,
-0.294755174410899));
#24467=DIRECTION('ref_axis',(-0.294755174410899,3.6095905940561E-17,0.955572805786142));
#24468=DIRECTION('',(-1.22460635382238E-16,-1.,-2.46519032881566E-32));
#24469=DIRECTION('center_axis',(0.733051871829822,-8.97699979924187E-17,
-0.680172737770924));
#24470=DIRECTION('ref_axis',(-0.680172737770924,8.32943856371034E-17,-0.733051871829822));
#24471=DIRECTION('center_axis',(-0.928367933016075,1.13688526945643E-16,
-0.371662455660323));
#24472=DIRECTION('ref_axis',(-0.371662455660323,4.55140204678859E-17,0.928367933016075));
#24473=DIRECTION('',(-1.22460635382238E-16,-1.,-2.46519032881566E-32));
#24474=DIRECTION('center_axis',(0.786053094742784,-9.62605614263756E-17,
-0.618158986220609));
#24475=DIRECTION('ref_axis',(-0.618158986220609,7.57001422198158E-17,-0.786053094742784));
#24476=DIRECTION('center_axis',(-0.894984924821712,1.09600422551191E-16,
-0.446096384587316));
#24477=DIRECTION('ref_axis',(-0.446096384587316,5.46292466982817E-17,0.894984924821712));
#24478=DIRECTION('',(-1.22460635382238E-16,-1.,-2.46519032881566E-32));
#24479=DIRECTION('center_axis',(0.833823263999864,-1.02110526705915E-16,
-0.552031488606051));
#24480=DIRECTION('ref_axis',(-0.552031488606051,6.76021268456996E-17,-0.833823263999864));
#24481=DIRECTION('center_axis',(-0.85564593961478,1.04782945427458E-16,
-0.517561615675603));
#24482=DIRECTION('ref_axis',(-0.517561615675603,6.33809243050919E-17,0.85564593961478));
#24483=DIRECTION('',(-1.22460635382238E-16,-1.,-2.46519032881566E-32));
#24484=DIRECTION('center_axis',(0.87604447700618,-1.07280963277277E-16,
-0.482230312513604));
#24485=DIRECTION('ref_axis',(-0.482230312513604,5.9054230470991E-17,-0.87604447700618));
#24486=DIRECTION('center_axis',(-0.810612771851354,9.92681550898737E-17,
-0.585582559603225));
#24487=DIRECTION('ref_axis',(-0.585582559603225,7.1710812317768E-17,0.810612771851354));
#24488=DIRECTION('',(-1.22460635382238E-16,-1.,-2.46519032881566E-32));
#24489=DIRECTION('center_axis',(0.912435758555185,-1.11737462738142E-16,
-0.40921997325378));
#24490=DIRECTION('ref_axis',(-0.40921997325378,5.01133379357602E-17,-0.912435758555185));
#24491=DIRECTION('center_axis',(-0.760185109832951,9.30927515582594E-17,
-0.649706548211009));
#24492=DIRECTION('ref_axis',(-0.649706548211009,7.95634767059206E-17,0.760185109832951));
#24493=DIRECTION('',(-1.22460635382238E-16,-1.,-2.46519032881566E-32));
#24494=DIRECTION('center_axis',(0.942754930672308,-1.15450367819868E-16,
-0.333486342588495));
#24495=DIRECTION('ref_axis',(-0.333486342588495,4.08389494046857E-17,-0.942754930672308));
#24496=DIRECTION('center_axis',(-0.704698541330324,8.62978311242476E-17,
-0.709506846934484));
#24497=DIRECTION('ref_axis',(-0.709506846934484,8.6886659283645E-17,0.704698541330324));
#24498=DIRECTION('',(-1.22460635382238E-16,-1.,-2.46519032881566E-32));
#24499=DIRECTION('center_axis',(0.966800224269422,-1.18394969751723E-16,
-0.255533415334658));
#24500=DIRECTION('ref_axis',(-0.255533415334658,3.12927844032754E-17,-0.966800224269422));
#24501=DIRECTION('center_axis',(-0.64452232030222,7.8928612862244E-17,-0.764585494652));
#24502=DIRECTION('ref_axis',(-0.764585494652,9.36316254791264E-17,0.64452232030222));
#24503=DIRECTION('',(-1.22460635382238E-16,-1.,-2.46519032881566E-32));
#24504=DIRECTION('center_axis',(0.984411621884833,-1.20551672693676E-16,
-0.175879955361814));
#24505=DIRECTION('ref_axis',(-0.175879955361814,2.15383710846073E-17,-0.984411621884833));
#24506=DIRECTION('center_axis',(-0.580056909571201,7.10341377039466E-17,
-0.814575952050334));
#24507=DIRECTION('ref_axis',(-0.814575952050334,9.9753488655175E-17,0.580056909571201));
#24508=DIRECTION('',(-1.22460635382238E-16,-1.,-2.46519032881566E-32));
#24509=DIRECTION('center_axis',(0.995471922573084,-1.21906124143478E-16,
-0.0950560433041868));
#24510=DIRECTION('ref_axis',(-0.0950560433041868,1.16406234599522E-17,-0.995471922573084));
#24511=DIRECTION('center_axis',(-0.51173131580964,6.26669420790371E-17,
-0.859145540883344));
#24512=DIRECTION('ref_axis',(-0.859145540883344,1.05211508822391E-16,0.51173131580964));
#24513=DIRECTION('',(-1.22460635382238E-16,-1.,-2.46519032881566E-32));
#24514=DIRECTION('center_axis',(0.999907521857918,-1.22449310450199E-16,
-0.013599548961514));
#24515=DIRECTION('ref_axis',(-0.013599548961514,1.66540940673888E-18,-0.999907521857918));
#24516=DIRECTION('center_axis',(-0.44000023457109,5.38827082939094E-17,
-0.897997657890813));
#24517=DIRECTION('ref_axis',(-0.897997657890813,1.0996936375707E-16,0.44000023457109));
#24518=DIRECTION('',(-1.22460635382238E-16,-1.,-2.46519032881566E-32));
#24519=DIRECTION('center_axis',(0.997688901557917,-1.22177616798589E-16,
0.0679474481357302));
#24520=DIRECTION('ref_axis',(0.0679474481357302,-8.32088767130315E-18,-0.997688901557917));
#24521=DIRECTION('center_axis',(-0.365341024366398,4.47398939751067E-17,
-0.930873748644203));
#24522=DIRECTION('ref_axis',(-0.930873748644203,1.13995390719615E-16,0.365341024366398));
#24523=DIRECTION('',(-1.22460635382238E-16,-1.,-2.46519032881566E-32));
#24524=DIRECTION('center_axis',(0.988830826225129,-1.21092851265072E-16,
0.149042266176171));
#24525=DIRECTION('ref_axis',(0.149042266176171,-1.82518106147425E-17,-0.988830826225129));
#24526=DIRECTION('center_axis',(-0.288250529921574,3.52993430434627E-17,
-0.957555028183724));
#24527=DIRECTION('ref_axis',(-0.957555028183724,1.17262797164835E-16,0.288250529921574));
#24528=DIRECTION('',(-1.22460635382238E-16,-1.,-2.46519032881566E-32));
#24529=DIRECTION('center_axis',(0.973392244889416,-1.19202232785301E-16,
0.229145232525452));
#24530=DIRECTION('ref_axis',(0.229145232525452,-2.80612707698774E-17,-0.973392244889416));
#24531=DIRECTION('center_axis',(-0.209241775758112,2.56238808078461E-17,
-0.977863936996141));
#24532=DIRECTION('ref_axis',(-0.977863936996141,1.19749839041924E-16,0.209241775758112));
#24533=DIRECTION('',(-1.22460635382238E-16,-1.,-2.46519032881566E-32));
#24534=DIRECTION('center_axis',(0.951475898762379,-1.16518343113327E-16,
0.307723275158579));
#24535=DIRECTION('ref_axis',(0.307723275158579,-3.76839877978227E-17,-0.951475898762379));
#24536=DIRECTION('center_axis',(-0.128840552099442,1.5777895873096E-17,
-0.991665322644042));
#24537=DIRECTION('ref_axis',(-0.991665322644042,1.21439965497521E-16,0.128840552099442));
#24538=DIRECTION('',(-1.22460635382238E-16,-1.,-2.46519032881566E-32));
#24539=DIRECTION('center_axis',(0.923227637511553,-1.13059043092107E-16,
0.384253470166292));
#24540=DIRECTION('ref_axis',(0.384253470166292,-4.70559241043938E-17,-0.923227637511553));
#24541=DIRECTION('center_axis',(-0.0475819158237449,5.82691164447997E-18,
-0.998867339183008));
#24542=DIRECTION('ref_axis',(-0.998867339183008,1.22321929018916E-16,0.0475819158237449));
#24543=DIRECTION('',(-1.22460635382238E-16,-1.,-2.46519032881566E-32));
#24544=DIRECTION('center_axis',(0.888835448654925,-1.08847353792538E-16,
0.458226521727408));
#24545=DIRECTION('ref_axis',(0.458226521727408,-5.61147109997311E-17,-0.888835448654925));
#24546=DIRECTION('center_axis',(0.0339933702512953,-4.16284971975726E-18,
-0.999422058381222));
#24547=DIRECTION('ref_axis',(-0.999422058381222,1.22389860284388E-16,-0.0339933702512953));
#24548=DIRECTION('',(-1.22460635382238E-16,-1.,-2.46519032881566E-32));
#24549=DIRECTION('center_axis',(0.848528206535025,-1.0391130331203E-16,
0.529150151388483));
#24550=DIRECTION('ref_axis',(0.529150151388483,-6.48000637516409E-17,-0.848528206535025));
#24551=DIRECTION('center_axis',(0.115342436055824,-1.41249080059314E-17,
-0.993325788673942));
#24552=DIRECTION('ref_axis',(-0.993325788673942,1.21643307222573E-16,-0.115342436055824));
#24553=DIRECTION('',(-1.22460635382238E-16,-1.,-2.46519032881566E-32));
#24554=DIRECTION('center_axis',(0.802574149197934,-9.82837402521379E-17,
0.596552374095697));
#24555=DIRECTION('ref_axis',(0.596552374095697,-7.30541827705414E-17,-0.802574149197934));
#24556=DIRECTION('center_axis',(0.195923916978565,-2.39929673597718E-17,
-0.980619099730256));
#24557=DIRECTION('ref_axis',(-0.980619099730256,1.20087238020925E-16,-0.195923916978565));
#24558=DIRECTION('',(-1.22460635382238E-16,-1.,-2.46519032881566E-32));
#24559=DIRECTION('center_axis',(0.751279093313345,-9.20021151165437E-17,
0.659984639177518));
#24560=DIRECTION('ref_axis',(0.659984639177518,-8.08221382561957E-17,-0.751279093313345));
#24561=DIRECTION('center_axis',(0.275201556558983,-3.37013574743939E-17,
-0.961386552468627));
#24562=DIRECTION('ref_axis',(-0.961386552468627,1.17732008063247E-16,-0.275201556558983));
#24563=DIRECTION('',(-1.22460635382238E-16,-1.,-2.46519032881566E-32));
#24564=DIRECTION('center_axis',(0.694984399015081,-8.51082310841295E-17,
0.719024815375413));
#24565=DIRECTION('ref_axis',(0.719024815375413,-8.80522357464692E-17,-0.694984399015081));
#24566=DIRECTION('center_axis',(0.352647775185563,-4.31854706153565E-17,
-0.935756136317937));
#24567=DIRECTION('ref_axis',(-0.935756136317937,1.14593291016322E-16,-0.352647775185563));
#24568=DIRECTION('',(-1.22460635382238E-16,-1.,-2.46519032881566E-32));
#24569=DIRECTION('center_axis',(0.634064698205726,-7.76479658157201E-17,
0.773280000057729));
#24570=DIRECTION('ref_axis',(0.773280000057729,-9.46963601354463E-17,-0.634064698205726));
#33359=CARTESIAN_POINT('',(0.,0.,0.));
#33360=CARTESIAN_POINT('Origin',(16.1460502915689,43.6543320991532,35.0294657090004));
#33361=CARTESIAN_POINT('',(16.1460502915689,43.6543320991532,33.0294657090004));
#33362=CARTESIAN_POINT('Origin',(16.1460502915689,43.6543320991532,35.0294657090004));
#33363=CARTESIAN_POINT('',(16.1460502915689,43.9543320991532,32.7294657090004));
#33364=CARTESIAN_POINT('',(16.1460502915689,43.6543320991532,33.0294657090004));
#33365=CARTESIAN_POINT('Origin',(16.1460502915689,43.9543320991532,35.0294657090004));
#33366=CARTESIAN_POINT('Origin',(43.4397894030341,37.9543320991532,35.0294657090004));
#33367=CARTESIAN_POINT('',(44.9397894030341,37.9543320991532,34.7294657090003));
#33368=CARTESIAN_POINT('',(41.9397894030341,37.9543320991532,34.7294657090003));
#33369=CARTESIAN_POINT('Origin',(43.4397894030341,37.9543320991532,34.7294657090003));
#33370=CARTESIAN_POINT('Origin',(43.4397894030341,37.9543320991532,34.7294657090003));
#33371=CARTESIAN_POINT('',(41.6397894030341,37.9543320991532,35.0294657090004));
#33372=CARTESIAN_POINT('',(41.6397894030341,37.9543320991532,35.0294657090004));
#33373=CARTESIAN_POINT('Origin',(43.4397894030341,37.9543320991532,35.0294657090004));
#33374=CARTESIAN_POINT('Origin',(54.9397894030341,37.9543320991532,35.0294657090004));
#33375=CARTESIAN_POINT('',(56.9397894030341,37.9543320991532,34.7294657090004));
#33376=CARTESIAN_POINT('',(52.9397894030341,37.9543320991532,34.7294657090004));
#33377=CARTESIAN_POINT('Origin',(54.9397894030341,37.9543320991532,34.7294657090004));
#33378=CARTESIAN_POINT('Origin',(54.9397894030341,37.9543320991532,34.7294657090004));
#33379=CARTESIAN_POINT('',(52.6397894030341,37.9543320991532,35.0294657090004));
#33380=CARTESIAN_POINT('',(52.6397894030341,37.9543320991532,35.0294657090004));
#33381=CARTESIAN_POINT('Origin',(54.9397894030341,37.9543320991532,35.0294657090004));
#33382=CARTESIAN_POINT('Origin',(35.9397894030341,41.6543320991532,38.5294657090004));
#33383=CARTESIAN_POINT('',(35.9397894030341,41.6543320991532,37.3294657090004));
#33384=CARTESIAN_POINT('Origin',(35.9397894030341,41.6543320991532,38.5294657090004));
#33385=CARTESIAN_POINT('',(35.9397894030341,41.9543320991532,37.0294657090003));
#33386=CARTESIAN_POINT('',(35.9397894030341,41.6543320991532,37.3294657090004));
#33387=CARTESIAN_POINT('Origin',(35.9397894030341,41.9543320991532,38.5294657090004));
#33388=CARTESIAN_POINT('Origin',(20.9397894030341,36.0543320991532,41.0294657090004));
#33389=CARTESIAN_POINT('',(17.9535710587063,37.2043320991532,40.7294657090004));
#33390=CARTESIAN_POINT('',(19.1460502915689,38.7043320991532,40.7294657090004));
#33391=CARTESIAN_POINT('Origin',(20.9397894030341,36.0543320991532,40.7294657090004));
#33392=CARTESIAN_POINT('',(17.634112467821,37.2043320991532,41.0294657090004));
#33393=CARTESIAN_POINT('Ctrl Pts',(17.6341124678211,37.2043320991532,41.0294657090003));
#33394=CARTESIAN_POINT('Ctrl Pts',(17.8009938212686,37.2043320991532,40.8718497544264));
#33395=CARTESIAN_POINT('Ctrl Pts',(17.9535710587063,37.2043320991532,40.7294657090004));
#33396=CARTESIAN_POINT('',(18.6534167299994,38.7043320991532,41.0294657090004));
#33397=CARTESIAN_POINT('Origin',(20.9397894030341,36.0543320991532,41.0294657090004));
#33398=CARTESIAN_POINT('Ctrl Pts',(19.1460502915689,38.7043320991532,40.7294657090004));
#33399=CARTESIAN_POINT('Ctrl Pts',(18.9107626203695,38.7043320991532,40.8613546772117));
#33400=CARTESIAN_POINT('Ctrl Pts',(18.6534167299948,38.7043320991532,41.0294657090034));
#33401=CARTESIAN_POINT('Origin',(35.9397894030341,33.9543320991532,38.5294657090004));
#33402=CARTESIAN_POINT('',(35.9397894030341,34.2543320991532,37.3294657090004));
#33403=CARTESIAN_POINT('',(35.9397894030341,34.2543320991532,39.7294657090004));
#33404=CARTESIAN_POINT('Origin',(35.9397894030341,34.2543320991532,38.5294657090004));
#33405=CARTESIAN_POINT('Origin',(35.9397894030341,34.2543320991532,38.5294657090004));
#33406=CARTESIAN_POINT('',(35.9397894030341,33.9543320991532,40.0294657090004));
#33407=CARTESIAN_POINT('',(35.9397894030341,33.9543320991532,40.0294657090004));
#33408=CARTESIAN_POINT('Origin',(35.9397894030341,33.9543320991532,38.5294657090004));
#33409=CARTESIAN_POINT('Origin',(16.1460502915689,31.9543320991532,35.0294657090004));
#33410=CARTESIAN_POINT('',(16.1460502915689,32.2543320991532,33.0294657090004));
#33411=CARTESIAN_POINT('',(16.1460502915689,32.2543320991532,37.0294657090004));
#33412=CARTESIAN_POINT('Origin',(16.1460502915689,32.2543320991532,35.0294657090004));
#33413=CARTESIAN_POINT('Origin',(16.1460502915689,32.2543320991532,35.0294657090004));
#33414=CARTESIAN_POINT('',(16.1460502915689,31.9543320991532,37.3294657090004));
#33415=CARTESIAN_POINT('',(16.1460502915689,31.9543320991532,37.3294657090004));
#33416=CARTESIAN_POINT('Origin',(16.1460502915689,31.9543320991532,35.0294657090004));
#33417=CARTESIAN_POINT('Origin',(54.9397894030341,37.9543320991532,29.3294657090003));
#33418=CARTESIAN_POINT('',(56.9397894030341,37.9543320991532,29.3294657090003));
#33419=CARTESIAN_POINT('Origin',(54.9397894030341,37.9543320991532,29.3294657090003));
#33420=CARTESIAN_POINT('',(57.2397894030341,37.9543320991532,29.0294657090004));
#33421=CARTESIAN_POINT('',(56.9397894030341,37.9543320991532,29.3294657090003));
#33422=CARTESIAN_POINT('Origin',(54.9397894030341,37.9543320991532,29.0294657090004));
#33423=CARTESIAN_POINT('Origin',(43.4397894030341,37.9543320991532,29.3294657090004));
#33424=CARTESIAN_POINT('',(44.9397894030341,37.9543320991532,29.3294657090004));
#33425=CARTESIAN_POINT('Origin',(43.4397894030341,37.9543320991532,29.3294657090004));
#33426=CARTESIAN_POINT('',(45.2397894030341,37.9543320991532,29.0294657090004));
#33427=CARTESIAN_POINT('',(44.9397894030341,37.9543320991532,29.3294657090004));
#33428=CARTESIAN_POINT('Origin',(43.4397894030341,37.9543320991532,29.0294657090004));
#33429=CARTESIAN_POINT('Origin',(20.9397894030341,36.0543320991532,29.3294657090004));
#33430=CARTESIAN_POINT('',(19.1460502915689,38.7043320991532,29.3294657090004));
#33431=CARTESIAN_POINT('',(17.9535710587063,37.2043320991532,29.3294657090004));
#33432=CARTESIAN_POINT('Origin',(20.9397894030341,36.0543320991532,29.3294657090004));
#33433=CARTESIAN_POINT('',(18.6534167299994,38.7043320991532,29.0294657090004));
#33434=CARTESIAN_POINT('Ctrl Pts',(18.6534167299948,38.7043320991532,29.0294657089973));
#33435=CARTESIAN_POINT('Ctrl Pts',(18.9107626203694,38.7043320991532,29.1975767407891));
#33436=CARTESIAN_POINT('Ctrl Pts',(19.1460502915689,38.7043320991532,29.3294657090004));
#33437=CARTESIAN_POINT('',(17.634112467821,37.2043320991532,29.0294657090004));
#33438=CARTESIAN_POINT('Origin',(20.9397894030341,36.0543320991532,29.0294657090004));
#33439=CARTESIAN_POINT('Ctrl Pts',(17.9535710587063,37.2043320991532,29.3294657090003));
#33440=CARTESIAN_POINT('Ctrl Pts',(17.8009938212686,37.2043320991532,29.1870816635743));
#33441=CARTESIAN_POINT('Ctrl Pts',(17.6341124678211,37.2043320991532,29.0294657090004));
#33442=CARTESIAN_POINT('Origin',(16.1460502915689,31.9543320991532,35.0294657090004));
#33443=CARTESIAN_POINT('',(16.1460502915689,37.2043320991532,33.0294657090004));
#33444=CARTESIAN_POINT('',(16.1460502915689,31.9543320991532,33.0294657090004));
#33445=CARTESIAN_POINT('',(17.9535710587063,37.2043320991532,35.8855432033705));
#33446=CARTESIAN_POINT('Origin',(16.1460502915689,37.2043320991532,35.0294657090004));
#33447=CARTESIAN_POINT('',(17.9535710587063,37.2043320991532,34.1733882146302));
#33448=CARTESIAN_POINT('Ctrl Pts',(17.9535710587063,37.2043320991532,35.8855432033705));
#33449=CARTESIAN_POINT('Ctrl Pts',(17.9192709480126,37.1152646037045,35.9579644068266));
#33450=CARTESIAN_POINT('Ctrl Pts',(17.8836292597541,37.0084958974654,36.0212420504143));
#33451=CARTESIAN_POINT('Ctrl Pts',(17.7876418033145,36.6624002842562,36.1795322193216));
#33452=CARTESIAN_POINT('Ctrl Pts',(17.7397894030341,36.3346151799028,36.2377685040754));
#33453=CARTESIAN_POINT('Ctrl Pts',(17.7397894030341,35.7740490184036,36.2377685040754));
#33454=CARTESIAN_POINT('Ctrl Pts',(17.7876418033145,35.4462639140502,36.1795322193216));
#33455=CARTESIAN_POINT('Ctrl Pts',(17.8925030363182,35.0681727125076,36.0066085592971));
#33456=CARTESIAN_POINT('Ctrl Pts',(17.9435339040124,34.9253475867885,35.9130653773292));
#33457=CARTESIAN_POINT('Ctrl Pts',(18.0267768582634,34.7255600011841,35.7177393279079));
#33458=CARTESIAN_POINT('Ctrl Pts',(18.069284710185,34.6385464913584,35.5957227639568));
#33459=CARTESIAN_POINT('Ctrl Pts',(18.1292923320046,34.522878497267,35.3231165996605));
#33460=CARTESIAN_POINT('Ctrl Pts',(18.1460502915689,34.4938764679129,35.1725117883411));
#33461=CARTESIAN_POINT('Ctrl Pts',(18.1460502915689,34.4938764679129,35.0294657090004));
#33462=CARTESIAN_POINT('Ctrl Pts',(18.1460502915689,34.4938764679129,34.8864196296597));
#33463=CARTESIAN_POINT('Ctrl Pts',(18.1292923320046,34.522878497267,34.7358148183402));
#33464=CARTESIAN_POINT('Ctrl Pts',(18.069284710185,34.6385464913584,34.463208654044));
#33465=CARTESIAN_POINT('Ctrl Pts',(18.0267768582634,34.7255600011841,34.3411920900928));
#33466=CARTESIAN_POINT('Ctrl Pts',(17.9435339040124,34.9253475867885,34.1458660406716));
#33467=CARTESIAN_POINT('Ctrl Pts',(17.8925030363182,35.0681727125076,34.0523228587036));
#33468=CARTESIAN_POINT('Ctrl Pts',(17.7876418033145,35.4462639140502,33.8793991986791));
#33469=CARTESIAN_POINT('Ctrl Pts',(17.7397894030341,35.7740490184036,33.8211629139253));
#33470=CARTESIAN_POINT('Ctrl Pts',(17.7397894030341,36.3346151799028,33.8211629139253));
#33471=CARTESIAN_POINT('Ctrl Pts',(17.7876418033145,36.6624002842562,33.8793991986791));
#33472=CARTESIAN_POINT('Ctrl Pts',(17.8836292597541,37.0084958974654,34.0376893675864));
#33473=CARTESIAN_POINT('Ctrl Pts',(17.9192709480126,37.1152646037045,34.1009670111741));
#33474=CARTESIAN_POINT('Ctrl Pts',(17.9535710587063,37.2043320991532,34.1733882146302));
#33475=CARTESIAN_POINT('Origin',(16.1460502915689,37.2043320991532,35.0294657090004));
#33476=CARTESIAN_POINT('Origin',(16.1460502915689,31.9543320991532,35.0294657090004));
#33477=CARTESIAN_POINT('',(16.1460502915689,38.7043320991532,33.0294657090004));
#33478=CARTESIAN_POINT('Origin',(16.1460502915689,38.7043320991532,35.0294657090004));
#33479=CARTESIAN_POINT('',(16.1460502915689,31.9543320991532,33.0294657090004));
#33480=CARTESIAN_POINT('Origin',(35.9397894030341,31.9543320991532,38.5294657090004));
#33481=CARTESIAN_POINT('',(35.9397894030341,31.9543320991532,37.3294657090004));
#33482=CARTESIAN_POINT('Origin',(20.9397894030341,36.0543320991532,41.0294657090004));
#33483=CARTESIAN_POINT('',(19.1460502915689,38.7043320991532,41.0294657090004));
#33484=CARTESIAN_POINT('',(17.9535710587063,37.2043320991532,41.0294657090004));
#33485=CARTESIAN_POINT('',(17.9535710587063,37.2043320991532,41.0294657090004));
#33486=CARTESIAN_POINT('Origin',(54.9397894030341,37.9543320991532,41.0294657090004));
#33487=CARTESIAN_POINT('',(56.9397894030341,37.9543320991532,41.0294657090004));
#33488=CARTESIAN_POINT('Origin',(43.4397894030341,37.9543320991532,41.0294657090004));
#33489=CARTESIAN_POINT('',(44.9397894030341,37.9543320991532,41.0294657090004));
#33490=CARTESIAN_POINT('Origin',(0.939789403034137,43.9543320991532,41.0294657090004));
#33491=CARTESIAN_POINT('',(0.939789403034137,43.6543320991532,41.0294657090004));
#33492=CARTESIAN_POINT('',(0.939789403034137,39.9843320991532,41.0294657090004));
#33493=CARTESIAN_POINT('',(0.939789403034137,43.9543320991532,41.0294657090004));
#33494=CARTESIAN_POINT('',(0.939789403034137,43.6543320991532,29.0294657090004));
#33495=CARTESIAN_POINT('',(0.939789403034137,43.6543320991532,41.0294657090004));
#33496=CARTESIAN_POINT('',(0.939789403034137,39.9843320991532,29.0294657090004));
#33497=CARTESIAN_POINT('',(0.939789403034137,43.9543320991532,29.0294657090004));
#33498=CARTESIAN_POINT('',(0.939789403034137,39.9843320991532,41.0294657090004));
#33499=CARTESIAN_POINT('Origin',(60.9397894030341,43.9543320991532,35.0294657090004));
#33500=CARTESIAN_POINT('',(60.9397894030341,43.6543320991532,29.3294657090004));
#33501=CARTESIAN_POINT('',(60.9397894030341,43.6543320991532,34.7294657090004));
#33502=CARTESIAN_POINT('',(60.9397894030341,43.6543320991532,35.0294657090004));
#33503=CARTESIAN_POINT('',(60.9397894030341,32.2543320991532,34.7294657090004));
#33504=CARTESIAN_POINT('',(60.9397894030341,43.9543320991532,34.7294657090004));
#33505=CARTESIAN_POINT('',(60.9397894030341,32.2543320991532,29.3294657090004));
#33506=CARTESIAN_POINT('',(60.9397894030341,32.2543320991532,29.0294657090004));
#33507=CARTESIAN_POINT('',(60.9397894030341,43.9543320991532,29.3294657090004));
#33508=CARTESIAN_POINT('Origin',(0.939789403034137,43.9543320991532,29.0294657090004));
#33509=CARTESIAN_POINT('',(13.1738772623021,38.7043320991532,29.0294657090004));
#33510=CARTESIAN_POINT('',(19.1460502915689,38.7043320991532,29.0294657090004));
#33511=CARTESIAN_POINT('',(4.70570154376622,38.7043320991532,29.0294657090004));
#33512=CARTESIAN_POINT('Origin',(8.93978940303414,37.9543320991532,29.0294657090004));
#33513=CARTESIAN_POINT('',(2.61978940303414,38.7043320991532,29.0294657090004));
#33514=CARTESIAN_POINT('',(5.01073099165871,38.7043320991532,29.0294657090004));
#33515=CARTESIAN_POINT('',(2.61978940303414,40.9543320991532,29.0294657090004));
#33516=CARTESIAN_POINT('',(2.61978940303414,40.9543320991532,29.0294657090004));
#33517=CARTESIAN_POINT('',(0.939789403034137,39.9843320991532,29.0294657090004));
#33518=CARTESIAN_POINT('',(60.6397894030341,43.6543320991532,29.0294657090004));
#33519=CARTESIAN_POINT('',(0.939789403034137,43.6543320991532,29.0294657090004));
#33520=CARTESIAN_POINT('',(60.6397894030341,32.2543320991532,29.0294657090004));
#33521=CARTESIAN_POINT('',(60.6397894030341,43.9543320991532,29.0294657090004));
#33522=CARTESIAN_POINT('',(0.939789403034137,32.2543320991532,29.0294657090004));
#33523=CARTESIAN_POINT('',(0.939789403034137,32.2543320991532,29.0294657090004));
#33524=CARTESIAN_POINT('',(0.939789403034137,35.9243320991532,29.0294657090004));
#33525=CARTESIAN_POINT('',(0.939789403034137,43.9543320991532,29.0294657090004));
#33526=CARTESIAN_POINT('',(2.61978940303414,34.9543320991532,29.0294657090004));
#33527=CARTESIAN_POINT('',(2.61978940303414,34.9543320991532,29.0294657090004));
#33528=CARTESIAN_POINT('',(2.61978940303414,37.2043320991532,29.0294657090004));
#33529=CARTESIAN_POINT('',(2.61978940303414,37.2043320991532,29.0294657090004));
#33530=CARTESIAN_POINT('',(4.70570154376622,37.2043320991532,29.0294657090004));
#33531=CARTESIAN_POINT('',(5.01073099165871,37.2043320991532,29.0294657090004));
#33532=CARTESIAN_POINT('',(13.1738772623021,37.2043320991532,29.0294657090004));
#33533=CARTESIAN_POINT('Origin',(8.93978940303414,37.9543320991532,29.0294657090004));
#33534=CARTESIAN_POINT('',(17.9535710587063,37.2043320991532,29.0294657090004));
#33535=CARTESIAN_POINT('Origin',(0.939789403034137,43.9543320991532,41.0294657090004));
#33536=CARTESIAN_POINT('',(0.939789403034137,32.2543320991532,41.0294657090004));
#33537=CARTESIAN_POINT('',(0.939789403034137,32.2543320991532,41.0294657090004));
#33538=CARTESIAN_POINT('',(0.939789403034137,35.9243320991532,41.0294657090004));
#33539=CARTESIAN_POINT('',(0.939789403034137,43.9543320991532,41.0294657090004));
#33540=CARTESIAN_POINT('',(0.939789403034137,35.9243320991532,41.0294657090004));
#33541=CARTESIAN_POINT('Origin',(0.939789403034137,43.9543320991532,41.0294657090004));
#33542=CARTESIAN_POINT('',(13.173877262302,38.7043320991532,41.0294657090004));
#33543=CARTESIAN_POINT('',(19.1460502915689,38.7043320991532,41.0294657090004));
#33544=CARTESIAN_POINT('',(13.173877262302,37.2043320991532,41.0294657090004));
#33545=CARTESIAN_POINT('',(17.9535710587063,37.2043320991532,41.0294657090004));
#33546=CARTESIAN_POINT('',(4.70570154376624,37.2043320991532,41.0294657090004));
#33547=CARTESIAN_POINT('Origin',(8.93978940303414,37.9543320991532,41.0294657090004));
#33548=CARTESIAN_POINT('',(2.61978940303414,37.2043320991532,41.0294657090004));
#33549=CARTESIAN_POINT('',(5.01073099165871,37.2043320991532,41.0294657090004));
#33550=CARTESIAN_POINT('',(2.61978940303414,34.9543320991532,41.0294657090004));
#33551=CARTESIAN_POINT('',(2.61978940303414,37.2043320991532,41.0294657090004));
#33552=CARTESIAN_POINT('',(2.61978940303414,34.9543320991532,41.0294657090004));
#33553=CARTESIAN_POINT('',(32.5397894030341,32.2543320991532,41.0294657090004));
#33554=CARTESIAN_POINT('',(32.8397894030341,32.2543320991532,41.0294657090004));
#33555=CARTESIAN_POINT('',(32.5397894030341,34.2543320991532,41.0294657090004));
#33556=CARTESIAN_POINT('',(32.5397894030341,43.9543320991532,41.0294657090004));
#33557=CARTESIAN_POINT('',(37.6397894030341,34.2543320991532,41.0294657090004));
#33558=CARTESIAN_POINT('',(0.939789403034137,34.2543320991532,41.0294657090004));
#33559=CARTESIAN_POINT('',(37.6397894030341,41.6543320991532,41.0294657090004));
#33560=CARTESIAN_POINT('',(37.6397894030341,43.9543320991532,41.0294657090004));
#33561=CARTESIAN_POINT('',(32.5397894030341,41.6543320991532,41.0294657090004));
#33562=CARTESIAN_POINT('',(0.939789403034137,41.6543320991532,41.0294657090004));
#33563=CARTESIAN_POINT('',(32.5397894030341,43.6543320991532,41.0294657090004));
#33564=CARTESIAN_POINT('',(32.5397894030341,43.9543320991532,41.0294657090004));
#33565=CARTESIAN_POINT('',(0.939789403034137,43.6543320991532,41.0294657090004));
#33566=CARTESIAN_POINT('',(2.61978940303414,40.9543320991532,41.0294657090004));
#33567=CARTESIAN_POINT('',(0.939789403034137,39.9843320991532,41.0294657090004));
#33568=CARTESIAN_POINT('',(2.61978940303414,38.7043320991532,41.0294657090004));
#33569=CARTESIAN_POINT('',(2.61978940303414,40.9543320991532,41.0294657090004));
#33570=CARTESIAN_POINT('',(4.70570154376623,38.7043320991532,41.0294657090004));
#33571=CARTESIAN_POINT('',(5.01073099165871,38.7043320991532,41.0294657090004));
#33572=CARTESIAN_POINT('Origin',(8.93978940303414,37.9543320991532,41.0294657090004));
#33573=CARTESIAN_POINT('Origin',(37.9397894030341,43.9543320991532,41.0294657090004));
#33574=CARTESIAN_POINT('',(37.9397894030341,41.9543320991532,35.0294657090004));
#33575=CARTESIAN_POINT('',(37.9397894030341,41.9543320991532,40.7294657090004));
#33576=CARTESIAN_POINT('',(37.9397894030341,41.9543320991532,41.0294657090004));
#33577=CARTESIAN_POINT('',(37.9397894030341,33.9543320991532,40.7294657090004));
#33578=CARTESIAN_POINT('',(37.9397894030341,43.9543320991532,40.7294657090004));
#33579=CARTESIAN_POINT('',(37.9397894030341,33.9543320991532,35.0294657090004));
#33580=CARTESIAN_POINT('',(37.9397894030341,33.9543320991532,41.0294657090004));
#33581=CARTESIAN_POINT('',(37.9397894030341,43.9543320991532,35.0294657090004));
#33582=CARTESIAN_POINT('Origin',(60.9397894030341,43.9543320991532,35.0294657090004));
#33583=CARTESIAN_POINT('',(43.0397894030341,33.9543320991532,35.0294657090004));
#33584=CARTESIAN_POINT('',(43.0397894030341,32.2543320991532,35.0294657090004));
#33585=CARTESIAN_POINT('',(43.0397894030341,43.9543320991532,35.0294657090004));
#33586=CARTESIAN_POINT('',(60.6397894030341,32.2543320991532,35.0294657090004));
#33587=CARTESIAN_POINT('',(60.9397894030341,32.2543320991532,35.0294657090004));
#33588=CARTESIAN_POINT('',(60.6397894030341,43.6543320991532,35.0294657090004));
#33589=CARTESIAN_POINT('',(60.6397894030341,43.9543320991532,35.0294657090004));
#33590=CARTESIAN_POINT('',(35.8397894030342,43.6543320991532,35.0294657090004));
#33591=CARTESIAN_POINT('',(60.9397894030341,43.6543320991532,35.0294657090004));
#33592=CARTESIAN_POINT('',(35.8397894030342,41.9543320991532,35.0294657090004));
#33593=CARTESIAN_POINT('',(35.8397894030342,41.9543320991532,35.0294657090004));
#33594=CARTESIAN_POINT('',(35.8397894030342,41.9543320991532,35.0294657090004));
#33595=CARTESIAN_POINT('',(60.9397894030341,33.9543320991532,35.0294657090004));
#33596=CARTESIAN_POINT('Origin',(30.9397894030341,43.9543320991532,35.0294657090004));
#33597=CARTESIAN_POINT('',(60.6397894030341,43.9543320991532,29.3294657090004));
#33598=CARTESIAN_POINT('',(1.23978940303414,43.9543320991532,29.3294657090004));
#33599=CARTESIAN_POINT('',(30.9397894030341,43.9543320991532,29.3294657090004));
#33600=CARTESIAN_POINT('',(1.23978940303414,43.9543320991532,40.7294657090004));
#33601=CARTESIAN_POINT('',(1.23978940303414,43.9543320991532,35.0294657090004));
#33602=CARTESIAN_POINT('',(32.5397894030341,43.9543320991532,40.7294657090004));
#33603=CARTESIAN_POINT('',(30.9397894030341,43.9543320991532,40.7294657090004));
#33604=CARTESIAN_POINT('',(32.5397894030341,43.9543320991532,38.0294657090004));
#33605=CARTESIAN_POINT('',(32.5397894030341,43.9543320991532,35.0294657090004));
#33606=CARTESIAN_POINT('',(35.8397894030342,43.9543320991532,34.7294657090004));
#33607=CARTESIAN_POINT('Origin',(35.8397894030341,43.9543320991532,38.0294657090004));
#33608=CARTESIAN_POINT('',(60.6397894030341,43.9543320991532,34.7294657090004));
#33609=CARTESIAN_POINT('',(30.9397894030341,43.9543320991532,34.7294657090004));
#33610=CARTESIAN_POINT('',(60.6397894030341,43.9543320991532,35.0294657090004));
#33611=CARTESIAN_POINT('Origin',(30.9397894030341,31.9543320991532,35.0294657090004));
#33612=CARTESIAN_POINT('',(60.6397894030341,31.9543320991532,29.3294657090004));
#33613=CARTESIAN_POINT('',(60.6397894030341,31.9543320991532,34.7294657090004));
#33614=CARTESIAN_POINT('',(60.6397894030341,31.9543320991532,35.0294657090004));
#33615=CARTESIAN_POINT('',(43.3397894030341,31.9543320991532,34.7294657090004));
#33616=CARTESIAN_POINT('',(43.0397894030341,31.9543320991532,34.7294657090004));
#33617=CARTESIAN_POINT('',(43.3397894030341,31.9543320991532,34.72672445582));
#33618=CARTESIAN_POINT('',(43.3397894030341,31.9543320991532,35.02672445582));
#33619=CARTESIAN_POINT('',(35.8397894030342,31.9543320991532,34.72672445582));
#33620=CARTESIAN_POINT('',(35.8397894030342,31.9543320991532,34.72672445582));
#33621=CARTESIAN_POINT('',(32.5397894030341,31.9543320991532,38.02672445582));
#33622=CARTESIAN_POINT('Origin',(35.8397894030341,31.9543320991532,38.02672445582));
#33623=CARTESIAN_POINT('',(32.5397894030341,31.9543320991532,40.7294657090004));
#33624=CARTESIAN_POINT('',(32.5397894030341,31.9543320991532,41.0294657090004));
#33625=CARTESIAN_POINT('',(1.23978940303414,31.9543320991532,40.7294657090004));
#33626=CARTESIAN_POINT('',(0.939789403034137,31.9543320991532,40.7294657090004));
#33627=CARTESIAN_POINT('',(1.23978940303414,31.9543320991532,29.3294657090004));
#33628=CARTESIAN_POINT('',(1.23978940303414,31.9543320991532,29.0294657090004));
#33629=CARTESIAN_POINT('',(60.9397894030341,31.9543320991532,29.3294657090004));
#33630=CARTESIAN_POINT('Origin',(8.93978940303414,37.9543320991532,41.0294657090004));
#33631=CARTESIAN_POINT('',(12.8688478144096,37.2043320991532,40.7294657090004));
#33632=CARTESIAN_POINT('',(12.8688478144096,37.2043320991532,29.3294657090004));
#33633=CARTESIAN_POINT('',(12.8688478144096,37.2043320991532,41.0294657090004));
#33634=CARTESIAN_POINT('',(5.01073099165871,37.2043320991532,29.3294657090004));
#33635=CARTESIAN_POINT('Origin',(8.93978940303414,37.9543320991532,29.3294657090004));
#33636=CARTESIAN_POINT('',(5.01073099165871,37.2043320991532,40.7294657090004));
#33637=CARTESIAN_POINT('',(5.01073099165871,37.2043320991532,41.0294657090004));
#33638=CARTESIAN_POINT('Origin',(8.93978940303414,37.9543320991532,40.7294657090004));
#33639=CARTESIAN_POINT('Origin',(17.9535710587063,37.2043320991532,41.0294657090004));
#33640=CARTESIAN_POINT('Ctrl Pts',(13.1738772623021,37.2043320991532,29.0294657090004));
#33641=CARTESIAN_POINT('Ctrl Pts',(13.0722597271638,37.2043320991532,29.1295256094231));
#33642=CARTESIAN_POINT('Ctrl Pts',(12.9705877024409,37.2043320991532,29.2295302182899));
#33643=CARTESIAN_POINT('Ctrl Pts',(12.8688478144096,37.2043320991532,29.3294657090004));
#33644=CARTESIAN_POINT('Ctrl Pts',(12.8688478144096,37.2043320991532,40.7294657090004));
#33645=CARTESIAN_POINT('Ctrl Pts',(12.9705877024409,37.2043320991532,40.8294011997109));
#33646=CARTESIAN_POINT('Ctrl Pts',(13.0722597271638,37.2043320991532,40.9294058085777));
#33647=CARTESIAN_POINT('Ctrl Pts',(13.173877262302,37.2043320991532,41.0294657090004));
#33648=CARTESIAN_POINT('Origin',(19.1460502915689,38.7043320991532,41.0294657090004));
#33649=CARTESIAN_POINT('',(12.8688478144096,38.7043320991532,40.7294657090004));
#33650=CARTESIAN_POINT('',(12.8688478144096,38.7043320991532,29.3294657090004));
#33651=CARTESIAN_POINT('',(12.8688478144096,38.7043320991532,41.0294657090004));
#33652=CARTESIAN_POINT('Ctrl Pts',(12.8688478144096,38.7043320991532,29.3294657090004));
#33653=CARTESIAN_POINT('Ctrl Pts',(12.9705877024409,38.7043320991532,29.2295302182899));
#33654=CARTESIAN_POINT('Ctrl Pts',(13.0722597271638,38.7043320991532,29.1295256094231));
#33655=CARTESIAN_POINT('Ctrl Pts',(13.1738772623021,38.7043320991532,29.0294657090004));
#33656=CARTESIAN_POINT('Ctrl Pts',(13.173877262302,38.7043320991532,41.0294657090004));
#33657=CARTESIAN_POINT('Ctrl Pts',(13.0722597271638,38.7043320991532,40.9294058085776));
#33658=CARTESIAN_POINT('Ctrl Pts',(12.9705877024409,38.7043320991532,40.8294011997109));
#33659=CARTESIAN_POINT('Ctrl Pts',(12.8688478144096,38.7043320991532,40.7294657090004));
#33660=CARTESIAN_POINT('Origin',(8.93978940303414,37.9543320991532,41.0294657090004));
#33661=CARTESIAN_POINT('',(5.01073099165871,38.7043320991532,40.7294657090004));
#33662=CARTESIAN_POINT('',(5.01073099165871,38.7043320991532,29.3294657090004));
#33663=CARTESIAN_POINT('',(5.01073099165871,38.7043320991532,41.0294657090004));
#33664=CARTESIAN_POINT('Origin',(8.93978940303414,37.9543320991532,29.3294657090004));
#33665=CARTESIAN_POINT('Origin',(8.93978940303414,37.9543320991532,40.7294657090004));
#33666=CARTESIAN_POINT('Origin',(5.01073099165871,38.7043320991532,41.0294657090004));
#33667=CARTESIAN_POINT('Ctrl Pts',(4.70570154376622,38.7043320991532,29.0294657090004));
#33668=CARTESIAN_POINT('Ctrl Pts',(4.80731907890448,38.7043320991532,29.1295256094231));
#33669=CARTESIAN_POINT('Ctrl Pts',(4.90899110362736,38.7043320991532,29.2295302182899));
#33670=CARTESIAN_POINT('Ctrl Pts',(5.01073099165871,38.7043320991532,29.3294657090004));
#33671=CARTESIAN_POINT('Ctrl Pts',(5.01073099165871,38.7043320991532,40.7294657090004));
#33672=CARTESIAN_POINT('Ctrl Pts',(4.90899110362737,38.7043320991532,40.8294011997109));
#33673=CARTESIAN_POINT('Ctrl Pts',(4.80731907890448,38.7043320991532,40.9294058085776));
#33674=CARTESIAN_POINT('Ctrl Pts',(4.70570154376623,38.7043320991532,41.0294657090004));
#33675=CARTESIAN_POINT('',(2.61978940303414,38.7043320991532,41.0294657090004));
#33676=CARTESIAN_POINT('Origin',(2.61978940303414,40.9543320991532,41.0294657090004));
#33677=CARTESIAN_POINT('',(2.61978940303414,40.9543320991532,41.0294657090004));
#33678=CARTESIAN_POINT('Origin',(0.939789403034137,39.9843320991532,41.0294657090004));
#33679=CARTESIAN_POINT('Origin',(2.61978940303414,34.9543320991532,41.0294657090004));
#33680=CARTESIAN_POINT('',(2.61978940303414,34.9543320991532,41.0294657090004));
#33681=CARTESIAN_POINT('Origin',(2.61978940303414,37.2043320991532,41.0294657090004));
#33682=CARTESIAN_POINT('',(2.61978940303414,37.2043320991532,41.0294657090004));
#33683=CARTESIAN_POINT('Origin',(5.01073099165871,37.2043320991532,41.0294657090004));
#33684=CARTESIAN_POINT('Ctrl Pts',(5.01073099165871,37.2043320991532,29.3294657090004));
#33685=CARTESIAN_POINT('Ctrl Pts',(4.90899110362736,37.2043320991532,29.2295302182899));
#33686=CARTESIAN_POINT('Ctrl Pts',(4.80731907890448,37.2043320991532,29.1295256094231));
#33687=CARTESIAN_POINT('Ctrl Pts',(4.70570154376622,37.2043320991532,29.0294657090004));
#33688=CARTESIAN_POINT('Ctrl Pts',(4.70570154376624,37.2043320991532,41.0294657090004));
#33689=CARTESIAN_POINT('Ctrl Pts',(4.80731907890449,37.2043320991532,40.9294058085777));
#33690=CARTESIAN_POINT('Ctrl Pts',(4.90899110362737,37.2043320991532,40.8294011997109));
#33691=CARTESIAN_POINT('Ctrl Pts',(5.01073099165871,37.2043320991532,40.7294657090004));
#33692=CARTESIAN_POINT('Origin',(35.8397894030341,33.9543320991532,38.02672445582));
#33693=CARTESIAN_POINT('',(32.8397894030341,33.9543320991532,40.7294657090004));
#33694=CARTESIAN_POINT('',(35.8397894030341,33.9543320991532,40.7294657090004));
#33695=CARTESIAN_POINT('',(32.8397894030341,33.9543320991532,38.02672445582));
#33696=CARTESIAN_POINT('',(32.8397894030341,33.9543320991532,47.0322069621808));
#33697=CARTESIAN_POINT('',(35.8397894030342,33.9543320991532,35.02672445582));
#33698=CARTESIAN_POINT('Origin',(35.8397894030341,33.9543320991532,38.02672445582));
#33699=CARTESIAN_POINT('',(43.0397894030341,33.9543320991532,35.02672445582));
#33700=CARTESIAN_POINT('',(43.0397894030341,33.9543320991532,35.02672445582));
#33701=CARTESIAN_POINT('',(43.0397894030341,33.9543320991532,47.0322069621808));
#33702=CARTESIAN_POINT('Origin',(43.0397894030341,33.9543320991532,47.0322069621808));
#33703=CARTESIAN_POINT('',(43.0397894030341,32.2543320991532,35.02672445582));
#33704=CARTESIAN_POINT('',(43.0397894030341,33.9543320991532,35.02672445582));
#33705=CARTESIAN_POINT('',(43.0397894030341,32.2543320991532,35.0294657090004));
#33706=CARTESIAN_POINT('Origin',(32.8397894030341,33.9543320991532,47.0322069621808));
#33707=CARTESIAN_POINT('',(32.8397894030341,32.2543320991532,40.7294657090004));
#33708=CARTESIAN_POINT('',(32.8397894030341,33.9543320991532,40.7294657090004));
#33709=CARTESIAN_POINT('',(32.8397894030341,32.2543320991532,38.02672445582));
#33710=CARTESIAN_POINT('',(32.8397894030341,32.2543320991532,38.02672445582));
#33711=CARTESIAN_POINT('',(32.8397894030341,33.9543320991532,38.02672445582));
#33712=CARTESIAN_POINT('Origin',(43.0397894030341,33.9543320991532,35.02672445582));
#33713=CARTESIAN_POINT('',(35.8397894030342,32.2543320991532,35.02672445582));
#33714=CARTESIAN_POINT('',(35.8397894030342,33.9543320991532,35.02672445582));
#33715=CARTESIAN_POINT('',(43.0397894030341,32.2543320991532,35.02672445582));
#33716=CARTESIAN_POINT('Origin',(35.8397894030341,33.9543320991532,38.02672445582));
#33717=CARTESIAN_POINT('Origin',(35.8397894030341,32.2543320991532,38.02672445582));
#33718=CARTESIAN_POINT('Origin',(35.8397894030341,41.9543320991532,38.0294657090004));
#33719=CARTESIAN_POINT('',(32.8397894030341,41.9543320991532,38.0294657090004));
#33720=CARTESIAN_POINT('',(32.8397894030341,41.9543320991532,40.7294657090004));
#33721=CARTESIAN_POINT('',(32.8397894030341,41.9543320991532,47.0294657090004));
#33722=CARTESIAN_POINT('',(35.8397894030341,41.9543320991532,40.7294657090004));
#33723=CARTESIAN_POINT('Origin',(35.8397894030341,41.9543320991532,38.0294657090004));
#33724=CARTESIAN_POINT('Origin',(32.8397894030341,41.9543320991532,47.0294657090004));
#33725=CARTESIAN_POINT('',(32.8397894030341,43.6543320991532,38.0294657090004));
#33726=CARTESIAN_POINT('',(32.8397894030341,43.6543320991532,40.7294657090004));
#33727=CARTESIAN_POINT('',(32.8397894030341,43.6543320991532,47.0294657090004));
#33728=CARTESIAN_POINT('',(32.8397894030341,41.9543320991532,40.7294657090004));
#33729=CARTESIAN_POINT('',(32.8397894030341,41.9543320991532,38.0294657090004));
#33730=CARTESIAN_POINT('Origin',(35.8397894030341,41.9543320991532,38.0294657090004));
#33731=CARTESIAN_POINT('Origin',(35.8397894030341,43.6543320991532,38.0294657090004));
#33732=CARTESIAN_POINT('Origin',(30.9397894030341,43.6543320991532,40.7294657090004));
#33733=CARTESIAN_POINT('Origin',(32.5397894030341,43.6543320991532,40.7294657090004));
#33734=CARTESIAN_POINT('Origin',(1.23978940303386,43.6543320991535,40.7294657090006));
#33735=CARTESIAN_POINT('Origin',(1.23978940303414,43.6543320991532,35.0294657090004));
#33736=CARTESIAN_POINT('Origin',(1.23978940303469,43.6543320991527,29.3294657090009));
#33737=CARTESIAN_POINT('Origin',(32.5397894030341,43.6543320991532,47.0294657090004));
#33738=CARTESIAN_POINT('Origin',(32.5397894030341,43.6543320991532,40.7294657090004));
#33739=CARTESIAN_POINT('Origin',(32.5397894030341,43.6543320991532,38.0294657090004));
#33740=CARTESIAN_POINT('Origin',(30.9397894030341,43.6543320991532,29.3294657090004));
#33741=CARTESIAN_POINT('Origin',(60.6397894030341,43.6543320991532,29.3294657090004));
#33742=CARTESIAN_POINT('Origin',(0.939789403034137,32.2543320991532,40.7294657090004));
#33743=CARTESIAN_POINT('Origin',(32.5397894030341,32.2543320991532,40.7294657090004));
#33744=CARTESIAN_POINT('Origin',(1.23978940303371,32.2543320991528,40.7294657090008));
#33745=CARTESIAN_POINT('Origin',(35.8397894030341,43.6543320991532,38.0294657090004));
#33746=CARTESIAN_POINT('Origin',(35.8397894030342,43.6543320991532,34.7294657090004));
#33747=CARTESIAN_POINT('Origin',(60.6397894030341,43.6543320991532,29.3294657090004));
#33748=CARTESIAN_POINT('Origin',(60.6397894030341,43.6543320991532,29.3294657090004));
#33749=CARTESIAN_POINT('Origin',(60.6397894030341,43.6543320991532,29.3294657090004));
#33750=CARTESIAN_POINT('Origin',(1.23978940303414,32.2543320991532,41.0294657090004));
#33751=CARTESIAN_POINT('Origin',(1.23978940303447,32.2543320991536,29.3294657090007));
#33752=CARTESIAN_POINT('Origin',(32.5397894030341,32.2543320991532,47.0322069621808));
#33753=CARTESIAN_POINT('Origin',(32.5397894030341,32.2543320991532,40.7294657090004));
#33754=CARTESIAN_POINT('Origin',(32.5397894030341,32.2543320991532,38.02672445582));
#33755=CARTESIAN_POINT('Origin',(30.9397894030341,43.6543320991532,34.7294657090004));
#33756=CARTESIAN_POINT('Origin',(60.6397894030341,43.6543320991532,34.7294657090004));
#33757=CARTESIAN_POINT('Origin',(60.6397894030341,43.6543320991532,35.0294657090004));
#33758=CARTESIAN_POINT('Origin',(60.6397894030341,43.6543320991532,34.7294657090004));
#33759=CARTESIAN_POINT('Origin',(60.6397894030341,43.9543320991532,29.3294657090004));
#33760=CARTESIAN_POINT('Origin',(60.6397894030341,32.2543320991532,29.3294657090004));
#33761=CARTESIAN_POINT('Origin',(0.939789403034137,32.2543320991532,29.3294657090004));
#33762=CARTESIAN_POINT('Origin',(60.6397894030341,32.2543320991532,29.3294657090004));
#33763=CARTESIAN_POINT('Origin',(35.8397894030341,32.2543320991532,38.02672445582));
#33764=CARTESIAN_POINT('Origin',(35.8397894030342,32.2543320991532,34.72672445582));
#33765=CARTESIAN_POINT('Origin',(60.6397894030341,43.6543320991532,34.7294657090004));
#33766=CARTESIAN_POINT('Origin',(60.6397894030341,43.6543320991532,34.7294657090004));
#33767=CARTESIAN_POINT('Origin',(60.6397894030341,32.2543320991532,29.3294657090004));
#33768=CARTESIAN_POINT('Origin',(60.6397894030341,32.2543320991532,29.3294657090004));
#33769=CARTESIAN_POINT('Origin',(43.0397894030341,32.2543320991532,34.72672445582));
#33770=CARTESIAN_POINT('Origin',(43.3397894030341,32.2543320991531,34.72672445582));
#33771=CARTESIAN_POINT('Origin',(60.6397894030341,43.9543320991532,34.7294657090004));
#33772=CARTESIAN_POINT('Origin',(60.6397894030341,32.2543320991532,34.7294657090004));
#33773=CARTESIAN_POINT('Origin',(60.6397894030341,32.2543320991532,35.0294657090004));
#33774=CARTESIAN_POINT('Origin',(60.6397894030341,32.2543320991532,34.7294657090004));
#33775=CARTESIAN_POINT('Origin',(43.3397894030341,32.2543320991532,47.0322069621808));
#33776=CARTESIAN_POINT('Origin',(43.3397894030341,32.2543320991532,34.7294657090004));
#33777=CARTESIAN_POINT('Origin',(60.6397894030341,32.2543320991532,34.7294657090004));
#33778=CARTESIAN_POINT('Origin',(60.6397894030341,32.2543320991532,34.7294657090004));
#33779=CARTESIAN_POINT('Origin',(60.9397894030341,32.2543320991532,34.7294657090004));
#33780=CARTESIAN_POINT('Origin',(32.5397894030341,43.6543320991532,40.7294657090004));
#33781=CARTESIAN_POINT('Origin',(32.5397894030341,43.6543320991532,40.7294657090004));
#33782=CARTESIAN_POINT('Origin',(32.5397894030341,43.9543320991532,40.7294657090004));
#33783=CARTESIAN_POINT('Origin',(32.5397894030357,41.6543320991548,40.7294657090019));
#33784=CARTESIAN_POINT('Origin',(0.939789403034137,41.6543320991532,40.7294657090004));
#33785=CARTESIAN_POINT('Origin',(37.6397894030353,41.6543320991544,40.7294657090015));
#33786=CARTESIAN_POINT('Origin',(37.6397894030341,43.9543320991532,40.7294657090004));
#33787=CARTESIAN_POINT('Origin',(37.6397894030347,34.2543320991526,40.729465709001));
#33788=CARTESIAN_POINT('Origin',(0.939789403034137,34.2543320991532,40.7294657090004));
#33789=CARTESIAN_POINT('Origin',(32.5397894030352,34.2543320991522,40.7294657090014));
#33790=CARTESIAN_POINT('Origin',(32.5397894030341,43.9543320991532,40.7294657090004));
#33791=CARTESIAN_POINT('Origin',(32.5397894030341,32.2543320991532,40.7294657090004));
#33792=CARTESIAN_POINT('Origin',(32.5397894030341,32.2543320991532,40.7294657090004));
#33793=CARTESIAN_POINT('Origin',(8.93978940303414,37.9543320991532,29.3294657090004));
#33794=CARTESIAN_POINT('Origin',(8.93978940303414,37.9543320991532,29.3294657090004));
#33795=CARTESIAN_POINT('Origin',(8.93978940303414,37.9543320991532,41.0294657090004));
#33796=CARTESIAN_POINT('Origin',(8.93978940303414,37.9543320991532,41.0294657090004));
#33797=CARTESIAN_POINT('Origin',(35.9397894030337,32.0543320991536,38.5294657090004));
#33798=CARTESIAN_POINT('',(34.8397894030337,31.9543320991536,38.5294657090004));
#33799=CARTESIAN_POINT('Origin',(35.9397894030337,31.9543320991536,38.5294657090004));
#33800=CARTESIAN_POINT('',(34.7397894030337,32.0543320991536,38.5294657090004));
#33801=CARTESIAN_POINT('Origin',(34.8397894030337,32.0543320991536,38.5294657090004));
#33802=CARTESIAN_POINT('',(37.1397894030337,32.0543320991536,38.5294657090004));
#33803=CARTESIAN_POINT('Origin',(35.9397894030337,32.0543320991536,38.5294657090004));
#33804=CARTESIAN_POINT('Origin',(35.9397894030337,32.0543320991536,38.5294657090004));
#33805=CARTESIAN_POINT('Origin',(35.9397894030336,43.8543320991536,38.5294657090005));
#33806=CARTESIAN_POINT('',(37.1397894030336,43.8543320991536,38.5294657090004));
#33807=CARTESIAN_POINT('',(34.7397894030336,43.8543320991536,38.5294657090005));
#33808=CARTESIAN_POINT('Origin',(35.9397894030336,43.8543320991536,38.5294657090005));
#33809=CARTESIAN_POINT('Origin',(35.9397894030336,43.8543320991536,38.5294657090005));
#33810=CARTESIAN_POINT('',(34.8397894030336,43.9543320991536,38.5294657090005));
#33811=CARTESIAN_POINT('Origin',(34.8397894030336,43.8543320991536,38.5294657090005));
#33812=CARTESIAN_POINT('Origin',(35.9397894030336,43.9543320991536,38.5294657090005));
#33813=CARTESIAN_POINT('Origin',(35.9397894030337,31.9543320991536,38.5294657090004));
#33814=CARTESIAN_POINT('',(37.1397894030337,31.9543320991536,38.5294657090004));
#33815=CARTESIAN_POINT('Origin',(35.9397894030337,31.9543320991536,38.5294657090004));
#33816=CARTESIAN_POINT('Origin',(35.9397894030336,43.9543320991536,38.5294657090005));
#33817=CARTESIAN_POINT('Origin',(71.9308774154808,37.9543320991532,39.3304548976388));
#33818=CARTESIAN_POINT('',(66.9321151915299,35.4543320991532,39.2192063992168));
#33819=CARTESIAN_POINT('Origin',(66.9321151915299,37.9543320991532,39.2192063992168));
#33820=CARTESIAN_POINT('',(71.9308774154808,35.4543320991532,39.3304548976388));
#33821=CARTESIAN_POINT('',(71.9308774154808,35.4543320991532,39.3304548976388));
#33822=CARTESIAN_POINT('Origin',(71.9308774154808,37.9543320991532,39.3304548976388));
#33823=CARTESIAN_POINT('Origin',(66.9321151915299,37.9543320991532,39.2192063992168));
#33824=CARTESIAN_POINT('',(61.000349621842,37.9543320991532,36.0864508667399));
#33825=CARTESIAN_POINT('',(60.8668514237356,37.9543320991532,42.084965535481));
#33826=CARTESIAN_POINT('Origin',(60.9336005227888,37.9543320991532,39.0857082011104));
#33827=CARTESIAN_POINT('',(60.9336005227888,34.9543320991532,39.0857082011104));
#33828=CARTESIAN_POINT('Origin',(60.9336005227888,37.9543320991532,39.0857082011104));
#33829=CARTESIAN_POINT('',(66.9321151915299,34.9543320991532,39.2192063992168));
#33830=CARTESIAN_POINT('',(66.9321151915299,34.9543320991532,39.2192063992168));
#33831=CARTESIAN_POINT('Origin',(66.9321151915299,37.9543320991532,39.2192063992168));
#33832=CARTESIAN_POINT('Origin',(60.9336005227888,37.9543320991532,39.0857082011104));
#33833=CARTESIAN_POINT('Origin',(43.4824321383293,37.9543320991532,36.6968335670531));
#33834=CARTESIAN_POINT('',(39.233484247971,37.9543320991532,36.6022723433944));
#33835=CARTESIAN_POINT('Origin',(43.4824321383293,37.9543320991532,36.6968335670531));
#33836=CARTESIAN_POINT('',(39.122235749549,37.9543320991532,41.6010345673453));
#33837=CARTESIAN_POINT('',(39.233484247971,37.9543320991532,36.6022723433944));
#33838=CARTESIAN_POINT('Origin',(43.3711836399073,37.9543320991532,41.695595791004));
#33839=CARTESIAN_POINT('Origin',(35.9397894030341,43.9543320991532,38.5294657090004));
#33840=CARTESIAN_POINT('',(37.1394923367823,33.9543320991532,38.5561653486217));
#33841=CARTESIAN_POINT('Origin',(35.9397894030341,33.9543320991532,38.5294657090004));
#33842=CARTESIAN_POINT('',(37.1394923367823,31.9543320991532,38.5561653486217));
#33843=CARTESIAN_POINT('',(37.1394923367823,43.9543320991532,38.5561653486217));
#33844=CARTESIAN_POINT('Origin',(35.9397894030341,31.9543320991532,38.5294657090004));
#33845=CARTESIAN_POINT('Origin',(35.9397894030341,43.9543320991532,38.5294657090004));
#33846=CARTESIAN_POINT('',(37.1394923367823,43.9543320991532,38.5561653486217));
#33847=CARTESIAN_POINT('Origin',(35.9397894030341,43.9543320991532,38.5294657090004));
#33848=CARTESIAN_POINT('',(37.1394923367823,41.9543320991532,38.5561653486217));
#33849=CARTESIAN_POINT('',(37.1394923367823,43.9543320991532,38.5561653486217));
#33850=CARTESIAN_POINT('Origin',(35.9397894030341,41.9543320991532,38.5294657090004));
#33851=CARTESIAN_POINT('Origin',(43.5046818380137,37.9543320991532,35.6970811222629));
#33852=CARTESIAN_POINT('',(41.5051769484333,37.9543320991532,35.6525817228941));
#33853=CARTESIAN_POINT('Origin',(43.5046818380137,37.9543320991532,35.6970811222629));
#33854=CARTESIAN_POINT('',(41.4829272487489,37.9543320991532,36.6523341676843));
#33855=CARTESIAN_POINT('',(41.5051769484333,37.9543320991532,35.6525817228941));
#33856=CARTESIAN_POINT('Origin',(43.4824321383293,37.9543320991532,36.6968335670531));
#33857=CARTESIAN_POINT('Origin',(60.8668514237356,43.9543320991532,42.084965535481));
#33858=CARTESIAN_POINT('',(61.000349621842,43.9543320991532,36.0864508667399));
#33859=CARTESIAN_POINT('',(61.000349621842,43.9543320991532,36.0864508667399));
#33860=CARTESIAN_POINT('',(60.8668514237356,43.9543320991532,42.084965535481));
#33861=CARTESIAN_POINT('',(60.8668514237356,43.9543320991532,42.084965535481));
#33862=CARTESIAN_POINT('',(60.8668514237356,43.9543320991532,42.084965535481));
#33863=CARTESIAN_POINT('Origin',(34.4735352853754,43.9543320991532,36.9964624922886));
#33864=CARTESIAN_POINT('',(34.506909834902,43.9543320991532,35.4968338251033));
#33865=CARTESIAN_POINT('',(34.506909834902,41.9543320991532,35.4968338251033));
#33866=CARTESIAN_POINT('',(34.506909834902,43.9543320991532,35.4968338251033));
#33867=CARTESIAN_POINT('',(32.9739066181901,41.9543320991532,36.963087942762));
#33868=CARTESIAN_POINT('Origin',(34.4735352853754,41.9543320991532,36.9964624922886));
#33869=CARTESIAN_POINT('',(32.9739066181901,43.9543320991532,36.963087942762));
#33870=CARTESIAN_POINT('',(32.9739066181901,43.9543320991532,36.963087942762));
#33871=CARTESIAN_POINT('Origin',(34.4735352853754,43.9543320991532,36.9964624922886));
#33872=CARTESIAN_POINT('Origin',(32.8737829696103,43.9543320991532,41.4619739443178));
#33873=CARTESIAN_POINT('',(32.8737829696103,41.9543320991532,41.4619739443178));
#33874=CARTESIAN_POINT('',(32.8737829696103,41.9543320991532,41.4619739443178));
#33875=CARTESIAN_POINT('',(32.8737829696103,43.9543320991532,41.4619739443178));
#33876=CARTESIAN_POINT('',(32.8737829696103,43.9543320991532,41.4619739443178));
#33877=CARTESIAN_POINT('',(32.8737829696103,43.9543320991532,41.4619739443178));
#33878=CARTESIAN_POINT('Origin',(34.4735352853754,43.9543320991532,36.9964624922886));
#33879=CARTESIAN_POINT('',(34.506909834902,43.9543320991532,35.4968338251033));
#33880=CARTESIAN_POINT('',(32.8737829696103,43.9543320991532,41.4619739443178));
#33881=CARTESIAN_POINT('Origin',(34.4735352853754,31.9543320991532,36.9964624922886));
#33882=CARTESIAN_POINT('',(60.8668514237356,31.9543320991532,42.084965535481));
#33883=CARTESIAN_POINT('',(61.000349621842,31.9543320991532,36.0864508667399));
#33884=CARTESIAN_POINT('',(60.8668514237356,31.9543320991532,42.084965535481));
#33885=CARTESIAN_POINT('',(32.8737829696103,31.9543320991532,41.4619739443178));
#33886=CARTESIAN_POINT('',(32.8737829696103,31.9543320991532,41.4619739443178));
#33887=CARTESIAN_POINT('',(32.9739066181901,31.9543320991532,36.963087942762));
#33888=CARTESIAN_POINT('',(32.8737829696103,31.9543320991532,41.4619739443178));
#33889=CARTESIAN_POINT('',(34.506909834902,31.9543320991532,35.4968338251033));
#33890=CARTESIAN_POINT('Origin',(34.4735352853754,31.9543320991532,36.9964624922886));
#33891=CARTESIAN_POINT('',(34.506909834902,31.9543320991532,35.4968338251033));
#33892=CARTESIAN_POINT('Origin',(60.8668514237356,43.9543320991532,42.084965535481));
#33893=CARTESIAN_POINT('',(60.8668514237356,43.9543320991532,42.084965535481));
#33894=CARTESIAN_POINT('',(61.000349621842,43.9543320991532,36.0864508667399));
#33895=CARTESIAN_POINT('Origin',(34.506909834902,43.9543320991532,35.4968338251033));
#33896=CARTESIAN_POINT('',(38.5059196140628,41.9543320991532,35.5858326238409));
#33897=CARTESIAN_POINT('',(38.5059196140628,33.9543320991532,35.5858326238409));
#33898=CARTESIAN_POINT('',(38.5059196140628,33.9543320991532,35.5858326238409));
#33899=CARTESIAN_POINT('',(30.5079000557413,41.9543320991532,35.4078350263657));
#33900=CARTESIAN_POINT('',(34.506909834902,33.9543320991532,35.4968338251033));
#33901=CARTESIAN_POINT('',(34.506909834902,43.9543320991532,35.4968338251033));
#33902=CARTESIAN_POINT('',(30.5079000557413,33.9543320991532,35.4078350263657));
#33903=CARTESIAN_POINT('Origin',(34.4735352853754,43.9543320991532,36.9964624922886));
#33904=CARTESIAN_POINT('',(32.9739066181901,33.9543320991532,36.963087942762));
#33905=CARTESIAN_POINT('',(32.9739066181901,43.9543320991532,36.963087942762));
#33906=CARTESIAN_POINT('Origin',(34.4735352853754,33.9543320991532,36.9964624922886));
#33907=CARTESIAN_POINT('Origin',(32.8737829696103,43.9543320991532,41.4619739443178));
#33908=CARTESIAN_POINT('',(32.8737829696103,33.9543320991532,41.4619739443178));
#33909=CARTESIAN_POINT('',(32.8737829696103,43.9543320991532,41.4619739443178));
#33910=CARTESIAN_POINT('',(32.8737829696103,33.9543320991532,41.4619739443178));
#33911=CARTESIAN_POINT('Origin',(32.8737829696103,43.9543320991532,41.4619739443178));
#33912=CARTESIAN_POINT('',(38.3724214159564,41.9543320991532,41.584347292582));
#33913=CARTESIAN_POINT('',(30.3744018576349,41.9543320991532,41.4063496951068));
#33914=CARTESIAN_POINT('',(38.3724214159564,33.9543320991532,41.584347292582));
#33915=CARTESIAN_POINT('',(38.3724214159564,33.9543320991532,41.584347292582));
#33916=CARTESIAN_POINT('',(30.3744018576349,33.9543320991532,41.4063496951068));
#33917=CARTESIAN_POINT('Origin',(30.3744018576349,41.9543320991532,41.4063496951068));
#33918=CARTESIAN_POINT('',(38.3724214159564,41.9543320991532,41.584347292582));
#33919=CARTESIAN_POINT('Origin',(30.3744018576349,33.9543320991532,41.4063496951068));
#33920=CARTESIAN_POINT('',(38.3724214159564,33.9543320991532,41.584347292582));
#33921=CARTESIAN_POINT('Origin',(38.3724214159564,33.9543320991532,41.584347292582));
#33922=CARTESIAN_POINT('Origin',(43.4824321383293,37.9543320991532,36.6968335670531));
#33923=CARTESIAN_POINT('Origin',(66.9321151915299,37.9543320991532,39.2192063992168));
#33924=CARTESIAN_POINT('Origin',(71.9308774154808,37.9543320991532,39.3304548976388));
#33925=CARTESIAN_POINT('Origin',(83.7526213271442,37.9543320991532,39.5935502800518));
#33926=CARTESIAN_POINT('',(66.9872301765546,38.2918510578248,36.7427082080277));
#33927=CARTESIAN_POINT('Origin',(66.93211519153,37.9543320991532,39.2192063992168));
#33928=CARTESIAN_POINT('',(71.9859924005056,38.2918510578248,36.8539567064497));
#33929=CARTESIAN_POINT('',(83.8077363121688,38.2918510578248,37.1170520888627));
#33930=CARTESIAN_POINT('Origin',(71.930877415481,37.9543320991532,39.3304548976388));
#33931=CARTESIAN_POINT('Origin',(71.829881909202,37.9543320991532,39.3282072215307));
#33932=CARTESIAN_POINT('',(71.8133605791719,43.4039772078075,40.0705651105397));
#33933=CARTESIAN_POINT('',(71.8464032392321,32.5046869904988,38.5858493325217));
#33934=CARTESIAN_POINT('Origin',(71.829881909202,37.9543320991532,39.3282072215307));
#33935=CARTESIAN_POINT('Origin',(71.930877415481,37.9543320991532,39.3304548976388));
#33936=CARTESIAN_POINT('Origin',(54.9397894030341,37.9543320991532,23.5294657090004));
#33937=CARTESIAN_POINT('',(57.4397894030341,37.9543320991532,23.0294657090004));
#33938=CARTESIAN_POINT('Origin',(54.9397894030341,37.9543320991532,23.0294657090004));
#33939=CARTESIAN_POINT('',(56.9397894030341,37.9543320991532,23.5294657090004));
#33940=CARTESIAN_POINT('Origin',(57.4397894030341,37.9543320991532,23.5294657090004));
#33941=CARTESIAN_POINT('Origin',(54.9397894030341,37.9543320991532,23.5294657090004));
#33942=CARTESIAN_POINT('Origin',(54.9397894030341,37.9543320991532,34.6394657090004));
#33943=CARTESIAN_POINT('',(54.9397894030341,35.9561834064188,34.6413170162659));
#33944=CARTESIAN_POINT('',(56.9379380957686,37.9543320991532,34.6413170162659));
#33945=CARTESIAN_POINT('Origin',(54.9397894030341,37.9543320991532,34.6413170162659));
#33946=CARTESIAN_POINT('Origin',(54.9397894030341,37.9543320991532,34.6413170162659));
#33947=CARTESIAN_POINT('',(56.5497894030341,37.9543320991532,35.0294657090004));
#33948=CARTESIAN_POINT('',(56.9397894030341,37.9543320991532,34.6394657090004));
#33949=CARTESIAN_POINT('Origin',(54.9397894030341,37.9543320991532,35.0294657090004));
#33950=CARTESIAN_POINT('Origin',(54.9397894030341,37.9543320991532,34.369532375667));
#33951=CARTESIAN_POINT('',(56.9397894030342,37.9543320991532,34.0964514357652));
#33952=CARTESIAN_POINT('',(54.9397894030341,39.9543320991532,34.0964514357652));
#33953=CARTESIAN_POINT('Origin',(54.9397894030341,37.9543320991532,34.0964514357652));
#33954=CARTESIAN_POINT('Origin',(54.9397894030341,37.9543320991532,34.0964514357652));
#33955=CARTESIAN_POINT('',(54.9397894030341,39.5643320991532,34.369532375667));
#33956=CARTESIAN_POINT('',(54.9397894030341,39.5643320991532,34.369532375667));
#33957=CARTESIAN_POINT('',(54.9397894030341,36.3443320991532,34.369532375667));
#33958=CARTESIAN_POINT('Origin',(54.9397894030341,37.9543320991532,34.369532375667));
#33959=CARTESIAN_POINT('Origin',(54.9397894030341,37.9543320991532,34.369532375667));
#33960=CARTESIAN_POINT('Origin',(54.9397894030341,37.9543320991532,34.6426133155688));
#33961=CARTESIAN_POINT('',(54.9397894030341,35.9543320991532,34.6426133155688));
#33962=CARTESIAN_POINT('Origin',(54.9397894030341,37.9543320991532,8.12867690713751));
#33963=CARTESIAN_POINT('',(54.9397894030341,35.9543320991532,33.9826799822355));
#33964=CARTESIAN_POINT('',(56.9397894030342,37.9543320991532,33.9826799822355));
#33965=CARTESIAN_POINT('Origin',(54.9397894030341,37.9543320991532,33.9826799822355));
#33966=CARTESIAN_POINT('Origin',(54.9397894030341,37.9543320991532,33.9826799822355));
#33967=CARTESIAN_POINT('',(56.9397894030341,37.9543320991532,8.12867690713751));
#33968=CARTESIAN_POINT('Origin',(54.9397894030341,37.9543320991532,33.7095990423337));
#33969=CARTESIAN_POINT('',(56.9397894030342,37.9543320991532,33.4365181024319));
#33970=CARTESIAN_POINT('',(54.9397894030341,39.9543320991532,33.4365181024319));
#33971=CARTESIAN_POINT('Origin',(54.9397894030341,37.9543320991532,33.4365181024319));
#33972=CARTESIAN_POINT('Origin',(54.9397894030341,37.9543320991532,33.4365181024319));
#33973=CARTESIAN_POINT('',(54.9397894030341,39.5643320991532,33.7095990423337));
#33974=CARTESIAN_POINT('',(54.9397894030341,39.5643320991532,33.7095990423337));
#33975=CARTESIAN_POINT('',(54.9397894030341,36.3443320991532,33.7095990423337));
#33976=CARTESIAN_POINT('Origin',(54.9397894030341,37.9543320991532,33.7095990423337));
#33977=CARTESIAN_POINT('Origin',(54.9397894030341,37.9543320991532,33.7095990423337));
#33978=CARTESIAN_POINT('Origin',(54.9397894030341,37.9543320991532,33.9826799822355));
#33979=CARTESIAN_POINT('',(54.9397894030341,35.9543320991532,33.9826799822355));
#33980=CARTESIAN_POINT('Origin',(54.9397894030341,37.9543320991532,8.12867690713751));
#33981=CARTESIAN_POINT('',(54.9397894030341,35.9543320991532,33.3227466489021));
#33982=CARTESIAN_POINT('',(56.9397894030342,37.9543320991532,33.3227466489021));
#33983=CARTESIAN_POINT('Origin',(54.9397894030341,37.9543320991532,33.3227466489021));
#33984=CARTESIAN_POINT('Origin',(54.9397894030341,37.9543320991532,33.3227466489021));
#33985=CARTESIAN_POINT('',(56.9397894030341,37.9543320991532,8.12867690713751));
#33986=CARTESIAN_POINT('Origin',(54.9397894030341,37.9543320991532,33.0496657090004));
#33987=CARTESIAN_POINT('',(56.9397894030342,37.9543320991532,32.7765847690986));
#33988=CARTESIAN_POINT('',(54.9397894030341,39.9543320991532,32.7765847690986));
#33989=CARTESIAN_POINT('Origin',(54.9397894030341,37.9543320991532,32.7765847690986));
#33990=CARTESIAN_POINT('Origin',(54.9397894030341,37.9543320991532,32.7765847690986));
#33991=CARTESIAN_POINT('',(54.9397894030341,39.5643320991532,33.0496657090004));
#33992=CARTESIAN_POINT('',(54.9397894030341,39.5643320991532,33.0496657090004));
#33993=CARTESIAN_POINT('',(54.9397894030341,36.3443320991532,33.0496657090004));
#33994=CARTESIAN_POINT('Origin',(54.9397894030341,37.9543320991532,33.0496657090004));
#33995=CARTESIAN_POINT('Origin',(54.9397894030341,37.9543320991532,33.0496657090004));
#33996=CARTESIAN_POINT('Origin',(54.9397894030341,37.9543320991532,33.3227466489021));
#33997=CARTESIAN_POINT('',(54.9397894030341,35.9543320991532,33.3227466489021));
#33998=CARTESIAN_POINT('Origin',(54.9397894030341,37.9543320991532,8.12867690713751));
#33999=CARTESIAN_POINT('',(54.9397894030341,35.9543320991532,32.6628133155688));
#34000=CARTESIAN_POINT('',(56.9397894030342,37.9543320991532,32.6628133155688));
#34001=CARTESIAN_POINT('Origin',(54.9397894030341,37.9543320991532,32.6628133155688));
#34002=CARTESIAN_POINT('Origin',(54.9397894030341,37.9543320991532,32.6628133155688));
#34003=CARTESIAN_POINT('',(56.9397894030341,37.9543320991532,8.12867690713751));
#34004=CARTESIAN_POINT('Origin',(54.9397894030341,37.9543320991532,32.389732375667));
#34005=CARTESIAN_POINT('',(56.9397894030342,37.9543320991532,32.1166514357652));
#34006=CARTESIAN_POINT('',(54.9397894030341,39.9543320991532,32.1166514357652));
#34007=CARTESIAN_POINT('Origin',(54.9397894030341,37.9543320991532,32.1166514357652));
#34008=CARTESIAN_POINT('Origin',(54.9397894030341,37.9543320991532,32.1166514357652));
#34009=CARTESIAN_POINT('',(54.9397894030341,39.5643320991532,32.389732375667));
#34010=CARTESIAN_POINT('',(54.9397894030341,39.5643320991532,32.389732375667));
#34011=CARTESIAN_POINT('',(54.9397894030341,36.3443320991532,32.389732375667));
#34012=CARTESIAN_POINT('Origin',(54.9397894030341,37.9543320991532,32.389732375667));
#34013=CARTESIAN_POINT('Origin',(54.9397894030341,37.9543320991532,32.389732375667));
#34014=CARTESIAN_POINT('Origin',(54.9397894030341,37.9543320991532,32.6628133155688));
#34015=CARTESIAN_POINT('',(54.9397894030341,35.9543320991532,32.6628133155688));
#34016=CARTESIAN_POINT('Origin',(54.9397894030341,37.9543320991532,8.12867690713751));
#34017=CARTESIAN_POINT('',(54.9397894030341,35.9543320991532,32.0028799822355));
#34018=CARTESIAN_POINT('',(56.9397894030342,37.9543320991532,32.0028799822355));
#34019=CARTESIAN_POINT('Origin',(54.9397894030341,37.9543320991532,32.0028799822355));
#34020=CARTESIAN_POINT('Origin',(54.9397894030341,37.9543320991532,32.0028799822355));
#34021=CARTESIAN_POINT('',(56.9397894030341,37.9543320991532,8.12867690713751));
#34022=CARTESIAN_POINT('Origin',(54.9397894030341,37.9543320991532,31.7297990423337));
#34023=CARTESIAN_POINT('',(56.9397894030342,37.9543320991532,31.4567181024319));
#34024=CARTESIAN_POINT('',(54.9397894030341,39.9543320991532,31.4567181024319));
#34025=CARTESIAN_POINT('Origin',(54.9397894030341,37.9543320991532,31.4567181024319));
#34026=CARTESIAN_POINT('Origin',(54.9397894030341,37.9543320991532,31.4567181024319));
#34027=CARTESIAN_POINT('',(54.9397894030341,39.5643320991532,31.7297990423337));
#34028=CARTESIAN_POINT('',(54.9397894030341,39.5643320991532,31.7297990423337));
#34029=CARTESIAN_POINT('',(54.9397894030341,36.3443320991532,31.7297990423337));
#34030=CARTESIAN_POINT('Origin',(54.9397894030341,37.9543320991532,31.7297990423337));
#34031=CARTESIAN_POINT('Origin',(54.9397894030341,37.9543320991532,31.7297990423337));
#34032=CARTESIAN_POINT('Origin',(54.9397894030341,37.9543320991532,32.0028799822355));
#34033=CARTESIAN_POINT('',(54.9397894030341,35.9543320991532,32.0028799822355));
#34034=CARTESIAN_POINT('Origin',(54.9397894030341,37.9543320991532,8.12867690713751));
#34035=CARTESIAN_POINT('',(54.9397894030341,35.9543320991532,31.3429466489021));
#34036=CARTESIAN_POINT('',(56.9397894030342,37.9543320991532,31.3429466489021));
#34037=CARTESIAN_POINT('Origin',(54.9397894030341,37.9543320991532,31.3429466489021));
#34038=CARTESIAN_POINT('Origin',(54.9397894030341,37.9543320991532,31.3429466489021));
#34039=CARTESIAN_POINT('',(56.9397894030341,37.9543320991532,8.12867690713751));
#34040=CARTESIAN_POINT('Origin',(54.9397894030341,37.9543320991532,31.0698657090004));
#34041=CARTESIAN_POINT('',(56.9397894030342,37.9543320991532,30.7967847690986));
#34042=CARTESIAN_POINT('',(54.9397894030341,39.9543320991532,30.7967847690986));
#34043=CARTESIAN_POINT('Origin',(54.9397894030341,37.9543320991532,30.7967847690986));
#34044=CARTESIAN_POINT('Origin',(54.9397894030341,37.9543320991532,30.7967847690986));
#34045=CARTESIAN_POINT('',(54.9397894030341,39.5643320991532,31.0698657090004));
#34046=CARTESIAN_POINT('',(54.9397894030341,39.5643320991532,31.0698657090004));
#34047=CARTESIAN_POINT('',(54.9397894030341,36.3443320991532,31.0698657090004));
#34048=CARTESIAN_POINT('Origin',(54.9397894030341,37.9543320991532,31.0698657090004));
#34049=CARTESIAN_POINT('Origin',(54.9397894030341,37.9543320991532,31.0698657090004));
#34050=CARTESIAN_POINT('Origin',(54.9397894030341,37.9543320991532,31.3429466489021));
#34051=CARTESIAN_POINT('',(54.9397894030341,35.9543320991532,31.3429466489021));
#34052=CARTESIAN_POINT('Origin',(54.9397894030341,37.9543320991532,8.12867690713751));
#34053=CARTESIAN_POINT('',(54.9397894030341,35.9543320991532,30.6830133155688));
#34054=CARTESIAN_POINT('',(56.9397894030342,37.9543320991532,30.6830133155688));
#34055=CARTESIAN_POINT('Origin',(54.9397894030341,37.9543320991532,30.6830133155688));
#34056=CARTESIAN_POINT('Origin',(54.9397894030341,37.9543320991532,30.6830133155688));
#34057=CARTESIAN_POINT('',(56.9397894030341,37.9543320991532,8.12867690713751));
#34058=CARTESIAN_POINT('Origin',(54.9397894030341,37.9543320991532,30.409932375667));
#34059=CARTESIAN_POINT('',(56.9397894030342,37.9543320991532,30.1368514357652));
#34060=CARTESIAN_POINT('',(54.9397894030341,39.9543320991532,30.1368514357652));
#34061=CARTESIAN_POINT('Origin',(54.9397894030341,37.9543320991532,30.1368514357652));
#34062=CARTESIAN_POINT('Origin',(54.9397894030341,37.9543320991532,30.1368514357652));
#34063=CARTESIAN_POINT('',(54.9397894030341,39.5643320991532,30.409932375667));
#34064=CARTESIAN_POINT('',(54.9397894030341,39.5643320991532,30.409932375667));
#34065=CARTESIAN_POINT('',(54.9397894030341,36.3443320991532,30.409932375667));
#34066=CARTESIAN_POINT('Origin',(54.9397894030341,37.9543320991532,30.409932375667));
#34067=CARTESIAN_POINT('Origin',(54.9397894030341,37.9543320991532,30.409932375667));
#34068=CARTESIAN_POINT('Origin',(54.9397894030341,37.9543320991532,30.6830133155688));
#34069=CARTESIAN_POINT('',(54.9397894030341,35.9543320991532,30.6830133155688));
#34070=CARTESIAN_POINT('Origin',(54.9397894030341,37.9543320991532,8.12867690713751));
#34071=CARTESIAN_POINT('',(54.9397894030341,35.9543320991532,30.0230799822355));
#34072=CARTESIAN_POINT('',(56.9397894030342,37.9543320991532,30.0230799822355));
#34073=CARTESIAN_POINT('Origin',(54.9397894030341,37.9543320991532,30.0230799822355));
#34074=CARTESIAN_POINT('Origin',(54.9397894030341,37.9543320991532,30.0230799822355));
#34075=CARTESIAN_POINT('',(56.9397894030341,37.9543320991532,8.12867690713751));
#34076=CARTESIAN_POINT('Origin',(54.9397894030341,37.9543320991532,29.7499990423337));
#34077=CARTESIAN_POINT('',(56.9397894030342,37.9543320991532,29.4769181024319));
#34078=CARTESIAN_POINT('',(54.9397894030341,39.9543320991532,29.4769181024319));
#34079=CARTESIAN_POINT('Origin',(54.9397894030341,37.9543320991532,29.4769181024319));
#34080=CARTESIAN_POINT('Origin',(54.9397894030341,37.9543320991532,29.4769181024319));
#34081=CARTESIAN_POINT('',(54.9397894030341,39.5643320991532,29.7499990423337));
#34082=CARTESIAN_POINT('',(54.9397894030341,39.5643320991532,29.7499990423337));
#34083=CARTESIAN_POINT('',(54.9397894030341,36.3443320991532,29.7499990423337));
#34084=CARTESIAN_POINT('Origin',(54.9397894030341,37.9543320991532,29.7499990423337));
#34085=CARTESIAN_POINT('Origin',(54.9397894030341,37.9543320991532,29.7499990423337));
#34086=CARTESIAN_POINT('Origin',(54.9397894030341,37.9543320991532,30.0230799822355));
#34087=CARTESIAN_POINT('',(54.9397894030341,35.9543320991532,30.0230799822355));
#34088=CARTESIAN_POINT('Origin',(54.9397894030341,37.9543320991532,8.12867690713751));
#34089=CARTESIAN_POINT('',(54.9397894030341,35.9543320991532,29.3631466489021));
#34090=CARTESIAN_POINT('',(56.9397894030342,37.9543320991532,29.3631466489021));
#34091=CARTESIAN_POINT('Origin',(54.9397894030341,37.9543320991532,29.3631466489021));
#34092=CARTESIAN_POINT('Origin',(54.9397894030341,37.9543320991532,29.3631466489021));
#34093=CARTESIAN_POINT('',(56.9397894030341,37.9543320991532,8.12867690713751));
#34094=CARTESIAN_POINT('Origin',(54.9397894030341,37.9543320991532,29.0900657090004));
#34095=CARTESIAN_POINT('',(56.9397894030342,37.9543320991532,28.8169847690986));
#34096=CARTESIAN_POINT('',(54.9397894030341,39.9543320991532,28.8169847690986));
#34097=CARTESIAN_POINT('Origin',(54.9397894030341,37.9543320991532,28.8169847690986));
#34098=CARTESIAN_POINT('Origin',(54.9397894030341,37.9543320991532,28.8169847690986));
#34099=CARTESIAN_POINT('',(54.9397894030341,39.5643320991532,29.0900657090004));
#34100=CARTESIAN_POINT('',(54.9397894030341,39.5643320991532,29.0900657090004));
#34101=CARTESIAN_POINT('',(54.9397894030341,36.3443320991532,29.0900657090004));
#34102=CARTESIAN_POINT('Origin',(54.9397894030341,37.9543320991532,29.0900657090004));
#34103=CARTESIAN_POINT('Origin',(54.9397894030341,37.9543320991532,29.0900657090004));
#34104=CARTESIAN_POINT('Origin',(54.9397894030341,37.9543320991532,29.3631466489021));
#34105=CARTESIAN_POINT('',(54.9397894030341,35.9543320991532,29.3631466489021));
#34106=CARTESIAN_POINT('Origin',(54.9397894030341,37.9543320991532,8.12867690713751));
#34107=CARTESIAN_POINT('',(54.9397894030341,35.9543320991532,28.7032133155688));
#34108=CARTESIAN_POINT('',(56.9397894030342,37.9543320991532,28.7032133155688));
#34109=CARTESIAN_POINT('Origin',(54.9397894030341,37.9543320991532,28.7032133155688));
#34110=CARTESIAN_POINT('Origin',(54.9397894030341,37.9543320991532,28.7032133155688));
#34111=CARTESIAN_POINT('',(56.9397894030341,37.9543320991532,8.12867690713751));
#34112=CARTESIAN_POINT('Origin',(54.9397894030341,37.9543320991532,28.430132375667));
#34113=CARTESIAN_POINT('',(56.9397894030342,37.9543320991532,28.1570514357652));
#34114=CARTESIAN_POINT('',(54.9397894030341,39.9543320991532,28.1570514357652));
#34115=CARTESIAN_POINT('Origin',(54.9397894030341,37.9543320991532,28.1570514357652));
#34116=CARTESIAN_POINT('Origin',(54.9397894030341,37.9543320991532,28.1570514357652));
#34117=CARTESIAN_POINT('',(54.9397894030341,39.5643320991532,28.430132375667));
#34118=CARTESIAN_POINT('',(54.9397894030341,39.5643320991532,28.430132375667));
#34119=CARTESIAN_POINT('',(54.9397894030341,36.3443320991532,28.430132375667));
#34120=CARTESIAN_POINT('Origin',(54.9397894030341,37.9543320991532,28.430132375667));
#34121=CARTESIAN_POINT('Origin',(54.9397894030341,37.9543320991532,28.430132375667));
#34122=CARTESIAN_POINT('Origin',(54.9397894030341,37.9543320991532,28.7032133155688));
#34123=CARTESIAN_POINT('',(54.9397894030341,35.9543320991532,28.7032133155688));
#34124=CARTESIAN_POINT('Origin',(54.9397894030341,37.9543320991532,8.12867690713751));
#34125=CARTESIAN_POINT('',(54.9397894030341,35.9543320991532,28.0432799822355));
#34126=CARTESIAN_POINT('',(56.9397894030342,37.9543320991532,28.0432799822355));
#34127=CARTESIAN_POINT('Origin',(54.9397894030341,37.9543320991532,28.0432799822355));
#34128=CARTESIAN_POINT('Origin',(54.9397894030341,37.9543320991532,28.0432799822355));
#34129=CARTESIAN_POINT('',(56.9397894030341,37.9543320991532,8.12867690713751));
#34130=CARTESIAN_POINT('Origin',(54.9397894030341,37.9543320991532,27.7701990423337));
#34131=CARTESIAN_POINT('',(56.9397894030342,37.9543320991532,27.4971181024319));
#34132=CARTESIAN_POINT('',(54.9397894030341,39.9543320991532,27.4971181024319));
#34133=CARTESIAN_POINT('Origin',(54.9397894030341,37.9543320991532,27.4971181024319));
#34134=CARTESIAN_POINT('Origin',(54.9397894030341,37.9543320991532,27.4971181024319));
#34135=CARTESIAN_POINT('',(54.9397894030341,39.5643320991532,27.7701990423337));
#34136=CARTESIAN_POINT('',(54.9397894030341,39.5643320991532,27.7701990423337));
#34137=CARTESIAN_POINT('',(54.9397894030341,36.3443320991532,27.7701990423337));
#34138=CARTESIAN_POINT('Origin',(54.9397894030341,37.9543320991532,27.7701990423337));
#34139=CARTESIAN_POINT('Origin',(54.9397894030341,37.9543320991532,27.7701990423337));
#34140=CARTESIAN_POINT('Origin',(54.9397894030341,37.9543320991532,28.0432799822355));
#34141=CARTESIAN_POINT('',(54.9397894030341,35.9543320991532,28.0432799822355));
#34142=CARTESIAN_POINT('Origin',(54.9397894030341,37.9543320991532,8.12867690713751));
#34143=CARTESIAN_POINT('',(54.9397894030341,35.9543320991532,27.3833466489021));
#34144=CARTESIAN_POINT('',(56.9397894030342,37.9543320991532,27.3833466489021));
#34145=CARTESIAN_POINT('Origin',(54.9397894030341,37.9543320991532,27.3833466489021));
#34146=CARTESIAN_POINT('Origin',(54.9397894030341,37.9543320991532,27.3833466489021));
#34147=CARTESIAN_POINT('',(56.9397894030341,37.9543320991532,8.12867690713751));
#34148=CARTESIAN_POINT('Origin',(54.9397894030341,37.9543320991532,27.1102657090004));
#34149=CARTESIAN_POINT('',(56.9397894030342,37.9543320991532,26.8371847690986));
#34150=CARTESIAN_POINT('',(54.9397894030341,39.9543320991532,26.8371847690986));
#34151=CARTESIAN_POINT('Origin',(54.9397894030341,37.9543320991532,26.8371847690986));
#34152=CARTESIAN_POINT('Origin',(54.9397894030341,37.9543320991532,26.8371847690986));
#34153=CARTESIAN_POINT('',(54.9397894030341,39.5643320991532,27.1102657090004));
#34154=CARTESIAN_POINT('',(54.9397894030341,39.5643320991532,27.1102657090004));
#34155=CARTESIAN_POINT('',(54.9397894030341,36.3443320991532,27.1102657090004));
#34156=CARTESIAN_POINT('Origin',(54.9397894030341,37.9543320991532,27.1102657090004));
#34157=CARTESIAN_POINT('Origin',(54.9397894030341,37.9543320991532,27.1102657090004));
#34158=CARTESIAN_POINT('Origin',(54.9397894030341,37.9543320991532,27.3833466489021));
#34159=CARTESIAN_POINT('',(54.9397894030341,35.9543320991532,27.3833466489021));
#34160=CARTESIAN_POINT('Origin',(54.9397894030341,37.9543320991532,8.12867690713751));
#34161=CARTESIAN_POINT('',(54.9397894030341,35.9543320991532,26.7234133155688));
#34162=CARTESIAN_POINT('',(56.9397894030342,37.9543320991532,26.7234133155688));
#34163=CARTESIAN_POINT('Origin',(54.9397894030341,37.9543320991532,26.7234133155688));
#34164=CARTESIAN_POINT('Origin',(54.9397894030341,37.9543320991532,26.7234133155688));
#34165=CARTESIAN_POINT('',(56.9397894030341,37.9543320991532,8.12867690713751));
#34166=CARTESIAN_POINT('Origin',(54.9397894030341,37.9543320991532,26.450332375667));
#34167=CARTESIAN_POINT('',(56.9397894030341,37.9543320991532,26.1772514357652));
#34168=CARTESIAN_POINT('',(54.9397894030341,39.9543320991532,26.1772514357652));
#34169=CARTESIAN_POINT('Origin',(54.9397894030341,37.9543320991532,26.1772514357652));
#34170=CARTESIAN_POINT('Origin',(54.9397894030341,37.9543320991532,26.1772514357652));
#34171=CARTESIAN_POINT('',(54.9397894030341,39.5643320991532,26.450332375667));
#34172=CARTESIAN_POINT('',(54.9397894030341,39.5643320991532,26.450332375667));
#34173=CARTESIAN_POINT('',(54.9397894030341,36.3443320991532,26.450332375667));
#34174=CARTESIAN_POINT('Origin',(54.9397894030341,37.9543320991532,26.450332375667));
#34175=CARTESIAN_POINT('Origin',(54.9397894030341,37.9543320991532,26.450332375667));
#34176=CARTESIAN_POINT('Origin',(54.9397894030341,37.9543320991532,26.7234133155688));
#34177=CARTESIAN_POINT('',(54.9397894030341,35.9543320991532,26.7234133155688));
#34178=CARTESIAN_POINT('Origin',(54.9397894030341,37.9543320991532,8.12867690713751));
#34179=CARTESIAN_POINT('',(54.9397894030341,35.9543320991532,26.0634799822355));
#34180=CARTESIAN_POINT('',(56.9397894030341,37.9543320991532,26.0634799822355));
#34181=CARTESIAN_POINT('Origin',(54.9397894030341,37.9543320991532,26.0634799822355));
#34182=CARTESIAN_POINT('Origin',(54.9397894030341,37.9543320991532,26.0634799822355));
#34183=CARTESIAN_POINT('',(56.9397894030341,37.9543320991532,8.12867690713751));
#34184=CARTESIAN_POINT('Origin',(54.9397894030341,37.9543320991532,25.7903990423337));
#34185=CARTESIAN_POINT('',(56.9397894030341,37.9543320991532,25.5173181024319));
#34186=CARTESIAN_POINT('',(54.9397894030341,39.9543320991532,25.5173181024319));
#34187=CARTESIAN_POINT('Origin',(54.9397894030341,37.9543320991532,25.5173181024319));
#34188=CARTESIAN_POINT('Origin',(54.9397894030341,37.9543320991532,25.5173181024319));
#34189=CARTESIAN_POINT('',(54.9397894030341,39.5643320991532,25.7903990423337));
#34190=CARTESIAN_POINT('',(54.9397894030341,39.5643320991532,25.7903990423337));
#34191=CARTESIAN_POINT('',(54.9397894030341,36.3443320991532,25.7903990423337));
#34192=CARTESIAN_POINT('Origin',(54.9397894030341,37.9543320991532,25.7903990423337));
#34193=CARTESIAN_POINT('Origin',(54.9397894030341,37.9543320991532,25.7903990423337));
#34194=CARTESIAN_POINT('Origin',(54.9397894030341,37.9543320991532,26.0634799822355));
#34195=CARTESIAN_POINT('',(54.9397894030341,35.9543320991532,26.0634799822355));
#34196=CARTESIAN_POINT('Origin',(54.9397894030341,37.9543320991532,8.12867690713751));
#34197=CARTESIAN_POINT('',(54.9397894030341,35.9543320991532,25.4035466489021));
#34198=CARTESIAN_POINT('',(56.9397894030341,37.9543320991532,25.4035466489021));
#34199=CARTESIAN_POINT('Origin',(54.9397894030341,37.9543320991532,25.4035466489021));
#34200=CARTESIAN_POINT('Origin',(54.9397894030341,37.9543320991532,25.4035466489021));
#34201=CARTESIAN_POINT('',(56.9397894030341,37.9543320991532,8.12867690713751));
#34202=CARTESIAN_POINT('Origin',(54.9397894030341,37.9543320991532,25.1304657090004));
#34203=CARTESIAN_POINT('',(56.9397894030341,37.9543320991532,24.8573847690986));
#34204=CARTESIAN_POINT('',(54.9397894030341,39.9543320991532,24.8573847690986));
#34205=CARTESIAN_POINT('Origin',(54.9397894030341,37.9543320991532,24.8573847690986));
#34206=CARTESIAN_POINT('Origin',(54.9397894030341,37.9543320991532,24.8573847690986));
#34207=CARTESIAN_POINT('',(54.9397894030341,39.5643320991532,25.1304657090004));
#34208=CARTESIAN_POINT('',(54.9397894030341,39.5643320991532,25.1304657090004));
#34209=CARTESIAN_POINT('',(54.9397894030341,36.3443320991532,25.1304657090004));
#34210=CARTESIAN_POINT('Origin',(54.9397894030341,37.9543320991532,25.1304657090004));
#34211=CARTESIAN_POINT('Origin',(54.9397894030341,37.9543320991532,25.1304657090004));
#34212=CARTESIAN_POINT('Origin',(54.9397894030341,37.9543320991532,25.4035466489021));
#34213=CARTESIAN_POINT('',(54.9397894030341,35.9543320991532,25.4035466489021));
#34214=CARTESIAN_POINT('Origin',(54.9397894030341,37.9543320991532,19.9294657090004));
#34215=CARTESIAN_POINT('',(63.1147876185643,37.9489306105332,19.9294657090004));
#34216=CARTESIAN_POINT('',(62.8131508375241,38.1149705811106,19.6294657090004));
#34217=CARTESIAN_POINT('Ctrl Pts',(63.1147876185643,37.9489306105332,19.9294657090003));
#34218=CARTESIAN_POINT('Ctrl Pts',(62.9611501927074,38.0335023712479,19.7757724373647));
#34219=CARTESIAN_POINT('Ctrl Pts',(62.8131508375241,38.1149705811106,19.6294657090003));
#34220=CARTESIAN_POINT('',(63.1082046987747,37.6262824743835,19.9294657090004));
#34221=CARTESIAN_POINT('Origin',(54.9397894030341,37.9543320991532,19.9294657090004));
#34222=CARTESIAN_POINT('',(62.8000464044319,37.4726840201813,19.6294657090004));
#34223=CARTESIAN_POINT('Ctrl Pts',(62.8000464044319,37.4726840201813,19.6294657090003));
#34224=CARTESIAN_POINT('Ctrl Pts',(62.951245567544,37.5480477477104,19.7757724373647));
#34225=CARTESIAN_POINT('Ctrl Pts',(63.1082046987747,37.6262824743835,19.9294657090003));
#34226=CARTESIAN_POINT('',(63.0871457149245,37.2826103359947,19.9294657090004));
#34227=CARTESIAN_POINT('Ctrl Pts',(63.0871457149245,37.2826103359947,19.9294657090003));
#34228=CARTESIAN_POINT('Ctrl Pts',(62.9409128885521,37.3794235676598,19.7757724373647));
#34229=CARTESIAN_POINT('Ctrl Pts',(62.8000464044319,37.4726840201813,19.6294657090004));
#34230=CARTESIAN_POINT('',(63.0542858808421,36.9615723539771,19.9294657090004));
#34231=CARTESIAN_POINT('Origin',(54.9397894030341,37.9543320991532,19.9294657090004));
#34232=CARTESIAN_POINT('',(62.7346332578465,36.8336027477512,19.6294657090004));
#34233=CARTESIAN_POINT('Ctrl Pts',(62.7346332578465,36.8336027477512,19.6294657090003));
#34234=CARTESIAN_POINT('Ctrl Pts',(62.8914721616528,36.8963915732358,19.7757724373647));
#34235=CARTESIAN_POINT('Ctrl Pts',(63.0542858808421,36.9615723539771,19.9294657090003));
#34236=CARTESIAN_POINT('',(63.0052844992482,36.6207602589636,19.9294657090004));
#34237=CARTESIAN_POINT('Ctrl Pts',(63.0052844992482,36.6207602589636,19.9294657090003));
#34238=CARTESIAN_POINT('Ctrl Pts',(62.8674294276931,36.7291706854956,19.7757724373646));
#34239=CARTESIAN_POINT('Ctrl Pts',(62.7346332578465,36.8336027477512,19.6294657090003));
#34240=CARTESIAN_POINT('',(62.9463664276474,36.3034688858809,19.9294657090004));
#34241=CARTESIAN_POINT('Origin',(54.9397894030341,37.9543320991532,19.9294657090004));
#34242=CARTESIAN_POINT('',(62.617346711466,36.2019797442473,19.6294657090004));
#34243=CARTESIAN_POINT('Ctrl Pts',(62.617346711466,36.2019797442473,19.6294657090004));
#34244=CARTESIAN_POINT('Ctrl Pts',(62.7787816189382,36.2517758184133,19.7757724373647));
#34245=CARTESIAN_POINT('Ctrl Pts',(62.9463664276474,36.3034688858809,19.9294657090003));
#34246=CARTESIAN_POINT('',(62.8697487444197,35.9677848825051,19.9294657090004));
#34247=CARTESIAN_POINT('Ctrl Pts',(62.8697487444197,35.9677848825052,19.9294657090003));
#34248=CARTESIAN_POINT('Ctrl Pts',(62.7411888304386,36.0870710504019,19.7757724373647));
#34249=CARTESIAN_POINT('Ctrl Pts',(62.617346711466,36.2019797442473,19.6294657090004));
#34250=CARTESIAN_POINT('',(62.785164525346,35.6563516400959,19.9294657090004));
#34251=CARTESIAN_POINT('Origin',(54.9397894030341,37.9543320991532,19.9294657090004));
#34252=CARTESIAN_POINT('',(62.4489672879057,35.5820183565476,19.6294657090004));
#34253=CARTESIAN_POINT('Ctrl Pts',(62.4489672879057,35.5820183565476,19.6294657090004));
#34254=CARTESIAN_POINT('Ctrl Pts',(62.6139238763694,35.6184902947372,19.7757724373647));
#34255=CARTESIAN_POINT('Ctrl Pts',(62.785164525346,35.6563516400959,19.9294657090003));
#34256=CARTESIAN_POINT('',(62.6814404185254,35.3280296500162,19.9294657090004));
#34257=CARTESIAN_POINT('Ctrl Pts',(62.6814404185254,35.3280296500162,19.9294657090003));
#34258=CARTESIAN_POINT('Ctrl Pts',(62.563031207135,35.4573977295112,19.7757724373647));
#34259=CARTESIAN_POINT('Ctrl Pts',(62.4489672879057,35.5820183565476,19.6294657090004));
#34260=CARTESIAN_POINT('',(62.5717529460015,35.0245270751257,19.9294657090004));
#34261=CARTESIAN_POINT('Origin',(54.9397894030341,37.9543320991532,19.9294657090004));
#34262=CARTESIAN_POINT('',(62.2306155244487,34.9778443254007,19.6294657090004));
#34263=CARTESIAN_POINT('Ctrl Pts',(62.2306155244487,34.9778443254006,19.6294657090004));
#34264=CARTESIAN_POINT('Ctrl Pts',(62.3979960350237,35.0007494128826,19.7757724373647));
#34265=CARTESIAN_POINT('Ctrl Pts',(62.5717529460015,35.0245270751257,19.9294657090004));
#34266=CARTESIAN_POINT('',(62.4416126824056,34.705752027017,19.9294657090004));
#34267=CARTESIAN_POINT('Ctrl Pts',(62.4416126824056,34.705752027017,19.9294657090003));
#34268=CARTESIAN_POINT('Ctrl Pts',(62.3341421673715,34.8443410948853,19.7757724373647));
#34269=CARTESIAN_POINT('Ctrl Pts',(62.2306155244488,34.9778443254007,19.6294657090004));
#34270=CARTESIAN_POINT('',(62.3075519084639,34.4121998792067,19.9294657090004));
#34271=CARTESIAN_POINT('Origin',(54.9397894030341,37.9543320991532,19.9294657090004));
#34272=CARTESIAN_POINT('',(61.9637445160554,34.3934783293021,19.6294657090004));
#34273=CARTESIAN_POINT('Ctrl Pts',(61.9637445160554,34.3934783293021,19.6294657090004));
#34274=CARTESIAN_POINT('Ctrl Pts',(62.1324350590596,34.4026641364983,19.7757724373647));
#34275=CARTESIAN_POINT('Ctrl Pts',(62.3075519084639,34.4121998792067,19.9294657090004));
#34276=CARTESIAN_POINT('',(62.1518615500752,34.1050931684198,19.9294657090004));
#34277=CARTESIAN_POINT('Ctrl Pts',(62.1518615500752,34.1050931684198,19.9294657090003));
#34278=CARTESIAN_POINT('Ctrl Pts',(62.0560449299436,34.2519809372804,19.7757724373647));
#34279=CARTESIAN_POINT('Ctrl Pts',(61.9637445160554,34.3934783293021,19.6294657090004));
#34280=CARTESIAN_POINT('',(61.9943196270479,33.8234449888007,19.9294657090004));
#34281=CARTESIAN_POINT('Origin',(54.9397894030341,37.9543320991532,19.9294657090004));
#34282=CARTESIAN_POINT('',(61.6501302452559,33.8328092275425,19.6294657090004));
#34283=CARTESIAN_POINT('Ctrl Pts',(61.6501302452559,33.8328092275425,19.6294657090003));
#34284=CARTESIAN_POINT('Ctrl Pts',(61.8190082129576,33.8282146244215,19.7757724373647));
#34285=CARTESIAN_POINT('Ctrl Pts',(61.9943196270479,33.8234449888008,19.9294657090004));
#34286=CARTESIAN_POINT('',(61.8141152675145,33.5300503598269,19.9294657090004));
#34287=CARTESIAN_POINT('Ctrl Pts',(61.8141152675145,33.5300503598269,19.9294657090003));
#34288=CARTESIAN_POINT('Ctrl Pts',(61.7305901860837,33.6842593158128,19.7757724373647));
#34289=CARTESIAN_POINT('Ctrl Pts',(61.6501302452559,33.8328092275425,19.6294657090003));
#34290=CARTESIAN_POINT('',(61.6341406109067,33.2621804705658,19.9294657090004));
#34291=CARTESIAN_POINT('Origin',(54.9397894030341,37.9543320991532,19.9294657090004));
#34292=CARTESIAN_POINT('',(61.2918597632797,33.2995681804899,19.6294657090004));
#34293=CARTESIAN_POINT('Ctrl Pts',(61.2918597632797,33.2995681804899,19.6294657090003));
#34294=CARTESIAN_POINT('Ctrl Pts',(61.4598013006668,33.2812237433776,19.7757724373647));
#34295=CARTESIAN_POINT('Ctrl Pts',(61.6341406109066,33.2621804705658,19.9294657090003));
#34296=CARTESIAN_POINT('',(61.4306214805095,32.9844504162541,19.9294657090004));
#34297=CARTESIAN_POINT('Ctrl Pts',(61.4306214805096,32.9844504162541,19.9294657090003));
#34298=CARTESIAN_POINT('Ctrl Pts',(61.3599437834159,33.144954324206,19.7757724373647));
#34299=CARTESIAN_POINT('Ctrl Pts',(61.2918597632797,33.2995681804899,19.6294657090004));
#34300=CARTESIAN_POINT('',(61.2294117919672,32.7321414472685,19.9294657090004));
#34301=CARTESIAN_POINT('Origin',(54.9397894030341,37.9543320991532,19.9294657090004));
#34302=CARTESIAN_POINT('',(60.891317301074,32.7973038193341,19.6294657090004));
#34303=CARTESIAN_POINT('Ctrl Pts',(60.891317301074,32.7973038193341,19.6294657090003));
#34304=CARTESIAN_POINT('Ctrl Pts',(61.0572047849235,32.7653316274328,19.7757724373647));
#34305=CARTESIAN_POINT('Ctrl Pts',(61.2294117919672,32.7321414472685,19.9294657090003));
#34306=CARTESIAN_POINT('',(61.0039322769409,32.4719242153082,19.9294657090004));
#34307=CARTESIAN_POINT('Ctrl Pts',(61.0039322769409,32.4719242153082,19.9294657090003));
#34308=CARTESIAN_POINT('Ctrl Pts',(60.9465723125975,32.6376549481999,19.7757724373647));
#34309=CARTESIAN_POINT('Ctrl Pts',(60.891317301074,32.7973038193342,19.6294657090004));
#34310=CARTESIAN_POINT('',(60.7828265737441,32.2368552411588,19.9294657090004));
#34311=CARTESIAN_POINT('Origin',(54.9397894030341,37.9543320991532,19.9294657090004));
#34312=CARTESIAN_POINT('',(60.4511684026397,32.3293586305308,19.6294657090004));
#34313=CARTESIAN_POINT('Ctrl Pts',(60.4511684026397,32.3293586305308,19.6294657090003));
#34314=CARTESIAN_POINT('Ctrl Pts',(60.6138978791162,32.2839714535025,19.7757724373647));
#34315=CARTESIAN_POINT('Ctrl Pts',(60.7828265737441,32.2368552411588,19.9294657090003));
#34316=CARTESIAN_POINT('',(60.5368872030596,31.9958825342957,19.9294657090004));
#34317=CARTESIAN_POINT('Ctrl Pts',(60.5368872030596,31.9958825342957,19.9294657090003));
#34318=CARTESIAN_POINT('Ctrl Pts',(60.4932266925654,32.1657371814435,19.7757724373647));
#34319=CARTESIAN_POINT('Ctrl Pts',(60.4511684026397,32.3293586305308,19.6294657090003));
#34320=CARTESIAN_POINT('',(60.2973569071831,31.7796179002217,19.9294657090004));
#34321=CARTESIAN_POINT('Origin',(54.9397894030341,37.9543320991532,19.9294657090004));
#34322=CARTESIAN_POINT('',(59.9743421862767,31.8988467121058,19.6294657090004));
#34323=CARTESIAN_POINT('Ctrl Pts',(59.9743421862767,31.8988467121058,19.6294657090003));
#34324=CARTESIAN_POINT('Ctrl Pts',(60.1328307175625,31.8403465941253,19.7757724373647));
#34325=CARTESIAN_POINT('Ctrl Pts',(60.2973569071831,31.7796179002217,19.9294657090003));
#34326=CARTESIAN_POINT('',(60.0325943667752,31.5594933520624,19.9294657090004));
#34327=CARTESIAN_POINT('Ctrl Pts',(60.0325943667752,31.5594933520624,19.9294657090003));
#34328=CARTESIAN_POINT('Ctrl Pts',(60.0029238636241,31.7323415588135,19.7757724373647));
#34329=CARTESIAN_POINT('Ctrl Pts',(59.9743421862767,31.8988467121058,19.6294657090003));
#34330=CARTESIAN_POINT('',(59.7762335128185,31.3634722635224,19.9294657090004));
#34331=CARTESIAN_POINT('Origin',(54.9397894030341,37.9543320991532,19.9294657090004));
#34332=CARTESIAN_POINT('',(59.4640118517838,31.5086330498468,19.6294657090004));
#34333=CARTESIAN_POINT('Ctrl Pts',(59.4640118517838,31.5086330498468,19.6294657090004));
#34334=CARTESIAN_POINT('Ctrl Pts',(59.6172047228522,31.4374092995474,19.7757724373647));
#34335=CARTESIAN_POINT('Ctrl Pts',(59.7762335128185,31.3634722635223,19.9294657090003));
#34336=CARTESIAN_POINT('',(59.4944097537108,31.1656607666168,19.9294657090004));
#34337=CARTESIAN_POINT('Ctrl Pts',(59.4944097537108,31.1656607666168,19.9294657090003));
#34338=CARTESIAN_POINT('Ctrl Pts',(59.478926710206,31.3403522566732,19.7757724373647));
#34339=CARTESIAN_POINT('Ctrl Pts',(59.4640118517839,31.5086330498468,19.6294657090004));
#34340=CARTESIAN_POINT('',(59.2229243808604,30.9911877116138,19.9294657090004));
#34341=CARTESIAN_POINT('Origin',(54.9397894030341,37.9543320991532,19.9294657090004));
#34342=CARTESIAN_POINT('',(58.9235735633387,31.1613144512955,19.6294657090004));
#34343=CARTESIAN_POINT('Ctrl Pts',(58.9235735633388,31.1613144512955,19.6294657090004));
#34344=CARTESIAN_POINT('Ctrl Pts',(59.0704513009078,31.0778410509844,19.7757724373647));
#34345=CARTESIAN_POINT('Ctrl Pts',(59.2229243808603,30.9911877116138,19.9294657090003));
#34346=CARTESIAN_POINT('',(58.9259148936722,30.8170056688373,19.9294657090004));
#34347=CARTESIAN_POINT('Ctrl Pts',(58.9259148936721,30.8170056688373,19.9294657090003));
#34348=CARTESIAN_POINT('Ctrl Pts',(58.9247223469135,30.9923778991548,19.7757724373647));
#34349=CARTESIAN_POINT('Ctrl Pts',(58.9235735633387,31.1613144512955,19.6294657090003));
#34350=CARTESIAN_POINT('',(58.6411116922923,30.6652417367664,19.9294657090004));
#34351=CARTESIAN_POINT('Origin',(54.9397894030341,37.9543320991532,19.9294657090004));
#34352=CARTESIAN_POINT('',(58.356623848585,30.8592022644217,19.6294657090004));
#34353=CARTESIAN_POINT('Ctrl Pts',(58.356623848585,30.8592022644217,19.6294657090003));
#34354=CARTESIAN_POINT('Ctrl Pts',(58.4962090055442,30.7640347158058,19.7757724373647));
#34355=CARTESIAN_POINT('Ctrl Pts',(58.6411116922923,30.6652417367664,19.9294657090003));
#34356=CARTESIAN_POINT('',(58.3308930261577,30.5158483008756,19.9294657090004));
#34357=CARTESIAN_POINT('Ctrl Pts',(58.3308930261577,30.5158483008756,19.9294657090003));
#34358=CARTESIAN_POINT('Ctrl Pts',(58.3439989123473,30.6907341981958,19.7757724373647));
#34359=CARTESIAN_POINT('Ctrl Pts',(58.356623848585,30.8592022644217,19.6294657090003));
#34360=CARTESIAN_POINT('',(58.0346673145644,30.3878034556654,19.9294657090004));
#34361=CARTESIAN_POINT('Origin',(54.9397894030341,37.9543320991532,19.9294657090004));
#34362=CARTESIAN_POINT('',(57.766935664334,30.604306995984,19.6294657090004));
#34363=CARTESIAN_POINT('Ctrl Pts',(57.766935664334,30.604306995984,19.6294657090004));
#34364=CARTESIAN_POINT('Ctrl Pts',(57.8982993244938,30.4980786233978,19.7757724373647));
#34365=CARTESIAN_POINT('Ctrl Pts',(58.0346673145644,30.3878034556654,19.9294657090003));
#34366=CARTESIAN_POINT('',(57.7133039235241,30.264192815328,19.9294657090004));
#34367=CARTESIAN_POINT('Ctrl Pts',(57.7133039235241,30.264192815328,19.9294657090004));
#34368=CARTESIAN_POINT('Ctrl Pts',(57.7406210251516,30.4374285428584,19.7757724373647));
#34369=CARTESIAN_POINT('Ctrl Pts',(57.7669356643341,30.604306995984,19.6294657090004));
#34370=CARTESIAN_POINT('',(57.4076270349543,30.1607191742974,19.9294657090004));
#34371=CARTESIAN_POINT('Origin',(54.9397894030341,37.9543320991532,19.9294657090004));
#34372=CARTESIAN_POINT('',(57.1584332881605,30.3983249319391,19.6294657090004));
#34373=CARTESIAN_POINT('Ctrl Pts',(57.1584332881605,30.3983249319391,19.6294657090003));
#34374=CARTESIAN_POINT('Ctrl Pts',(57.2807012480359,30.2817426676757,19.7757724373647));
#34375=CARTESIAN_POINT('Ctrl Pts',(57.4076270349543,30.1607191742974,19.9294657090003));
#34376=CARTESIAN_POINT('',(57.0772575393543,30.0637139379306,19.9294657090004));
#34377=CARTESIAN_POINT('Ctrl Pts',(57.0772575393543,30.0637139379306,19.9294657090004));
#34378=CARTESIAN_POINT('Ctrl Pts',(57.1186040656154,30.2341466404863,19.7757724373647));
#34379=CARTESIAN_POINT('Ctrl Pts',(57.1584332881605,30.3983249319391,19.6294657090003));
#34380=CARTESIAN_POINT('',(56.7641637030682,29.9855001010888,19.9294657090004));
#34381=CARTESIAN_POINT('Origin',(54.9397894030341,37.9543320991532,19.9294657090004));
#34382=CARTESIAN_POINT('',(56.5351662029818,30.2426268489385,19.6294657090004));
#34383=CARTESIAN_POINT('Ctrl Pts',(56.5351662029818,30.2426268489385,19.6294657090003));
#34384=CARTESIAN_POINT('Ctrl Pts',(56.6475247894728,30.1164665287319,19.7757724373647));
#34385=CARTESIAN_POINT('Ctrl Pts',(56.7641637030682,29.9855001010888,19.9294657090003));
#34386=CARTESIAN_POINT('',(56.4269866573947,29.9157458225358,19.9294657090004));
#34387=CARTESIAN_POINT('Ctrl Pts',(56.4269866573947,29.9157458225358,19.9294657090003));
#34388=CARTESIAN_POINT('Ctrl Pts',(56.4820874539788,30.0822412986007,19.7757724373647));
#34389=CARTESIAN_POINT('Ctrl Pts',(56.5351662029818,30.2426268489385,19.6294657090004));
#34390=CARTESIAN_POINT('',(56.108559461216,29.8633122900625,19.9294657090004));
#34391=CARTESIAN_POINT('Origin',(54.9397894030341,37.9543320991532,19.9294657090004));
#34392=CARTESIAN_POINT('',(55.9012821484182,30.1382488920364,19.6294657090004));
#34393=CARTESIAN_POINT('Ctrl Pts',(55.9012821484182,30.1382488920364,19.6294657090004));
#34394=CARTESIAN_POINT('Ctrl Pts',(56.0029836336694,30.0033500920025,19.7757724373647));
#34395=CARTESIAN_POINT('Ctrl Pts',(56.108559461216,29.8633122900626,19.9294657090003));
#34396=CARTESIAN_POINT('',(55.7668187230776,29.8212731725384,19.9294657090004));
#34397=CARTESIAN_POINT('Ctrl Pts',(55.7668187230776,29.8212731725384,19.9294657090004));
#34398=CARTESIAN_POINT('Ctrl Pts',(55.8353071032744,29.9827234221893,19.7757724373647));
#34399=CARTESIAN_POINT('Ctrl Pts',(55.9012821484182,30.1382488920364,19.6294657090004));
#34400=CARTESIAN_POINT('',(55.44517724746,29.7949688809415,19.9294657090004));
#34401=CARTESIAN_POINT('Origin',(54.9397894030341,37.9543320991532,19.9294657090004));
#34402=CARTESIAN_POINT('',(55.2609995182692,30.0858856793146,19.6294657090004));
#34403=CARTESIAN_POINT('Ctrl Pts',(55.2609995182692,30.0858856793146,19.6294657090003));
#34404=CARTESIAN_POINT('Ctrl Pts',(55.3513670956759,29.943146128711,19.7757724373647));
#34405=CARTESIAN_POINT('Ctrl Pts',(55.44517724746,29.7949688809415,19.9294657090003));
#34406=CARTESIAN_POINT('',(55.1011470450858,29.7809246878375,19.9294657090004));
#34407=CARTESIAN_POINT('Ctrl Pts',(55.1011470450858,29.7809246878375,19.9294657090004));
#34408=CARTESIAN_POINT('Ctrl Pts',(55.182567230025,29.9362552863001,19.7757724373647));
#34409=CARTESIAN_POINT('Ctrl Pts',(55.2609995182692,30.0858856793146,19.6294657090004));
#34410=CARTESIAN_POINT('',(54.7784317609826,29.7809246878375,19.9294657090004));
#34411=CARTESIAN_POINT('Origin',(54.9397894030341,37.9543320991532,19.9294657090004));
#34412=CARTESIAN_POINT('',(54.6185792877992,30.0858856793146,19.6294657090004));
#34413=CARTESIAN_POINT('Ctrl Pts',(54.6185792877992,30.0858856793146,19.6294657090003));
#34414=CARTESIAN_POINT('Ctrl Pts',(54.6970115760434,29.9362552863001,19.7757724373647));
#34415=CARTESIAN_POINT('Ctrl Pts',(54.7784317609826,29.7809246878375,19.9294657090003));
#34416=CARTESIAN_POINT('',(54.4344015586084,29.7949688809415,19.9294657090004));
#34417=CARTESIAN_POINT('Ctrl Pts',(54.4344015586084,29.7949688809415,19.9294657090003));
#34418=CARTESIAN_POINT('Ctrl Pts',(54.5282117103925,29.943146128711,19.7757724373647));
#34419=CARTESIAN_POINT('Ctrl Pts',(54.6185792877992,30.0858856793146,19.6294657090003));
#34420=CARTESIAN_POINT('',(54.1127600829908,29.8212731725384,19.9294657090004));
#34421=CARTESIAN_POINT('Origin',(54.9397894030341,37.9543320991532,19.9294657090004));
#34422=CARTESIAN_POINT('',(53.9782966576502,30.1382488920364,19.6294657090004));
#34423=CARTESIAN_POINT('Ctrl Pts',(53.9782966576502,30.1382488920364,19.6294657090003));
#34424=CARTESIAN_POINT('Ctrl Pts',(54.0442717027939,29.9827234221892,19.7757724373647));
#34425=CARTESIAN_POINT('Ctrl Pts',(54.1127600829908,29.8212731725384,19.9294657090003));
#34426=CARTESIAN_POINT('',(53.7710193448524,29.8633122900625,19.9294657090004));
#34427=CARTESIAN_POINT('Ctrl Pts',(53.7710193448524,29.8633122900625,19.9294657090003));
#34428=CARTESIAN_POINT('Ctrl Pts',(53.8765951723989,30.0033500920025,19.7757724373647));
#34429=CARTESIAN_POINT('Ctrl Pts',(53.9782966576502,30.1382488920364,19.6294657090003));
#34430=CARTESIAN_POINT('',(53.4525921486737,29.9157458225357,19.9294657090004));
#34431=CARTESIAN_POINT('Origin',(54.9397894030341,37.9543320991532,19.9294657090004));
#34432=CARTESIAN_POINT('',(53.3444126030865,30.2426268489385,19.6294657090004));
#34433=CARTESIAN_POINT('Ctrl Pts',(53.3444126030866,30.2426268489385,19.6294657090003));
#34434=CARTESIAN_POINT('Ctrl Pts',(53.3974913520896,30.0822412986007,19.7757724373647));
#34435=CARTESIAN_POINT('Ctrl Pts',(53.4525921486737,29.9157458225357,19.9294657090003));
#34436=CARTESIAN_POINT('',(53.1154151030002,29.9855001010888,19.9294657090004));
#34437=CARTESIAN_POINT('Ctrl Pts',(53.1154151030002,29.9855001010888,19.9294657090003));
#34438=CARTESIAN_POINT('Ctrl Pts',(53.2320540165956,30.1164665287319,19.7757724373647));
#34439=CARTESIAN_POINT('Ctrl Pts',(53.3444126030865,30.2426268489385,19.6294657090003));
#34440=CARTESIAN_POINT('',(52.8023212667141,30.0637139379306,19.9294657090004));
#34441=CARTESIAN_POINT('Origin',(54.9397894030341,37.9543320991532,19.9294657090004));
#34442=CARTESIAN_POINT('',(52.7211455179079,30.398324931939,19.6294657090004));
#34443=CARTESIAN_POINT('Ctrl Pts',(52.7211455179079,30.398324931939,19.6294657090004));
#34444=CARTESIAN_POINT('Ctrl Pts',(52.760974740453,30.2341466404863,19.7757724373647));
#34445=CARTESIAN_POINT('Ctrl Pts',(52.8023212667141,30.0637139379306,19.9294657090004));
#34446=CARTESIAN_POINT('',(52.4719517711141,30.1607191742974,19.9294657090004));
#34447=CARTESIAN_POINT('Ctrl Pts',(52.4719517711141,30.1607191742974,19.9294657090003));
#34448=CARTESIAN_POINT('Ctrl Pts',(52.5988775580325,30.2817426676756,19.7757724373647));
#34449=CARTESIAN_POINT('Ctrl Pts',(52.7211455179079,30.398324931939,19.6294657090004));
#34450=CARTESIAN_POINT('',(52.1662748825443,30.264192815328,19.9294657090004));
#34451=CARTESIAN_POINT('Origin',(54.9397894030341,37.9543320991532,19.9294657090004));
#34452=CARTESIAN_POINT('',(52.1126431417343,30.6043069959839,19.6294657090004));
#34453=CARTESIAN_POINT('Ctrl Pts',(52.1126431417343,30.6043069959839,19.6294657090004));
#34454=CARTESIAN_POINT('Ctrl Pts',(52.1389577809168,30.4374285428584,19.7757724373647));
#34455=CARTESIAN_POINT('Ctrl Pts',(52.1662748825443,30.264192815328,19.9294657090004));
#34456=CARTESIAN_POINT('',(51.8449114915039,30.3878034556653,19.9294657090004));
#34457=CARTESIAN_POINT('Ctrl Pts',(51.8449114915039,30.3878034556653,19.9294657090003));
#34458=CARTESIAN_POINT('Ctrl Pts',(51.9812794815746,30.4980786233977,19.7757724373647));
#34459=CARTESIAN_POINT('Ctrl Pts',(52.1126431417343,30.6043069959839,19.6294657090003));
#34460=CARTESIAN_POINT('',(51.5486857799107,30.5158483008756,19.9294657090004));
#34461=CARTESIAN_POINT('Origin',(54.9397894030341,37.9543320991532,19.9294657090004));
#34462=CARTESIAN_POINT('',(51.5229549574834,30.8592022644217,19.6294657090004));
#34463=CARTESIAN_POINT('Ctrl Pts',(51.5229549574834,30.8592022644216,19.6294657090004));
#34464=CARTESIAN_POINT('Ctrl Pts',(51.5355798937211,30.6907341981958,19.7757724373647));
#34465=CARTESIAN_POINT('Ctrl Pts',(51.5486857799107,30.5158483008756,19.9294657090004));
#34466=CARTESIAN_POINT('',(51.2384671137761,30.6652417367663,19.9294657090004));
#34467=CARTESIAN_POINT('Ctrl Pts',(51.2384671137761,30.6652417367663,19.9294657090003));
#34468=CARTESIAN_POINT('Ctrl Pts',(51.3833698005242,30.7640347158057,19.7757724373647));
#34469=CARTESIAN_POINT('Ctrl Pts',(51.5229549574834,30.8592022644217,19.6294657090004));
#34470=CARTESIAN_POINT('',(50.9536639123962,30.8170056688373,19.9294657090004));
#34471=CARTESIAN_POINT('Origin',(54.9397894030341,37.9543320991532,19.9294657090004));
#34472=CARTESIAN_POINT('',(50.9560052427296,31.1613144512955,19.6294657090004));
#34473=CARTESIAN_POINT('Ctrl Pts',(50.9560052427296,31.1613144512955,19.6294657090004));
#34474=CARTESIAN_POINT('Ctrl Pts',(50.9548564591548,30.9923778991548,19.7757724373647));
#34475=CARTESIAN_POINT('Ctrl Pts',(50.9536639123962,30.8170056688373,19.9294657090004));
#34476=CARTESIAN_POINT('',(50.656654425208,30.9911877116138,19.9294657090004));
#34477=CARTESIAN_POINT('Ctrl Pts',(50.656654425208,30.9911877116138,19.9294657090003));
#34478=CARTESIAN_POINT('Ctrl Pts',(50.8091275051606,31.0778410509844,19.7757724373647));
#34479=CARTESIAN_POINT('Ctrl Pts',(50.9560052427296,31.1613144512955,19.6294657090003));
#34480=CARTESIAN_POINT('',(50.3851690523575,31.1656607666167,19.9294657090004));
#34481=CARTESIAN_POINT('Origin',(54.9397894030341,37.9543320991532,19.9294657090004));
#34482=CARTESIAN_POINT('',(50.4155669542845,31.5086330498468,19.6294657090004));
#34483=CARTESIAN_POINT('Ctrl Pts',(50.4155669542845,31.5086330498468,19.6294657090003));
#34484=CARTESIAN_POINT('Ctrl Pts',(50.4006520958624,31.3403522566732,19.7757724373647));
#34485=CARTESIAN_POINT('Ctrl Pts',(50.3851690523575,31.1656607666167,19.9294657090003));
#34486=CARTESIAN_POINT('',(50.1033452932499,31.3634722635223,19.9294657090004));
#34487=CARTESIAN_POINT('Ctrl Pts',(50.1033452932499,31.3634722635223,19.9294657090003));
#34488=CARTESIAN_POINT('Ctrl Pts',(50.2623740832161,31.4374092995474,19.7757724373647));
#34489=CARTESIAN_POINT('Ctrl Pts',(50.4155669542845,31.5086330498468,19.6294657090003));
#34490=CARTESIAN_POINT('',(49.8469844392931,31.5594933520623,19.9294657090004));
#34491=CARTESIAN_POINT('Origin',(54.9397894030341,37.9543320991532,19.9294657090004));
#34492=CARTESIAN_POINT('',(49.9052366197917,31.8988467121057,19.6294657090004));
#34493=CARTESIAN_POINT('Ctrl Pts',(49.9052366197917,31.8988467121057,19.6294657090003));
#34494=CARTESIAN_POINT('Ctrl Pts',(49.8766549424443,31.7323415588134,19.7757724373647));
#34495=CARTESIAN_POINT('Ctrl Pts',(49.8469844392931,31.5594933520623,19.9294657090003));
#34496=CARTESIAN_POINT('',(49.5822218988852,31.7796179002216,19.9294657090004));
#34497=CARTESIAN_POINT('Ctrl Pts',(49.5822218988852,31.7796179002216,19.9294657090004));
#34498=CARTESIAN_POINT('Ctrl Pts',(49.7467480885058,31.8403465941252,19.7757724373647));
#34499=CARTESIAN_POINT('Ctrl Pts',(49.9052366197917,31.8988467121057,19.6294657090004));
#34500=CARTESIAN_POINT('',(49.3426916030088,31.9958825342957,19.9294657090004));
#34501=CARTESIAN_POINT('Origin',(54.9397894030341,37.9543320991532,19.9294657090004));
#34502=CARTESIAN_POINT('',(49.4284104034286,32.3293586305307,19.6294657090004));
#34503=CARTESIAN_POINT('Ctrl Pts',(49.4284104034286,32.3293586305307,19.6294657090003));
#34504=CARTESIAN_POINT('Ctrl Pts',(49.386352113503,32.1657371814434,19.7757724373647));
#34505=CARTESIAN_POINT('Ctrl Pts',(49.3426916030088,31.9958825342957,19.9294657090003));
#34506=CARTESIAN_POINT('',(49.0967522323243,32.2368552411587,19.9294657090004));
#34507=CARTESIAN_POINT('Ctrl Pts',(49.0967522323243,32.2368552411587,19.9294657090004));
#34508=CARTESIAN_POINT('Ctrl Pts',(49.2656809269522,32.2839714535024,19.7757724373647));
#34509=CARTESIAN_POINT('Ctrl Pts',(49.4284104034286,32.3293586305307,19.6294657090003));
#34510=CARTESIAN_POINT('',(48.8756465291274,32.4719242153081,19.9294657090004));
#34511=CARTESIAN_POINT('Origin',(54.9397894030341,37.9543320991532,19.9294657090004));
#34512=CARTESIAN_POINT('',(48.9882615049944,32.7973038193341,19.6294657090004));
#34513=CARTESIAN_POINT('Ctrl Pts',(48.9882615049944,32.7973038193341,19.6294657090003));
#34514=CARTESIAN_POINT('Ctrl Pts',(48.9330064934709,32.6376549481999,19.7757724373647));
#34515=CARTESIAN_POINT('Ctrl Pts',(48.8756465291274,32.4719242153081,19.9294657090004));
#34516=CARTESIAN_POINT('',(48.6501670141011,32.7321414472684,19.9294657090004));
#34517=CARTESIAN_POINT('Ctrl Pts',(48.6501670141011,32.7321414472685,19.9294657090004));
#34518=CARTESIAN_POINT('Ctrl Pts',(48.8223740211449,32.7653316274327,19.7757724373647));
#34519=CARTESIAN_POINT('Ctrl Pts',(48.9882615049944,32.7973038193341,19.6294657090003));
#34520=CARTESIAN_POINT('',(48.4489573255588,32.984450416254,19.9294657090004));
#34521=CARTESIAN_POINT('Origin',(54.9397894030341,37.9543320991532,19.9294657090004));
#34522=CARTESIAN_POINT('',(48.5877190427886,33.2995681804899,19.6294657090004));
#34523=CARTESIAN_POINT('Ctrl Pts',(48.5877190427886,33.2995681804898,19.6294657090004));
#34524=CARTESIAN_POINT('Ctrl Pts',(48.5196350226525,33.1449543242059,19.7757724373647));
#34525=CARTESIAN_POINT('Ctrl Pts',(48.4489573255588,32.984450416254,19.9294657090004));
#34526=CARTESIAN_POINT('',(48.2454381951617,33.2621804705657,19.9294657090004));
#34527=CARTESIAN_POINT('Ctrl Pts',(48.2454381951617,33.2621804705657,19.9294657090003));
#34528=CARTESIAN_POINT('Ctrl Pts',(48.4197775054016,33.2812237433775,19.7757724373647));
#34529=CARTESIAN_POINT('Ctrl Pts',(48.5877190427886,33.2995681804899,19.6294657090004));
#34530=CARTESIAN_POINT('',(48.0654635385539,33.5300503598268,19.9294657090004));
#34531=CARTESIAN_POINT('Origin',(54.9397894030341,37.9543320991532,19.9294657090004));
#34532=CARTESIAN_POINT('',(48.2294485608124,33.8328092275424,19.6294657090004));
#34533=CARTESIAN_POINT('Ctrl Pts',(48.2294485608124,33.8328092275424,19.6294657090004));
#34534=CARTESIAN_POINT('Ctrl Pts',(48.1489886199846,33.6842593158128,19.7757724373647));
#34535=CARTESIAN_POINT('Ctrl Pts',(48.0654635385539,33.5300503598268,19.9294657090004));
#34536=CARTESIAN_POINT('',(47.8852591790204,33.8234449888006,19.9294657090004));
#34537=CARTESIAN_POINT('Ctrl Pts',(47.8852591790204,33.8234449888007,19.9294657090004));
#34538=CARTESIAN_POINT('Ctrl Pts',(48.0605705931107,33.8282146244214,19.7757724373647));
#34539=CARTESIAN_POINT('Ctrl Pts',(48.2294485608124,33.8328092275424,19.6294657090004));
#34540=CARTESIAN_POINT('',(47.7277172559931,34.1050931684197,19.9294657090004));
#34541=CARTESIAN_POINT('Origin',(54.9397894030341,37.9543320991532,19.9294657090004));
#34542=CARTESIAN_POINT('',(47.9158342900129,34.393478329302,19.6294657090004));
#34543=CARTESIAN_POINT('Ctrl Pts',(47.9158342900129,34.393478329302,19.6294657090003));
#34544=CARTESIAN_POINT('Ctrl Pts',(47.8235338761247,34.2519809372803,19.7757724373647));
#34545=CARTESIAN_POINT('Ctrl Pts',(47.7277172559931,34.1050931684197,19.9294657090003));
#34546=CARTESIAN_POINT('',(47.5720268976044,34.4121998792066,19.9294657090004));
#34547=CARTESIAN_POINT('Ctrl Pts',(47.5720268976044,34.4121998792066,19.9294657090004));
#34548=CARTESIAN_POINT('Ctrl Pts',(47.7471437470088,34.4026641364982,19.7757724373647));
#34549=CARTESIAN_POINT('Ctrl Pts',(47.9158342900129,34.393478329302,19.6294657090004));
#34550=CARTESIAN_POINT('',(47.4379661236627,34.7057520270169,19.9294657090004));
#34551=CARTESIAN_POINT('Origin',(54.9397894030341,37.9543320991532,19.9294657090004));
#34552=CARTESIAN_POINT('',(47.6489632816196,34.9778443254006,19.6294657090004));
#34553=CARTESIAN_POINT('Ctrl Pts',(47.6489632816196,34.9778443254005,19.6294657090003));
#34554=CARTESIAN_POINT('Ctrl Pts',(47.5454366386968,34.8443410948852,19.7757724373647));
#34555=CARTESIAN_POINT('Ctrl Pts',(47.4379661236628,34.7057520270169,19.9294657090003));
#34556=CARTESIAN_POINT('',(47.3078258600668,35.0245270751256,19.9294657090004));
#34557=CARTESIAN_POINT('Ctrl Pts',(47.3078258600668,35.0245270751256,19.9294657090003));
#34558=CARTESIAN_POINT('Ctrl Pts',(47.4815827710446,35.0007494128825,19.7757724373647));
#34559=CARTESIAN_POINT('Ctrl Pts',(47.6489632816196,34.9778443254006,19.6294657090004));
#34560=CARTESIAN_POINT('',(47.1981383875429,35.3280296500161,19.9294657090004));
#34561=CARTESIAN_POINT('Origin',(54.9397894030341,37.9543320991532,19.9294657090004));
#34562=CARTESIAN_POINT('',(47.4306115181626,35.5820183565475,19.6294657090004));
#34563=CARTESIAN_POINT('Ctrl Pts',(47.4306115181626,35.5820183565475,19.6294657090004));
#34564=CARTESIAN_POINT('Ctrl Pts',(47.3165475989333,35.4573977295111,19.7757724373647));
#34565=CARTESIAN_POINT('Ctrl Pts',(47.1981383875429,35.3280296500162,19.9294657090004));
#34566=CARTESIAN_POINT('',(47.0944142807223,35.6563516400958,19.9294657090004));
#34567=CARTESIAN_POINT('Ctrl Pts',(47.0944142807223,35.6563516400958,19.9294657090004));
#34568=CARTESIAN_POINT('Ctrl Pts',(47.2656549296989,35.6184902947371,19.7757724373647));
#34569=CARTESIAN_POINT('Ctrl Pts',(47.4306115181626,35.5820183565475,19.6294657090004));
#34570=CARTESIAN_POINT('',(47.0098300616486,35.967784882505,19.9294657090004));
#34571=CARTESIAN_POINT('Origin',(54.9397894030341,37.9543320991532,19.9294657090004));
#34572=CARTESIAN_POINT('',(47.2622320946023,36.2019797442472,19.6294657090004));
#34573=CARTESIAN_POINT('Ctrl Pts',(47.2622320946023,36.2019797442472,19.6294657090003));
#34574=CARTESIAN_POINT('Ctrl Pts',(47.1383899756297,36.0870710504017,19.7757724373647));
#34575=CARTESIAN_POINT('Ctrl Pts',(47.0098300616486,35.967784882505,19.9294657090003));
#34576=CARTESIAN_POINT('',(46.9332123784209,36.3034688858808,19.9294657090004));
#34577=CARTESIAN_POINT('Ctrl Pts',(46.9332123784209,36.3034688858808,19.9294657090004));
#34578=CARTESIAN_POINT('Ctrl Pts',(47.1007971871301,36.2517758184133,19.7757724373647));
#34579=CARTESIAN_POINT('Ctrl Pts',(47.2622320946023,36.2019797442472,19.6294657090004));
#34580=CARTESIAN_POINT('',(46.8742943068201,36.6207602589635,19.9294657090004));
#34581=CARTESIAN_POINT('Origin',(54.9397894030341,37.9543320991532,19.9294657090004));
#34582=CARTESIAN_POINT('',(47.1449455482218,36.8336027477511,19.6294657090004));
#34583=CARTESIAN_POINT('Ctrl Pts',(47.1449455482218,36.8336027477511,19.6294657090003));
#34584=CARTESIAN_POINT('Ctrl Pts',(47.0121493783752,36.7291706854955,19.7757724373647));
#34585=CARTESIAN_POINT('Ctrl Pts',(46.8742943068201,36.6207602589635,19.9294657090003));
#34586=CARTESIAN_POINT('',(46.8252929252262,36.961572353977,19.9294657090004));
#34587=CARTESIAN_POINT('Ctrl Pts',(46.8252929252262,36.961572353977,19.9294657090004));
#34588=CARTESIAN_POINT('Ctrl Pts',(46.9881066444156,36.8963915732357,19.7757724373647));
#34589=CARTESIAN_POINT('Ctrl Pts',(47.1449455482218,36.8336027477511,19.6294657090003));
#34590=CARTESIAN_POINT('',(46.7924330911438,37.2826103359946,19.9294657090004));
#34591=CARTESIAN_POINT('Origin',(54.9397894030341,37.9543320991532,19.9294657090004));
#34592=CARTESIAN_POINT('',(47.0795324016364,37.4726840201812,19.6294657090004));
#34593=CARTESIAN_POINT('Ctrl Pts',(47.0795324016364,37.4726840201812,19.6294657090004));
#34594=CARTESIAN_POINT('Ctrl Pts',(46.9386659175162,37.3794235676597,19.7757724373647));
#34595=CARTESIAN_POINT('Ctrl Pts',(46.7924330911438,37.2826103359945,19.9294657090004));
#34596=CARTESIAN_POINT('',(46.7713741072936,37.6262824743834,19.9294657090004));
#34597=CARTESIAN_POINT('Ctrl Pts',(46.7713741072936,37.6262824743834,19.9294657090004));
#34598=CARTESIAN_POINT('Ctrl Pts',(46.9283332385243,37.5480477477103,19.7757724373647));
#34599=CARTESIAN_POINT('Ctrl Pts',(47.0795324016364,37.4726840201812,19.6294657090004));
#34600=CARTESIAN_POINT('',(46.764791187504,37.9489306105331,19.9294657090004));
#34601=CARTESIAN_POINT('Origin',(54.9397894030341,37.9543320991532,19.9294657090004));
#34602=CARTESIAN_POINT('',(46.7746038105401,37.9543320991532,19.9196513014945));
#34603=CARTESIAN_POINT('Ctrl Pts',(46.764791187504,37.9489306105331,19.9294657090004));
#34604=CARTESIAN_POINT('Ctrl Pts',(46.7697004459005,37.9516329769915,19.924554666134));
#34605=CARTESIAN_POINT('Ctrl Pts',(46.7746038105401,37.9543320991532,19.9196513014945));
#34606=CARTESIAN_POINT('',(47.1647894030341,37.9543320991532,19.5294657090004));
#34607=CARTESIAN_POINT('',(46.7647894030341,37.9543320991532,19.9294657090004));
#34608=CARTESIAN_POINT('Origin',(54.9397894030341,37.9543320991532,19.5294657090004));
#34609=CARTESIAN_POINT('',(47.0664279685441,38.1149705811105,19.6294657090004));
#34610=CARTESIAN_POINT('Ctrl Pts',(46.7746038105401,37.9543320991532,19.9196513014945));
#34611=CARTESIAN_POINT('Ctrl Pts',(46.9231556085686,38.0361044085143,19.7710995034659));
#34612=CARTESIAN_POINT('Ctrl Pts',(47.0664279685441,38.1149705811105,19.6294657090004));
#34613=CARTESIAN_POINT('',(46.7718147454605,38.2931757109183,19.9294657090004));
#34614=CARTESIAN_POINT('Ctrl Pts',(46.7718147454605,38.2931757109183,19.9294657090004));
#34615=CARTESIAN_POINT('Ctrl Pts',(46.9218747516106,38.2024076775116,19.7757724373647));
#34616=CARTESIAN_POINT('Ctrl Pts',(47.0664279685441,38.1149705811105,19.6294657090004));
#34617=CARTESIAN_POINT('',(46.7915525482088,38.6152868310873,19.9294657090004));
#34618=CARTESIAN_POINT('Origin',(54.9397894030341,37.9543320991532,19.9294657090004));
#34619=CARTESIAN_POINT('',(47.1057194567852,38.7561881194459,19.6294657090004));
#34620=CARTESIAN_POINT('Ctrl Pts',(47.1057194567852,38.7561881194459,19.6294657090004));
#34621=CARTESIAN_POINT('Ctrl Pts',(46.9515721418295,38.6870543097372,19.7757724373647));
#34622=CARTESIAN_POINT('Ctrl Pts',(46.7915525482088,38.6152868310873,19.9294657090003));
#34623=CARTESIAN_POINT('',(46.8266119073525,38.9578139991222,19.9294657090004));
#34624=CARTESIAN_POINT('Ctrl Pts',(46.8266119073525,38.9578139991222,19.9294657090004));
#34625=CARTESIAN_POINT('Ctrl Pts',(46.9687741638393,38.8551167052684,19.7757724373647));
#34626=CARTESIAN_POINT('Ctrl Pts',(47.1057194567852,38.7561881194459,19.6294657090003));
#34627=CARTESIAN_POINT('',(46.872539080818,39.2772445069503,19.9294657090004));
#34628=CARTESIAN_POINT('Origin',(54.9397894030341,37.9543320991532,19.9294657090004));
#34629=CARTESIAN_POINT('',(47.197145387988,39.3920694382632,19.6294657090004));
#34630=CARTESIAN_POINT('Ctrl Pts',(47.1971453879881,39.3920694382632,19.6294657090004));
#34631=CARTESIAN_POINT('Ctrl Pts',(47.0378759382084,39.3357301028059,19.7757724373647));
#34632=CARTESIAN_POINT('Ctrl Pts',(46.872539080818,39.2772445069503,19.9294657090004));
#34633=CARTESIAN_POINT('',(46.9354009268983,39.6157742808447,19.9294657090004));
#34634=CARTESIAN_POINT('Ctrl Pts',(46.9354009268983,39.6157742808447,19.9294657090004));
#34635=CARTESIAN_POINT('Ctrl Pts',(47.0687193673599,39.5018311600905,19.7757724373647));
#34636=CARTESIAN_POINT('Ctrl Pts',(47.197145387988,39.3920694382632,19.6294657090004));
#34637=CARTESIAN_POINT('',(47.0072118333189,39.9303984190046,19.9294657090004));
#34638=CARTESIAN_POINT('Origin',(54.9397894030341,37.9543320991532,19.9294657090004));
#34639=CARTESIAN_POINT('',(47.3400973376647,40.0183828522986,19.6294657090004));
#34640=CARTESIAN_POINT('Ctrl Pts',(47.3400973376646,40.0183828522986,19.6294657090004));
#34641=CARTESIAN_POINT('Ctrl Pts',(47.1767656649717,39.9752129200749,19.7757724373647));
#34642=CARTESIAN_POINT('Ctrl Pts',(47.0072118333189,39.9303984190046,19.9294657090004));
#34643=CARTESIAN_POINT('',(47.0974578311216,40.2626779389666,19.9294657090004));
#34644=CARTESIAN_POINT('Ctrl Pts',(47.0974578311216,40.2626779389666,19.9294657090004));
#34645=CARTESIAN_POINT('Ctrl Pts',(47.2210452433328,40.1382472639815,19.7757724373647));
#34646=CARTESIAN_POINT('Ctrl Pts',(47.3400973376647,40.0183828522986,19.6294657090004));
#34647=CARTESIAN_POINT('',(47.1946745807631,40.5704019357283,19.9294657090004));
#34648=CARTESIAN_POINT('Origin',(54.9397894030341,37.9543320991532,19.9294657090004));
#34649=CARTESIAN_POINT('',(47.5336239841754,40.6309603491163,19.6294657090004));
#34650=CARTESIAN_POINT('Ctrl Pts',(47.5336239841753,40.6309603491163,19.6294657090004));
#34651=CARTESIAN_POINT('Ctrl Pts',(47.367317033903,40.6012471089026,19.7757724373647));
#34652=CARTESIAN_POINT('Ctrl Pts',(47.1946745807631,40.5704019357283,19.9294657090003));
#34653=CARTESIAN_POINT('',(47.3117041580624,40.8942199363749,19.9294657090004));
#34654=CARTESIAN_POINT('Ctrl Pts',(47.3117041580624,40.8942199363749,19.9294657090004));
#34655=CARTESIAN_POINT('Ctrl Pts',(47.4247380881853,40.7601297727712,19.7757724373647));
#34656=CARTESIAN_POINT('Ctrl Pts',(47.5336239841754,40.6309603491163,19.6294657090004));
#34657=CARTESIAN_POINT('',(47.4336797894956,41.1929959393107,19.9294657090004));
#34658=CARTESIAN_POINT('Origin',(54.9397894030341,37.9543320991532,19.9294657090004));
#34659=CARTESIAN_POINT('',(47.7764374396173,41.2257253265431,19.6294657090004));
#34660=CARTESIAN_POINT('Ctrl Pts',(47.7764374396173,41.2257253265431,19.6294657090004));
#34661=CARTESIAN_POINT('Ctrl Pts',(47.6082619570809,41.2096665150506,19.7757724373647));
#34662=CARTESIAN_POINT('Ctrl Pts',(47.4336797894956,41.1929959393107,19.9294657090003));
#34663=CARTESIAN_POINT('',(47.5767141337629,41.5061974652738,19.9294657090004));
#34664=CARTESIAN_POINT('Ctrl Pts',(47.5767141337629,41.5061974652738,19.9294657090004));
#34665=CARTESIAN_POINT('Ctrl Pts',(47.678442359642,41.363340160967,19.7757724373647));
#34666=CARTESIAN_POINT('Ctrl Pts',(47.7764374396173,41.2257253265431,19.6294657090004));
#34667=CARTESIAN_POINT('',(47.7226369192852,41.7940371693788,19.9294657090004));
#34668=CARTESIAN_POINT('Origin',(54.9397894030341,37.9543320991532,19.9294657090004));
#34669=CARTESIAN_POINT('',(48.0669218205059,41.7987197217834,19.6294657090004));
#34670=CARTESIAN_POINT('Ctrl Pts',(48.0669218205059,41.7987197217834,19.6294657090004));
#34671=CARTESIAN_POINT('Ctrl Pts',(47.8979969857948,41.7964222077531,19.7757724373647));
#34672=CARTESIAN_POINT('Ctrl Pts',(47.7226369192852,41.7940371693788,19.9294657090004));
#34673=CARTESIAN_POINT('',(47.8907241605586,42.0945379161777,19.9294657090004));
#34674=CARTESIAN_POINT('Ctrl Pts',(47.8907241605586,42.0945379161777,19.9294657090003));
#34675=CARTESIAN_POINT('Ctrl Pts',(47.9804696976346,41.9438641629582,19.7757724373647));
#34676=CARTESIAN_POINT('Ctrl Pts',(48.0669218205059,41.7987197217834,19.6294657090004));
#34677=CARTESIAN_POINT('',(48.0596230081078,42.3695257957113,19.9294657090004));
#34678=CARTESIAN_POINT('Origin',(54.9397894030341,37.9543320991532,19.9294657090004));
#34679=CARTESIAN_POINT('',(48.4031440012129,42.3461303516745,19.6294657090004));
#34680=CARTESIAN_POINT('Ctrl Pts',(48.4031440012129,42.3461303516745,19.6294657090003));
#34681=CARTESIAN_POINT('Ctrl Pts',(48.2345939812314,42.3576094246832,19.7757724373647));
#34682=CARTESIAN_POINT('Ctrl Pts',(48.0596230081078,42.3695257957113,19.9294657090003));
#34683=CARTESIAN_POINT('',(48.251644553529,42.6553259804552,19.9294657090004));
#34684=CARTESIAN_POINT('Ctrl Pts',(48.251644553529,42.6553259804552,19.9294657090004));
#34685=CARTESIAN_POINT('Ctrl Pts',(48.3288101600596,42.4978384872912,19.7757724373647));
#34686=CARTESIAN_POINT('Ctrl Pts',(48.4031440012129,42.3461303516745,19.6294657090004));
#34687=CARTESIAN_POINT('',(48.4423954691411,42.9156320364489,19.9294657090004));
#34688=CARTESIAN_POINT('Origin',(54.9397894030341,37.9543320991532,19.9294657090004));
#34689=CARTESIAN_POINT('',(48.7828664785984,42.8643142887907,19.6294657090004));
#34690=CARTESIAN_POINT('Ctrl Pts',(48.7828664785984,42.8643142887908,19.6294657090004));
#34691=CARTESIAN_POINT('Ctrl Pts',(48.6158129459207,42.8894935575015,19.7757724373647));
#34692=CARTESIAN_POINT('Ctrl Pts',(48.4423954691411,42.9156320364489,19.9294657090003));
#34693=CARTESIAN_POINT('',(48.6570734470067,43.184829706062,19.9294657090004));
#34694=CARTESIAN_POINT('Ctrl Pts',(48.6570734470067,43.184829706062,19.9294657090003));
#34695=CARTESIAN_POINT('Ctrl Pts',(48.7211455986118,43.0215765262369,19.7757724373647));
#34696=CARTESIAN_POINT('Ctrl Pts',(48.7828664785984,42.8643142887907,19.6294657090003));
#34697=CARTESIAN_POINT('',(48.8684070148099,43.4287216446606,19.9294657090004));
#34698=CARTESIAN_POINT('Origin',(54.9397894030341,37.9543320991532,19.9294657090004));
#34699=CARTESIAN_POINT('',(49.2035622622253,43.349823104525,19.6294657090004));
#34700=CARTESIAN_POINT('Ctrl Pts',(49.2035622622253,43.349823104525,19.6294657090004));
#34701=CARTESIAN_POINT('Ctrl Pts',(49.0391169305495,43.3885350050588,19.7757724373647));
#34702=CARTESIAN_POINT('Ctrl Pts',(48.8684070148099,43.4287216446606,19.9294657090004));
#34703=CARTESIAN_POINT('',(49.1043127785965,43.6795253330662,19.9294657090004));
#34704=CARTESIAN_POINT('Ctrl Pts',(49.1043127785966,43.6795253330662,19.9294657090004));
#34705=CARTESIAN_POINT('Ctrl Pts',(49.1548650856785,43.5115928895569,19.7757724373647));
#34706=CARTESIAN_POINT('Ctrl Pts',(49.2035622622253,43.349823104525,19.6294657090004));
#34707=CARTESIAN_POINT('',(49.3348226085648,43.9053800936577,19.9294657090004));
#34708=CARTESIAN_POINT('Origin',(54.9397894030341,37.9543320991532,19.9294657090004));
#34709=CARTESIAN_POINT('',(49.6624316910633,43.7994258178118,19.6294657090004));
#34710=CARTESIAN_POINT('Ctrl Pts',(49.6624316910633,43.7994258178118,19.6294657090004));
#34711=CARTESIAN_POINT('Ctrl Pts',(49.5016889169402,43.8514127288577,19.7757724373647));
#34712=CARTESIAN_POINT('Ctrl Pts',(49.3348226085648,43.9053800936577,19.9294657090003));
#34713=CARTESIAN_POINT('',(49.5903862443362,44.1361207436891,19.9294657090004));
#34714=CARTESIAN_POINT('Ctrl Pts',(49.5903862443362,44.136120743689,19.9294657090004));
#34715=CARTESIAN_POINT('Ctrl Pts',(49.6270822896318,43.9646265992002,19.7757724373647));
#34716=CARTESIAN_POINT('Ctrl Pts',(49.6624316910633,43.7994258178118,19.6294657090004));
#34717=CARTESIAN_POINT('',(49.8385383315824,44.3424353001052,19.9294657090004));
#34718=CARTESIAN_POINT('Origin',(54.9397894030341,37.9543320991532,19.9294657090004));
#34719=CARTESIAN_POINT('',(50.1564210647719,44.2101303967736,19.6294657090004));
#34720=CARTESIAN_POINT('Ctrl Pts',(50.1564210647719,44.2101303967736,19.6294657090003));
#34721=CARTESIAN_POINT('Ctrl Pts',(50.0004505648425,44.2750463540157,19.7757724373647));
#34722=CARTESIAN_POINT('Ctrl Pts',(49.8385383315824,44.3424353001052,19.9294657090004));
#34723=CARTESIAN_POINT('',(50.1120591055075,44.5515773708059,19.9294657090004));
#34724=CARTESIAN_POINT('Ctrl Pts',(50.1120591055075,44.5515773708059,19.9294657090004));
#34725=CARTESIAN_POINT('Ctrl Pts',(50.1346546828898,44.3776627905745,19.7757724373647));
#34726=CARTESIAN_POINT('Ctrl Pts',(50.1564210647719,44.2101303967736,19.6294657090004));
#34727=CARTESIAN_POINT('',(50.3762020388334,44.7369787337131,19.9294657090004));
#34728=CARTESIAN_POINT('Origin',(54.9397894030341,37.9543320991532,19.9294657090004));
#34729=CARTESIAN_POINT('',(50.6822429655713,44.5792036701988,19.6294657090004));
#34730=CARTESIAN_POINT('Ctrl Pts',(50.6822429655713,44.5792036701988,19.6294657090004));
#34731=CARTESIAN_POINT('Ctrl Pts',(50.5320826977793,44.6566166686521,19.7757724373647));
#34732=CARTESIAN_POINT('Ctrl Pts',(50.3762020388334,44.7369787337131,19.9294657090004));
#34733=CARTESIAN_POINT('',(50.6658597152895,44.9231304191087,19.9294657090004));
#34734=CARTESIAN_POINT('Ctrl Pts',(50.6658597152895,44.9231304191087,19.9294657090004));
#34735=CARTESIAN_POINT('Ctrl Pts',(50.674204454919,44.7479527759724,19.7757724373647));
#34736=CARTESIAN_POINT('Ctrl Pts',(50.6822429655713,44.5792036701988,19.6294657090004));
#34737=CARTESIAN_POINT('',(50.9442356670542,45.086384773026,19.9294657090004));
#34738=CARTESIAN_POINT('Origin',(54.9397894030341,37.9543320991532,19.9294657090004));
#34739=CARTESIAN_POINT('',(51.2363981354663,44.9041895163455,19.6294657090004));
#34740=CARTESIAN_POINT('Ctrl Pts',(51.2363981354663,44.9041895163455,19.6294657090004));
#34741=CARTESIAN_POINT('Ctrl Pts',(51.0930473916193,44.9935843852776,19.7757724373647));
#34742=CARTESIAN_POINT('Ctrl Pts',(50.9442356670542,45.0863847730261,19.9294657090004));
#34743=CARTESIAN_POINT('',(51.2481026219946,45.2483072643631,19.9294657090004));
#34744=CARTESIAN_POINT('Ctrl Pts',(51.2481026219946,45.2483072643631,19.9294657090004));
#34745=CARTESIAN_POINT('Ctrl Pts',(51.2421409910059,45.0730323366345,19.7757724373647));
#34746=CARTESIAN_POINT('Ctrl Pts',(51.2363981354663,44.9041895163455,19.6294657090003));
#34747=CARTESIAN_POINT('',(51.5388590461679,45.3883281785002,19.9294657090004));
#34748=CARTESIAN_POINT('Origin',(54.9397894030341,37.9543320991532,19.9294657090004));
#34749=CARTESIAN_POINT('',(51.8151987632305,45.1829252080266,19.6294657090004));
#34750=CARTESIAN_POINT('Ctrl Pts',(51.8151987632305,45.1829252080266,19.6294657090003));
#34751=CARTESIAN_POINT('Ctrl Pts',(51.6796115188774,45.2837070393337,19.7757724373647));
#34752=CARTESIAN_POINT('Ctrl Pts',(51.538859046168,45.3883281785002,19.9294657090003));
#34753=CARTESIAN_POINT('',(51.8549130951421,45.5249439083141,19.9294657090004));
#34754=CARTESIAN_POINT('Ctrl Pts',(51.8549130951421,45.5249439083141,19.9294657090004));
#34755=CARTESIAN_POINT('Ctrl Pts',(51.8346847672058,45.3507381217191,19.7757724373647));
#34756=CARTESIAN_POINT('Ctrl Pts',(51.8151987632305,45.1829252080266,19.6294657090004));
#34757=CARTESIAN_POINT('',(52.1561150556927,45.6407995665893,19.9294657090004));
#34758=CARTESIAN_POINT('Origin',(54.9397894030341,37.9543320991532,19.9294657090004));
#34759=CARTESIAN_POINT('',(52.4147930261813,45.413555805202,19.6294657090004));
#34760=CARTESIAN_POINT('Ctrl Pts',(52.4147930261813,45.413555805202,19.6294657090003));
#34761=CARTESIAN_POINT('Ctrl Pts',(52.2878715920631,45.5250539124247,19.7757724373647));
#34762=CARTESIAN_POINT('Ctrl Pts',(52.1561150556927,45.6407995665893,19.9294657090004));
#34763=CARTESIAN_POINT('',(52.4822529111499,45.7511993797382,19.9294657090004));
#34764=CARTESIAN_POINT('Ctrl Pts',(52.4822529111499,45.7511993797382,19.9294657090003));
#34765=CARTESIAN_POINT('Ctrl Pts',(52.447892502451,45.5792220450446,19.7757724373647));
#34766=CARTESIAN_POINT('Ctrl Pts',(52.4147930261813,45.413555805202,19.6294657090003));
#34767=CARTESIAN_POINT('',(52.791895958725,45.8421187818605,19.9294657090004));
#34768=CARTESIAN_POINT('Origin',(54.9397894030341,37.9543320991532,19.9294657090004));
#34769=CARTESIAN_POINT('',(53.0311907234251,45.594546499299,19.6294657090004));
#34770=CARTESIAN_POINT('Ctrl Pts',(53.0311907234251,45.594546499299,19.6294657090003));
#34771=CARTESIAN_POINT('Ctrl Pts',(52.9137797407451,45.7160188809296,19.7757724373647));
#34772=CARTESIAN_POINT('Ctrl Pts',(52.791895958725,45.8421187818605,19.9294657090003));
#34773=CARTESIAN_POINT('',(53.1259472270462,45.9255679858026,19.9294657090004));
#34774=CARTESIAN_POINT('Ctrl Pts',(53.1259472270462,45.9255679858026,19.9294657090004));
#34775=CARTESIAN_POINT('Ctrl Pts',(53.0776834004354,45.7569635837984,19.7757724373647));
#34776=CARTESIAN_POINT('Ctrl Pts',(53.0311907234251,45.594546499299,19.6294657090004));
#34777=CARTESIAN_POINT('',(53.4419707382517,45.9909460781514,19.9294657090004));
#34778=CARTESIAN_POINT('Origin',(54.9397894030341,37.9543320991532,19.9294657090004));
#34779=CARTESIAN_POINT('',(53.660289829985,45.7246928271096,19.6294657090004));
#34780=CARTESIAN_POINT('Ctrl Pts',(53.660289829985,45.7246928271096,19.6294657090003));
#34781=CARTESIAN_POINT('Ctrl Pts',(53.5531706494617,45.8553311044899,19.7757724373647));
#34782=CARTESIAN_POINT('Ctrl Pts',(53.4419707382517,45.9909460781514,19.9294657090003));
#34783=CARTESIAN_POINT('',(53.7817123633608,46.0468893322027,19.9294657090004));
#34784=CARTESIAN_POINT('Ctrl Pts',(53.7817123633608,46.0468893322027,19.9294657090003));
#34785=CARTESIAN_POINT('Ctrl Pts',(53.7198663066414,45.8827798973656,19.7757724373647));
#34786=CARTESIAN_POINT('Ctrl Pts',(53.660289829985,45.7246928271096,19.6294657090003));
#34787=CARTESIAN_POINT('',(54.1020132538699,46.0862910343601,19.9294657090004));
#34788=CARTESIAN_POINT('Origin',(54.9397894030341,37.9543320991532,19.9294657090004));
#34789=CARTESIAN_POINT('',(54.297903795101,45.803128686295,19.6294657090004));
#34790=CARTESIAN_POINT('Ctrl Pts',(54.297903795101,45.803128686295,19.6294657090004));
#34791=CARTESIAN_POINT('Ctrl Pts',(54.2017892772072,45.9420634832428,19.7757724373647));
#34792=CARTESIAN_POINT('Ctrl Pts',(54.1020132538699,46.0862910343602,19.9294657090004));
#34793=CARTESIAN_POINT('',(54.4451843113051,46.1143560453948,19.9294657090004));
#34794=CARTESIAN_POINT('Ctrl Pts',(54.4451843113051,46.1143560453948,19.9294657090003));
#34795=CARTESIAN_POINT('Ctrl Pts',(54.3701675997806,45.9558336989374,19.7757724373647));
#34796=CARTESIAN_POINT('Ctrl Pts',(54.297903795101,45.803128686295,19.6294657090003));
#34797=CARTESIAN_POINT('',(54.7676310315374,46.1275191455338,19.9294657090004));
#34798=CARTESIAN_POINT('Origin',(54.9397894030341,37.9543320991532,19.9294657090004));
#34799=CARTESIAN_POINT('',(54.9397894030341,45.8293320991532,19.6294657090004));
#34800=CARTESIAN_POINT('Ctrl Pts',(54.9397894030341,45.8293320991532,19.6294657090003));
#34801=CARTESIAN_POINT('Ctrl Pts',(54.8553191740287,45.9756388275175,19.7757724373647));
#34802=CARTESIAN_POINT('Ctrl Pts',(54.7676310315374,46.1275191455338,19.9294657090003));
#34803=CARTESIAN_POINT('',(55.1119477745308,46.1275191455338,19.9294657090004));
#34804=CARTESIAN_POINT('Ctrl Pts',(55.1119477745308,46.1275191455338,19.9294657090003));
#34805=CARTESIAN_POINT('Ctrl Pts',(55.0242596320395,45.9756388275175,19.7757724373647));
#34806=CARTESIAN_POINT('Ctrl Pts',(54.9397894030341,45.8293320991532,19.6294657090003));
#34807=CARTESIAN_POINT('',(55.434394494763,46.1143560453948,19.9294657090004));
#34808=CARTESIAN_POINT('Origin',(54.9397894030341,37.9543320991532,19.9294657090004));
#34809=CARTESIAN_POINT('',(55.5816750109672,45.803128686295,19.6294657090004));
#34810=CARTESIAN_POINT('Ctrl Pts',(55.5816750109672,45.803128686295,19.6294657090004));
#34811=CARTESIAN_POINT('Ctrl Pts',(55.5094112062876,45.9558336989374,19.7757724373647));
#34812=CARTESIAN_POINT('Ctrl Pts',(55.434394494763,46.1143560453948,19.9294657090003));
#34813=CARTESIAN_POINT('',(55.7775655521983,46.0862910343602,19.9294657090004));
#34814=CARTESIAN_POINT('Ctrl Pts',(55.7775655521983,46.0862910343601,19.9294657090004));
#34815=CARTESIAN_POINT('Ctrl Pts',(55.6777895288609,45.9420634832429,19.7757724373647));
#34816=CARTESIAN_POINT('Ctrl Pts',(55.5816750109672,45.803128686295,19.6294657090003));
#34817=CARTESIAN_POINT('',(56.0978664427074,46.0468893322027,19.9294657090004));
#34818=CARTESIAN_POINT('Origin',(54.9397894030341,37.9543320991532,19.9294657090004));
#34819=CARTESIAN_POINT('',(56.2192889760832,45.7246928271096,19.6294657090004));
#34820=CARTESIAN_POINT('Ctrl Pts',(56.2192889760832,45.7246928271096,19.6294657090004));
#34821=CARTESIAN_POINT('Ctrl Pts',(56.1597124994268,45.8827798973656,19.7757724373647));
#34822=CARTESIAN_POINT('Ctrl Pts',(56.0978664427074,46.0468893322027,19.9294657090004));
#34823=CARTESIAN_POINT('',(56.4376080678164,45.9909460781515,19.9294657090004));
#34824=CARTESIAN_POINT('Ctrl Pts',(56.4376080678164,45.9909460781515,19.9294657090004));
#34825=CARTESIAN_POINT('Ctrl Pts',(56.3264081566065,45.85533110449,19.7757724373647));
#34826=CARTESIAN_POINT('Ctrl Pts',(56.2192889760832,45.7246928271096,19.6294657090004));
#34827=CARTESIAN_POINT('',(56.753631579022,45.9255679858027,19.9294657090004));
#34828=CARTESIAN_POINT('Origin',(54.9397894030341,37.9543320991532,19.9294657090004));
#34829=CARTESIAN_POINT('',(56.8483880826431,45.594546499299,19.6294657090004));
#34830=CARTESIAN_POINT('Ctrl Pts',(56.8483880826431,45.594546499299,19.6294657090003));
#34831=CARTESIAN_POINT('Ctrl Pts',(56.8018954056327,45.7569635837985,19.7757724373647));
#34832=CARTESIAN_POINT('Ctrl Pts',(56.753631579022,45.9255679858026,19.9294657090003));
#34833=CARTESIAN_POINT('',(57.0876828473432,45.8421187818605,19.9294657090004));
#34834=CARTESIAN_POINT('Ctrl Pts',(57.0876828473432,45.8421187818605,19.9294657090003));
#34835=CARTESIAN_POINT('Ctrl Pts',(56.965799065323,45.7160188809296,19.7757724373647));
#34836=CARTESIAN_POINT('Ctrl Pts',(56.8483880826431,45.594546499299,19.6294657090003));
#34837=CARTESIAN_POINT('',(57.3973258949183,45.7511993797383,19.9294657090004));
#34838=CARTESIAN_POINT('Origin',(54.9397894030341,37.9543320991532,19.9294657090004));
#34839=CARTESIAN_POINT('',(57.4647857798868,45.413555805202,19.6294657090004));
#34840=CARTESIAN_POINT('Ctrl Pts',(57.4647857798868,45.413555805202,19.6294657090003));
#34841=CARTESIAN_POINT('Ctrl Pts',(57.4316863036172,45.5792220450446,19.7757724373647));
#34842=CARTESIAN_POINT('Ctrl Pts',(57.3973258949183,45.7511993797383,19.9294657090003));
#34843=CARTESIAN_POINT('',(57.7234637503755,45.6407995665893,19.9294657090004));
#34844=CARTESIAN_POINT('Ctrl Pts',(57.7234637503755,45.6407995665893,19.9294657090004));
#34845=CARTESIAN_POINT('Ctrl Pts',(57.5917072140051,45.5250539124248,19.7757724373647));
#34846=CARTESIAN_POINT('Ctrl Pts',(57.4647857798868,45.413555805202,19.6294657090003));
#34847=CARTESIAN_POINT('',(58.024665710926,45.5249439083142,19.9294657090004));
#34848=CARTESIAN_POINT('Origin',(54.9397894030341,37.9543320991532,19.9294657090004));
#34849=CARTESIAN_POINT('',(58.0643800428377,45.1829252080266,19.6294657090004));
#34850=CARTESIAN_POINT('Ctrl Pts',(58.0643800428377,45.1829252080266,19.6294657090004));
#34851=CARTESIAN_POINT('Ctrl Pts',(58.0448940388624,45.3507381217191,19.7757724373647));
#34852=CARTESIAN_POINT('Ctrl Pts',(58.024665710926,45.5249439083142,19.9294657090003));
#34853=CARTESIAN_POINT('',(58.3407197599002,45.3883281785002,19.9294657090004));
#34854=CARTESIAN_POINT('Ctrl Pts',(58.3407197599002,45.3883281785002,19.9294657090003));
#34855=CARTESIAN_POINT('Ctrl Pts',(58.1999672871908,45.2837070393338,19.7757724373647));
#34856=CARTESIAN_POINT('Ctrl Pts',(58.0643800428377,45.1829252080266,19.6294657090003));
#34857=CARTESIAN_POINT('',(58.6314761840736,45.2483072643631,19.9294657090004));
#34858=CARTESIAN_POINT('Origin',(54.9397894030341,37.9543320991532,19.9294657090004));
#34859=CARTESIAN_POINT('',(58.6431806706019,44.9041895163456,19.6294657090004));
#34860=CARTESIAN_POINT('Ctrl Pts',(58.6431806706019,44.9041895163456,19.6294657090004));
#34861=CARTESIAN_POINT('Ctrl Pts',(58.6374378150623,45.0730323366346,19.7757724373647));
#34862=CARTESIAN_POINT('Ctrl Pts',(58.6314761840736,45.2483072643631,19.9294657090003));
#34863=CARTESIAN_POINT('',(58.935343139014,45.0863847730261,19.9294657090004));
#34864=CARTESIAN_POINT('Ctrl Pts',(58.935343139014,45.0863847730261,19.9294657090003));
#34865=CARTESIAN_POINT('Ctrl Pts',(58.7865314144489,44.9935843852776,19.7757724373647));
#34866=CARTESIAN_POINT('Ctrl Pts',(58.6431806706019,44.9041895163456,19.6294657090004));
#34867=CARTESIAN_POINT('',(59.2137190907787,44.9231304191088,19.9294657090004));
#34868=CARTESIAN_POINT('Origin',(54.9397894030341,37.9543320991532,19.9294657090004));
#34869=CARTESIAN_POINT('',(59.1973358404969,44.5792036701988,19.6294657090004));
#34870=CARTESIAN_POINT('Ctrl Pts',(59.1973358404969,44.5792036701988,19.6294657090003));
#34871=CARTESIAN_POINT('Ctrl Pts',(59.2053743511492,44.7479527759724,19.7757724373647));
#34872=CARTESIAN_POINT('Ctrl Pts',(59.2137190907787,44.9231304191088,19.9294657090003));
#34873=CARTESIAN_POINT('',(59.5033767672348,44.7369787337132,19.9294657090004));
#34874=CARTESIAN_POINT('Ctrl Pts',(59.5033767672348,44.7369787337132,19.9294657090003));
#34875=CARTESIAN_POINT('Ctrl Pts',(59.3474961082889,44.6566166686521,19.7757724373647));
#34876=CARTESIAN_POINT('Ctrl Pts',(59.1973358404969,44.5792036701988,19.6294657090003));
#34877=CARTESIAN_POINT('',(59.7675197005607,44.551577370806,19.9294657090004));
#34878=CARTESIAN_POINT('Origin',(54.9397894030341,37.9543320991532,19.9294657090004));
#34879=CARTESIAN_POINT('',(59.7231577412963,44.2101303967737,19.6294657090004));
#34880=CARTESIAN_POINT('Ctrl Pts',(59.7231577412963,44.2101303967737,19.6294657090003));
#34881=CARTESIAN_POINT('Ctrl Pts',(59.7449241231784,44.3776627905746,19.7757724373647));
#34882=CARTESIAN_POINT('Ctrl Pts',(59.7675197005607,44.551577370806,19.9294657090003));
#34883=CARTESIAN_POINT('',(60.0410404744858,44.3424353001052,19.9294657090004));
#34884=CARTESIAN_POINT('Ctrl Pts',(60.0410404744858,44.3424353001052,19.9294657090003));
#34885=CARTESIAN_POINT('Ctrl Pts',(59.8791282412257,44.2750463540158,19.7757724373647));
#34886=CARTESIAN_POINT('Ctrl Pts',(59.7231577412963,44.2101303967737,19.6294657090003));
#34887=CARTESIAN_POINT('',(60.289192561732,44.1361207436891,19.9294657090004));
#34888=CARTESIAN_POINT('Origin',(54.9397894030341,37.9543320991532,19.9294657090004));
#34889=CARTESIAN_POINT('',(60.2171471150049,43.7994258178119,19.6294657090004));
#34890=CARTESIAN_POINT('Ctrl Pts',(60.2171471150049,43.7994258178119,19.6294657090003));
#34891=CARTESIAN_POINT('Ctrl Pts',(60.2524965164364,43.9646265992003,19.7757724373647));
#34892=CARTESIAN_POINT('Ctrl Pts',(60.289192561732,44.1361207436891,19.9294657090004));
#34893=CARTESIAN_POINT('',(60.5447561975034,43.9053800936578,19.9294657090004));
#34894=CARTESIAN_POINT('Ctrl Pts',(60.5447561975034,43.9053800936578,19.9294657090003));
#34895=CARTESIAN_POINT('Ctrl Pts',(60.377889889128,43.8514127288578,19.7757724373647));
#34896=CARTESIAN_POINT('Ctrl Pts',(60.2171471150048,43.7994258178119,19.6294657090003));
#34897=CARTESIAN_POINT('',(60.7752660274717,43.6795253330662,19.9294657090004));
#34898=CARTESIAN_POINT('Origin',(54.9397894030341,37.9543320991532,19.9294657090004));
#34899=CARTESIAN_POINT('',(60.6760165438429,43.3498231045251,19.6294657090004));
#34900=CARTESIAN_POINT('Ctrl Pts',(60.6760165438429,43.3498231045251,19.6294657090004));
#34901=CARTESIAN_POINT('Ctrl Pts',(60.7247137203897,43.511592889557,19.7757724373647));
#34902=CARTESIAN_POINT('Ctrl Pts',(60.7752660274716,43.6795253330662,19.9294657090004));
#34903=CARTESIAN_POINT('',(61.0111717912583,43.4287216446607,19.9294657090004));
#34904=CARTESIAN_POINT('Ctrl Pts',(61.0111717912583,43.4287216446607,19.9294657090003));
#34905=CARTESIAN_POINT('Ctrl Pts',(60.8404618755187,43.3885350050589,19.7757724373647));
#34906=CARTESIAN_POINT('Ctrl Pts',(60.6760165438429,43.3498231045251,19.6294657090003));
#34907=CARTESIAN_POINT('',(61.2225053590615,43.184829706062,19.9294657090004));
#34908=CARTESIAN_POINT('Origin',(54.9397894030341,37.9543320991532,19.9294657090004));
#34909=CARTESIAN_POINT('',(61.0967123274698,42.8643142887908,19.6294657090004));
#34910=CARTESIAN_POINT('Ctrl Pts',(61.0967123274698,42.8643142887908,19.6294657090004));
#34911=CARTESIAN_POINT('Ctrl Pts',(61.1584332074564,43.021576526237,19.7757724373647));
#34912=CARTESIAN_POINT('Ctrl Pts',(61.2225053590615,43.184829706062,19.9294657090003));
#34913=CARTESIAN_POINT('',(61.4371833369271,42.915632036449,19.9294657090004));
#34914=CARTESIAN_POINT('Ctrl Pts',(61.4371833369271,42.915632036449,19.9294657090004));
#34915=CARTESIAN_POINT('Ctrl Pts',(61.2637658601475,42.8894935575016,19.7757724373647));
#34916=CARTESIAN_POINT('Ctrl Pts',(61.0967123274698,42.8643142887908,19.6294657090003));
#34917=CARTESIAN_POINT('',(61.6279342525392,42.6553259804552,19.9294657090004));
#34918=CARTESIAN_POINT('Origin',(54.9397894030341,37.9543320991532,19.9294657090004));
#34919=CARTESIAN_POINT('',(61.4764348048553,42.3461303516746,19.6294657090004));
#34920=CARTESIAN_POINT('Ctrl Pts',(61.4764348048554,42.3461303516746,19.6294657090003));
#34921=CARTESIAN_POINT('Ctrl Pts',(61.5507686460086,42.4978384872913,19.7757724373647));
#34922=CARTESIAN_POINT('Ctrl Pts',(61.6279342525392,42.6553259804552,19.9294657090003));
#34923=CARTESIAN_POINT('',(61.8199557979604,42.3695257957114,19.9294657090004));
#34924=CARTESIAN_POINT('Ctrl Pts',(61.8199557979604,42.3695257957114,19.9294657090004));
#34925=CARTESIAN_POINT('Ctrl Pts',(61.6449848248368,42.3576094246833,19.7757724373647));
#34926=CARTESIAN_POINT('Ctrl Pts',(61.4764348048553,42.3461303516746,19.6294657090003));
#34927=CARTESIAN_POINT('',(61.9888546455096,42.0945379161778,19.9294657090004));
#34928=CARTESIAN_POINT('Origin',(54.9397894030341,37.9543320991532,19.9294657090004));
#34929=CARTESIAN_POINT('',(61.8126569855623,41.7987197217835,19.6294657090004));
#34930=CARTESIAN_POINT('Ctrl Pts',(61.8126569855623,41.7987197217835,19.6294657090004));
#34931=CARTESIAN_POINT('Ctrl Pts',(61.8991091084337,41.9438641629583,19.7757724373647));
#34932=CARTESIAN_POINT('Ctrl Pts',(61.9888546455096,42.0945379161778,19.9294657090003));
#34933=CARTESIAN_POINT('',(62.1569418867831,41.7940371693789,19.9294657090004));
#34934=CARTESIAN_POINT('Ctrl Pts',(62.156941886783,41.7940371693789,19.9294657090003));
#34935=CARTESIAN_POINT('Ctrl Pts',(61.9815818202734,41.7964222077532,19.7757724373647));
#34936=CARTESIAN_POINT('Ctrl Pts',(61.8126569855623,41.7987197217835,19.6294657090003));
#34937=CARTESIAN_POINT('',(62.3028646723053,41.5061974652739,19.9294657090004));
#34938=CARTESIAN_POINT('Origin',(54.9397894030341,37.9543320991532,19.9294657090004));
#34939=CARTESIAN_POINT('',(62.1031413664509,41.2257253265432,19.6294657090004));
#34940=CARTESIAN_POINT('Ctrl Pts',(62.1031413664509,41.2257253265432,19.6294657090004));
#34941=CARTESIAN_POINT('Ctrl Pts',(62.2011364464262,41.3633401609671,19.7757724373647));
#34942=CARTESIAN_POINT('Ctrl Pts',(62.3028646723053,41.5061974652739,19.9294657090004));
#34943=CARTESIAN_POINT('',(62.4458990165727,41.1929959393108,19.9294657090004));
#34944=CARTESIAN_POINT('Ctrl Pts',(62.4458990165727,41.1929959393108,19.9294657090003));
#34945=CARTESIAN_POINT('Ctrl Pts',(62.2713168489873,41.2096665150507,19.7757724373647));
#34946=CARTESIAN_POINT('Ctrl Pts',(62.1031413664509,41.2257253265432,19.6294657090003));
#34947=CARTESIAN_POINT('',(62.5678746480059,40.894219936375,19.9294657090004));
#34948=CARTESIAN_POINT('Origin',(54.9397894030341,37.9543320991532,19.9294657090004));
#34949=CARTESIAN_POINT('',(62.3459548218929,40.6309603491164,19.6294657090004));
#34950=CARTESIAN_POINT('Ctrl Pts',(62.3459548218929,40.6309603491164,19.6294657090004));
#34951=CARTESIAN_POINT('Ctrl Pts',(62.4548407178829,40.7601297727713,19.7757724373647));
#34952=CARTESIAN_POINT('Ctrl Pts',(62.5678746480059,40.894219936375,19.9294657090004));
#34953=CARTESIAN_POINT('',(62.6849042253051,40.5704019357284,19.9294657090004));
#34954=CARTESIAN_POINT('Ctrl Pts',(62.6849042253051,40.5704019357284,19.9294657090004));
#34955=CARTESIAN_POINT('Ctrl Pts',(62.5122617721652,40.6012471089027,19.7757724373647));
#34956=CARTESIAN_POINT('Ctrl Pts',(62.3459548218929,40.6309603491164,19.6294657090004));
#34957=CARTESIAN_POINT('',(62.7821209749467,40.2626779389667,19.9294657090004));
#34958=CARTESIAN_POINT('Origin',(54.9397894030341,37.9543320991532,19.9294657090004));
#34959=CARTESIAN_POINT('',(62.5394814684036,40.0183828522987,19.6294657090004));
#34960=CARTESIAN_POINT('Ctrl Pts',(62.5394814684036,40.0183828522987,19.6294657090003));
#34961=CARTESIAN_POINT('Ctrl Pts',(62.6585335627355,40.1382472639816,19.7757724373647));
#34962=CARTESIAN_POINT('Ctrl Pts',(62.7821209749466,40.2626779389667,19.9294657090004));
#34963=CARTESIAN_POINT('',(62.8723669727493,39.9303984190047,19.9294657090004));
#34964=CARTESIAN_POINT('Ctrl Pts',(62.8723669727493,39.9303984190047,19.9294657090003));
#34965=CARTESIAN_POINT('Ctrl Pts',(62.7028131410966,39.9752129200751,19.7757724373647));
#34966=CARTESIAN_POINT('Ctrl Pts',(62.5394814684036,40.0183828522987,19.6294657090003));
#34967=CARTESIAN_POINT('',(62.94417787917,39.6157742808448,19.9294657090004));
#34968=CARTESIAN_POINT('Origin',(54.9397894030341,37.9543320991532,19.9294657090004));
#34969=CARTESIAN_POINT('',(62.6824334180802,39.3920694382633,19.6294657090004));
#34970=CARTESIAN_POINT('Ctrl Pts',(62.6824334180802,39.3920694382633,19.6294657090003));
#34971=CARTESIAN_POINT('Ctrl Pts',(62.8108594387083,39.5018311600907,19.7757724373647));
#34972=CARTESIAN_POINT('Ctrl Pts',(62.94417787917,39.6157742808448,19.9294657090003));
#34973=CARTESIAN_POINT('',(63.0070397252503,39.2772445069504,19.9294657090004));
#34974=CARTESIAN_POINT('Ctrl Pts',(63.0070397252503,39.2772445069504,19.9294657090004));
#34975=CARTESIAN_POINT('Ctrl Pts',(62.8417028678599,39.335730102806,19.7757724373647));
#34976=CARTESIAN_POINT('Ctrl Pts',(62.6824334180802,39.3920694382633,19.6294657090003));
#34977=CARTESIAN_POINT('',(63.0529668987158,38.9578139991223,19.9294657090004));
#34978=CARTESIAN_POINT('Origin',(54.9397894030341,37.9543320991532,19.9294657090004));
#34979=CARTESIAN_POINT('',(62.773859349283,38.756188119446,19.6294657090004));
#34980=CARTESIAN_POINT('Ctrl Pts',(62.773859349283,38.756188119446,19.6294657090003));
#34981=CARTESIAN_POINT('Ctrl Pts',(62.910804642229,38.8551167052685,19.7757724373647));
#34982=CARTESIAN_POINT('Ctrl Pts',(63.0529668987157,38.9578139991223,19.9294657090004));
#34983=CARTESIAN_POINT('',(63.0880262578595,38.6152868310874,19.9294657090004));
#34984=CARTESIAN_POINT('Ctrl Pts',(63.0880262578595,38.6152868310874,19.9294657090003));
#34985=CARTESIAN_POINT('Ctrl Pts',(62.9280066642388,38.6870543097374,19.7757724373647));
#34986=CARTESIAN_POINT('Ctrl Pts',(62.773859349283,38.756188119446,19.6294657090004));
#34987=CARTESIAN_POINT('',(63.1077640606078,38.2931757109184,19.9294657090004));
#34988=CARTESIAN_POINT('Origin',(54.9397894030341,37.9543320991532,19.9294657090004));
#34989=CARTESIAN_POINT('Ctrl Pts',(62.8131508375241,38.1149705811106,19.6294657090003));
#34990=CARTESIAN_POINT('Ctrl Pts',(62.9577040544577,38.2024076775117,19.7757724373647));
#34991=CARTESIAN_POINT('Ctrl Pts',(63.1077640606078,38.2931757109184,19.9294657090003));
#34992=CARTESIAN_POINT('Origin',(54.9397894030341,37.9543320991532,22.6294657090004));
#34993=CARTESIAN_POINT('',(47.0664279685441,38.1149705811105,22.9294657090004));
#34994=CARTESIAN_POINT('',(46.764791187504,37.9489306105331,22.6294657090004));
#34995=CARTESIAN_POINT('Ctrl Pts',(46.764791187504,37.9489306105332,22.6294657090004));
#34996=CARTESIAN_POINT('Ctrl Pts',(46.9184286133609,38.0335023712478,22.783158980636));
#34997=CARTESIAN_POINT('Ctrl Pts',(47.0664279685441,38.1149705811105,22.9294657090004));
#34998=CARTESIAN_POINT('',(46.7713741072936,37.6262824743834,22.6294657090004));
#34999=CARTESIAN_POINT('Origin',(54.9397894030341,37.9543320991532,22.6294657090004));
#35000=CARTESIAN_POINT('',(47.0795324016364,37.4726840201812,22.9294657090004));
#35001=CARTESIAN_POINT('Ctrl Pts',(46.7713741072936,37.6262824743834,22.6294657090004));
#35002=CARTESIAN_POINT('Ctrl Pts',(46.9283332385242,37.5480477477103,22.783158980636));
#35003=CARTESIAN_POINT('Ctrl Pts',(47.0795324016364,37.4726840201812,22.9294657090004));
#35004=CARTESIAN_POINT('',(46.7924330911438,37.2826103359946,22.6294657090004));
#35005=CARTESIAN_POINT('Ctrl Pts',(47.0795324016364,37.4726840201812,22.9294657090003));
#35006=CARTESIAN_POINT('Ctrl Pts',(46.9386659175162,37.3794235676597,22.783158980636));
#35007=CARTESIAN_POINT('Ctrl Pts',(46.7924330911438,37.2826103359945,22.6294657090004));
#35008=CARTESIAN_POINT('',(46.8252929252262,36.961572353977,22.6294657090004));
#35009=CARTESIAN_POINT('Origin',(54.9397894030341,37.9543320991532,22.6294657090004));
#35010=CARTESIAN_POINT('',(47.1449455482218,36.8336027477511,22.9294657090004));
#35011=CARTESIAN_POINT('Ctrl Pts',(46.8252929252262,36.961572353977,22.6294657090004));
#35012=CARTESIAN_POINT('Ctrl Pts',(46.9881066444155,36.8963915732357,22.783158980636));
#35013=CARTESIAN_POINT('Ctrl Pts',(47.1449455482218,36.8336027477511,22.9294657090004));
#35014=CARTESIAN_POINT('',(46.8742943068201,36.6207602589635,22.6294657090004));
#35015=CARTESIAN_POINT('Ctrl Pts',(47.1449455482218,36.8336027477511,22.9294657090004));
#35016=CARTESIAN_POINT('Ctrl Pts',(47.0121493783752,36.7291706854955,22.783158980636));
#35017=CARTESIAN_POINT('Ctrl Pts',(46.8742943068201,36.6207602589635,22.6294657090004));
#35018=CARTESIAN_POINT('',(46.9332123784209,36.3034688858808,22.6294657090004));
#35019=CARTESIAN_POINT('Origin',(54.9397894030341,37.9543320991532,22.6294657090004));
#35020=CARTESIAN_POINT('',(47.2622320946023,36.2019797442472,22.9294657090004));
#35021=CARTESIAN_POINT('Ctrl Pts',(46.9332123784209,36.3034688858808,22.6294657090004));
#35022=CARTESIAN_POINT('Ctrl Pts',(47.1007971871301,36.2517758184132,22.783158980636));
#35023=CARTESIAN_POINT('Ctrl Pts',(47.2622320946023,36.2019797442472,22.9294657090004));
#35024=CARTESIAN_POINT('',(47.0098300616486,35.967784882505,22.6294657090004));
#35025=CARTESIAN_POINT('Ctrl Pts',(47.2622320946023,36.2019797442472,22.9294657090004));
#35026=CARTESIAN_POINT('Ctrl Pts',(47.1383899756297,36.0870710504017,22.7831589806361));
#35027=CARTESIAN_POINT('Ctrl Pts',(47.0098300616486,35.967784882505,22.6294657090004));
#35028=CARTESIAN_POINT('',(47.0944142807223,35.6563516400958,22.6294657090004));
#35029=CARTESIAN_POINT('Origin',(54.9397894030341,37.9543320991532,22.6294657090004));
#35030=CARTESIAN_POINT('',(47.4306115181626,35.5820183565475,22.9294657090004));
#35031=CARTESIAN_POINT('Ctrl Pts',(47.0944142807223,35.6563516400958,22.6294657090004));
#35032=CARTESIAN_POINT('Ctrl Pts',(47.2656549296989,35.6184902947371,22.783158980636));
#35033=CARTESIAN_POINT('Ctrl Pts',(47.4306115181626,35.5820183565475,22.9294657090004));
#35034=CARTESIAN_POINT('',(47.1981383875429,35.3280296500161,22.6294657090004));
#35035=CARTESIAN_POINT('Ctrl Pts',(47.4306115181626,35.5820183565475,22.9294657090004));
#35036=CARTESIAN_POINT('Ctrl Pts',(47.3165475989333,35.4573977295111,22.783158980636));
#35037=CARTESIAN_POINT('Ctrl Pts',(47.1981383875429,35.3280296500161,22.6294657090004));
#35038=CARTESIAN_POINT('',(47.3078258600668,35.0245270751256,22.6294657090004));
#35039=CARTESIAN_POINT('Origin',(54.9397894030341,37.9543320991532,22.6294657090004));
#35040=CARTESIAN_POINT('',(47.6489632816196,34.9778443254006,22.9294657090004));
#35041=CARTESIAN_POINT('Ctrl Pts',(47.3078258600668,35.0245270751256,22.6294657090004));
#35042=CARTESIAN_POINT('Ctrl Pts',(47.4815827710446,35.0007494128825,22.783158980636));
#35043=CARTESIAN_POINT('Ctrl Pts',(47.6489632816196,34.9778443254006,22.9294657090004));
#35044=CARTESIAN_POINT('',(47.4379661236627,34.7057520270169,22.6294657090004));
#35045=CARTESIAN_POINT('Ctrl Pts',(47.6489632816196,34.9778443254006,22.9294657090004));
#35046=CARTESIAN_POINT('Ctrl Pts',(47.5454366386968,34.8443410948852,22.7831589806361));
#35047=CARTESIAN_POINT('Ctrl Pts',(47.4379661236628,34.7057520270169,22.6294657090004));
#35048=CARTESIAN_POINT('',(47.5720268976044,34.4121998792066,22.6294657090004));
#35049=CARTESIAN_POINT('Origin',(54.9397894030341,37.9543320991532,22.6294657090004));
#35050=CARTESIAN_POINT('',(47.9158342900129,34.393478329302,22.9294657090004));
#35051=CARTESIAN_POINT('Ctrl Pts',(47.5720268976044,34.4121998792066,22.6294657090004));
#35052=CARTESIAN_POINT('Ctrl Pts',(47.7471437470088,34.4026641364982,22.783158980636));
#35053=CARTESIAN_POINT('Ctrl Pts',(47.9158342900129,34.393478329302,22.9294657090004));
#35054=CARTESIAN_POINT('',(47.7277172559931,34.1050931684197,22.6294657090004));
#35055=CARTESIAN_POINT('Ctrl Pts',(47.9158342900129,34.393478329302,22.9294657090004));
#35056=CARTESIAN_POINT('Ctrl Pts',(47.8235338761247,34.2519809372803,22.783158980636));
#35057=CARTESIAN_POINT('Ctrl Pts',(47.7277172559931,34.1050931684197,22.6294657090004));
#35058=CARTESIAN_POINT('',(47.8852591790204,33.8234449888006,22.6294657090004));
#35059=CARTESIAN_POINT('Origin',(54.9397894030341,37.9543320991532,22.6294657090004));
#35060=CARTESIAN_POINT('',(48.2294485608124,33.8328092275424,22.9294657090004));
#35061=CARTESIAN_POINT('Ctrl Pts',(47.8852591790204,33.8234449888007,22.6294657090004));
#35062=CARTESIAN_POINT('Ctrl Pts',(48.0605705931107,33.8282146244214,22.783158980636));
#35063=CARTESIAN_POINT('Ctrl Pts',(48.2294485608124,33.8328092275424,22.9294657090004));
#35064=CARTESIAN_POINT('',(48.0654635385539,33.5300503598268,22.6294657090004));
#35065=CARTESIAN_POINT('Ctrl Pts',(48.2294485608124,33.8328092275424,22.9294657090004));
#35066=CARTESIAN_POINT('Ctrl Pts',(48.1489886199846,33.6842593158128,22.783158980636));
#35067=CARTESIAN_POINT('Ctrl Pts',(48.0654635385539,33.5300503598268,22.6294657090004));
#35068=CARTESIAN_POINT('',(48.2454381951617,33.2621804705657,22.6294657090004));
#35069=CARTESIAN_POINT('Origin',(54.9397894030341,37.9543320991532,22.6294657090004));
#35070=CARTESIAN_POINT('',(48.5877190427886,33.2995681804899,22.9294657090004));
#35071=CARTESIAN_POINT('Ctrl Pts',(48.2454381951617,33.2621804705657,22.6294657090004));
#35072=CARTESIAN_POINT('Ctrl Pts',(48.4197775054016,33.2812237433775,22.783158980636));
#35073=CARTESIAN_POINT('Ctrl Pts',(48.5877190427886,33.2995681804899,22.9294657090004));
#35074=CARTESIAN_POINT('',(48.4489573255588,32.984450416254,22.6294657090004));
#35075=CARTESIAN_POINT('Ctrl Pts',(48.5877190427886,33.2995681804899,22.9294657090004));
#35076=CARTESIAN_POINT('Ctrl Pts',(48.5196350226525,33.1449543242059,22.783158980636));
#35077=CARTESIAN_POINT('Ctrl Pts',(48.4489573255588,32.984450416254,22.6294657090004));
#35078=CARTESIAN_POINT('',(48.6501670141011,32.7321414472684,22.6294657090004));
#35079=CARTESIAN_POINT('Origin',(54.9397894030341,37.9543320991532,22.6294657090004));
#35080=CARTESIAN_POINT('',(48.9882615049944,32.7973038193341,22.9294657090004));
#35081=CARTESIAN_POINT('Ctrl Pts',(48.6501670141012,32.7321414472685,22.6294657090004));
#35082=CARTESIAN_POINT('Ctrl Pts',(48.8223740211449,32.7653316274327,22.783158980636));
#35083=CARTESIAN_POINT('Ctrl Pts',(48.9882615049944,32.7973038193341,22.9294657090004));
#35084=CARTESIAN_POINT('',(48.8756465291274,32.4719242153081,22.6294657090004));
#35085=CARTESIAN_POINT('Ctrl Pts',(48.9882615049944,32.7973038193341,22.9294657090004));
#35086=CARTESIAN_POINT('Ctrl Pts',(48.9330064934709,32.6376549481999,22.7831589806361));
#35087=CARTESIAN_POINT('Ctrl Pts',(48.8756465291274,32.4719242153081,22.6294657090004));
#35088=CARTESIAN_POINT('',(49.0967522323243,32.2368552411587,22.6294657090004));
#35089=CARTESIAN_POINT('Origin',(54.9397894030341,37.9543320991532,22.6294657090004));
#35090=CARTESIAN_POINT('',(49.4284104034286,32.3293586305307,22.9294657090004));
#35091=CARTESIAN_POINT('Ctrl Pts',(49.0967522323243,32.2368552411587,22.6294657090004));
#35092=CARTESIAN_POINT('Ctrl Pts',(49.2656809269522,32.2839714535024,22.783158980636));
#35093=CARTESIAN_POINT('Ctrl Pts',(49.4284104034286,32.3293586305307,22.9294657090004));
#35094=CARTESIAN_POINT('',(49.3426916030088,31.9958825342957,22.6294657090004));
#35095=CARTESIAN_POINT('Ctrl Pts',(49.4284104034286,32.3293586305307,22.9294657090004));
#35096=CARTESIAN_POINT('Ctrl Pts',(49.386352113503,32.1657371814434,22.7831589806361));
#35097=CARTESIAN_POINT('Ctrl Pts',(49.3426916030088,31.9958825342957,22.6294657090004));
#35098=CARTESIAN_POINT('',(49.5822218988852,31.7796179002216,22.6294657090004));
#35099=CARTESIAN_POINT('Origin',(54.9397894030341,37.9543320991532,22.6294657090004));
#35100=CARTESIAN_POINT('',(49.9052366197917,31.8988467121057,22.9294657090004));
#35101=CARTESIAN_POINT('Ctrl Pts',(49.5822218988853,31.7796179002216,22.6294657090004));
#35102=CARTESIAN_POINT('Ctrl Pts',(49.7467480885058,31.8403465941252,22.7831589806361));
#35103=CARTESIAN_POINT('Ctrl Pts',(49.9052366197917,31.8988467121057,22.9294657090004));
#35104=CARTESIAN_POINT('',(49.8469844392931,31.5594933520623,22.6294657090004));
#35105=CARTESIAN_POINT('Ctrl Pts',(49.9052366197917,31.8988467121057,22.9294657090004));
#35106=CARTESIAN_POINT('Ctrl Pts',(49.8766549424443,31.7323415588134,22.783158980636));
#35107=CARTESIAN_POINT('Ctrl Pts',(49.8469844392932,31.5594933520623,22.6294657090004));
#35108=CARTESIAN_POINT('',(50.1033452932499,31.3634722635223,22.6294657090004));
#35109=CARTESIAN_POINT('Origin',(54.9397894030341,37.9543320991532,22.6294657090004));
#35110=CARTESIAN_POINT('',(50.4155669542845,31.5086330498468,22.9294657090004));
#35111=CARTESIAN_POINT('Ctrl Pts',(50.1033452932499,31.3634722635223,22.6294657090004));
#35112=CARTESIAN_POINT('Ctrl Pts',(50.2623740832161,31.4374092995474,22.783158980636));
#35113=CARTESIAN_POINT('Ctrl Pts',(50.4155669542845,31.5086330498468,22.9294657090004));
#35114=CARTESIAN_POINT('',(50.3851690523575,31.1656607666167,22.6294657090004));
#35115=CARTESIAN_POINT('Ctrl Pts',(50.4155669542845,31.5086330498468,22.9294657090004));
#35116=CARTESIAN_POINT('Ctrl Pts',(50.4006520958624,31.3403522566732,22.7831589806361));
#35117=CARTESIAN_POINT('Ctrl Pts',(50.3851690523575,31.1656607666167,22.6294657090004));
#35118=CARTESIAN_POINT('',(50.656654425208,30.9911877116138,22.6294657090004));
#35119=CARTESIAN_POINT('Origin',(54.9397894030341,37.9543320991532,22.6294657090004));
#35120=CARTESIAN_POINT('',(50.9560052427296,31.1613144512955,22.9294657090004));
#35121=CARTESIAN_POINT('Ctrl Pts',(50.656654425208,30.9911877116138,22.6294657090004));
#35122=CARTESIAN_POINT('Ctrl Pts',(50.8091275051606,31.0778410509844,22.783158980636));
#35123=CARTESIAN_POINT('Ctrl Pts',(50.9560052427296,31.1613144512955,22.9294657090004));
#35124=CARTESIAN_POINT('',(50.9536639123962,30.8170056688373,22.6294657090004));
#35125=CARTESIAN_POINT('Ctrl Pts',(50.9560052427296,31.1613144512955,22.9294657090004));
#35126=CARTESIAN_POINT('Ctrl Pts',(50.9548564591548,30.9923778991548,22.783158980636));
#35127=CARTESIAN_POINT('Ctrl Pts',(50.9536639123962,30.8170056688373,22.6294657090004));
#35128=CARTESIAN_POINT('',(51.2384671137761,30.6652417367663,22.6294657090004));
#35129=CARTESIAN_POINT('Origin',(54.9397894030341,37.9543320991532,22.6294657090004));
#35130=CARTESIAN_POINT('',(51.5229549574834,30.8592022644217,22.9294657090004));
#35131=CARTESIAN_POINT('Ctrl Pts',(51.2384671137761,30.6652417367663,22.6294657090004));
#35132=CARTESIAN_POINT('Ctrl Pts',(51.3833698005242,30.7640347158057,22.783158980636));
#35133=CARTESIAN_POINT('Ctrl Pts',(51.5229549574834,30.8592022644216,22.9294657090004));
#35134=CARTESIAN_POINT('',(51.5486857799107,30.5158483008756,22.6294657090004));
#35135=CARTESIAN_POINT('Ctrl Pts',(51.5229549574834,30.8592022644217,22.9294657090004));
#35136=CARTESIAN_POINT('Ctrl Pts',(51.5355798937211,30.6907341981958,22.783158980636));
#35137=CARTESIAN_POINT('Ctrl Pts',(51.5486857799107,30.5158483008756,22.6294657090004));
#35138=CARTESIAN_POINT('',(51.844911491504,30.3878034556653,22.6294657090004));
#35139=CARTESIAN_POINT('Origin',(54.9397894030341,37.9543320991532,22.6294657090004));
#35140=CARTESIAN_POINT('',(52.1126431417343,30.6043069959839,22.9294657090004));
#35141=CARTESIAN_POINT('Ctrl Pts',(51.8449114915039,30.3878034556653,22.6294657090004));
#35142=CARTESIAN_POINT('Ctrl Pts',(51.9812794815746,30.4980786233977,22.7831589806361));
#35143=CARTESIAN_POINT('Ctrl Pts',(52.1126431417343,30.6043069959839,22.9294657090004));
#35144=CARTESIAN_POINT('',(52.1662748825443,30.264192815328,22.6294657090004));
#35145=CARTESIAN_POINT('Ctrl Pts',(52.1126431417343,30.6043069959839,22.9294657090004));
#35146=CARTESIAN_POINT('Ctrl Pts',(52.1389577809168,30.4374285428584,22.783158980636));
#35147=CARTESIAN_POINT('Ctrl Pts',(52.1662748825443,30.264192815328,22.6294657090004));
#35148=CARTESIAN_POINT('',(52.4719517711141,30.1607191742974,22.6294657090004));
#35149=CARTESIAN_POINT('Origin',(54.9397894030341,37.9543320991532,22.6294657090004));
#35150=CARTESIAN_POINT('',(52.7211455179079,30.398324931939,22.9294657090004));
#35151=CARTESIAN_POINT('Ctrl Pts',(52.4719517711141,30.1607191742974,22.6294657090004));
#35152=CARTESIAN_POINT('Ctrl Pts',(52.5988775580325,30.2817426676756,22.7831589806361));
#35153=CARTESIAN_POINT('Ctrl Pts',(52.7211455179079,30.398324931939,22.9294657090004));
#35154=CARTESIAN_POINT('',(52.8023212667141,30.0637139379306,22.6294657090004));
#35155=CARTESIAN_POINT('Ctrl Pts',(52.7211455179079,30.398324931939,22.9294657090004));
#35156=CARTESIAN_POINT('Ctrl Pts',(52.760974740453,30.2341466404863,22.783158980636));
#35157=CARTESIAN_POINT('Ctrl Pts',(52.8023212667141,30.0637139379306,22.6294657090004));
#35158=CARTESIAN_POINT('',(53.1154151030002,29.9855001010888,22.6294657090004));
#35159=CARTESIAN_POINT('Origin',(54.9397894030341,37.9543320991532,22.6294657090004));
#35160=CARTESIAN_POINT('',(53.3444126030865,30.2426268489385,22.9294657090004));
#35161=CARTESIAN_POINT('Ctrl Pts',(53.1154151030002,29.9855001010888,22.6294657090004));
#35162=CARTESIAN_POINT('Ctrl Pts',(53.2320540165956,30.1164665287319,22.783158980636));
#35163=CARTESIAN_POINT('Ctrl Pts',(53.3444126030865,30.2426268489385,22.9294657090004));
#35164=CARTESIAN_POINT('',(53.4525921486737,29.9157458225357,22.6294657090004));
#35165=CARTESIAN_POINT('Ctrl Pts',(53.3444126030866,30.2426268489385,22.9294657090004));
#35166=CARTESIAN_POINT('Ctrl Pts',(53.3974913520896,30.0822412986007,22.7831589806361));
#35167=CARTESIAN_POINT('Ctrl Pts',(53.4525921486737,29.9157458225357,22.6294657090004));
#35168=CARTESIAN_POINT('',(53.7710193448524,29.8633122900625,22.6294657090004));
#35169=CARTESIAN_POINT('Origin',(54.9397894030341,37.9543320991532,22.6294657090004));
#35170=CARTESIAN_POINT('',(53.9782966576502,30.1382488920364,22.9294657090004));
#35171=CARTESIAN_POINT('Ctrl Pts',(53.7710193448524,29.8633122900625,22.6294657090004));
#35172=CARTESIAN_POINT('Ctrl Pts',(53.876595172399,30.0033500920025,22.783158980636));
#35173=CARTESIAN_POINT('Ctrl Pts',(53.9782966576502,30.1382488920364,22.9294657090004));
#35174=CARTESIAN_POINT('',(54.1127600829908,29.8212731725384,22.6294657090004));
#35175=CARTESIAN_POINT('Ctrl Pts',(53.9782966576502,30.1382488920364,22.9294657090004));
#35176=CARTESIAN_POINT('Ctrl Pts',(54.044271702794,29.9827234221892,22.7831589806361));
#35177=CARTESIAN_POINT('Ctrl Pts',(54.1127600829908,29.8212731725384,22.6294657090004));
#35178=CARTESIAN_POINT('',(54.4344015586084,29.7949688809415,22.6294657090004));
#35179=CARTESIAN_POINT('Origin',(54.9397894030341,37.9543320991532,22.6294657090004));
#35180=CARTESIAN_POINT('',(54.6185792877992,30.0858856793146,22.9294657090004));
#35181=CARTESIAN_POINT('Ctrl Pts',(54.4344015586084,29.7949688809415,22.6294657090004));
#35182=CARTESIAN_POINT('Ctrl Pts',(54.5282117103925,29.943146128711,22.783158980636));
#35183=CARTESIAN_POINT('Ctrl Pts',(54.6185792877992,30.0858856793146,22.9294657090004));
#35184=CARTESIAN_POINT('',(54.7784317609826,29.7809246878375,22.6294657090004));
#35185=CARTESIAN_POINT('Ctrl Pts',(54.6185792877992,30.0858856793146,22.9294657090004));
#35186=CARTESIAN_POINT('Ctrl Pts',(54.6970115760434,29.9362552863001,22.783158980636));
#35187=CARTESIAN_POINT('Ctrl Pts',(54.7784317609826,29.7809246878375,22.6294657090004));
#35188=CARTESIAN_POINT('',(55.1011470450858,29.7809246878375,22.6294657090004));
#35189=CARTESIAN_POINT('Origin',(54.9397894030341,37.9543320991532,22.6294657090004));
#35190=CARTESIAN_POINT('',(55.2609995182692,30.0858856793146,22.9294657090004));
#35191=CARTESIAN_POINT('Ctrl Pts',(55.1011470450858,29.7809246878374,22.6294657090004));
#35192=CARTESIAN_POINT('Ctrl Pts',(55.182567230025,29.9362552863001,22.783158980636));
#35193=CARTESIAN_POINT('Ctrl Pts',(55.2609995182692,30.0858856793146,22.9294657090004));
#35194=CARTESIAN_POINT('',(55.44517724746,29.7949688809415,22.6294657090004));
#35195=CARTESIAN_POINT('Ctrl Pts',(55.2609995182692,30.0858856793146,22.9294657090003));
#35196=CARTESIAN_POINT('Ctrl Pts',(55.3513670956759,29.943146128711,22.783158980636));
#35197=CARTESIAN_POINT('Ctrl Pts',(55.44517724746,29.7949688809415,22.6294657090004));
#35198=CARTESIAN_POINT('',(55.7668187230776,29.8212731725384,22.6294657090004));
#35199=CARTESIAN_POINT('Origin',(54.9397894030341,37.9543320991532,22.6294657090004));
#35200=CARTESIAN_POINT('',(55.9012821484182,30.1382488920364,22.9294657090004));
#35201=CARTESIAN_POINT('Ctrl Pts',(55.7668187230776,29.8212731725384,22.6294657090004));
#35202=CARTESIAN_POINT('Ctrl Pts',(55.8353071032744,29.9827234221893,22.783158980636));
#35203=CARTESIAN_POINT('Ctrl Pts',(55.9012821484182,30.1382488920364,22.9294657090004));
#35204=CARTESIAN_POINT('',(56.108559461216,29.8633122900625,22.6294657090004));
#35205=CARTESIAN_POINT('Ctrl Pts',(55.9012821484182,30.1382488920364,22.9294657090004));
#35206=CARTESIAN_POINT('Ctrl Pts',(56.0029836336695,30.0033500920025,22.7831589806361));
#35207=CARTESIAN_POINT('Ctrl Pts',(56.108559461216,29.8633122900626,22.6294657090004));
#35208=CARTESIAN_POINT('',(56.4269866573947,29.9157458225358,22.6294657090004));
#35209=CARTESIAN_POINT('Origin',(54.9397894030341,37.9543320991532,22.6294657090004));
#35210=CARTESIAN_POINT('',(56.5351662029818,30.2426268489385,22.9294657090004));
#35211=CARTESIAN_POINT('Ctrl Pts',(56.4269866573947,29.9157458225358,22.6294657090004));
#35212=CARTESIAN_POINT('Ctrl Pts',(56.4820874539788,30.0822412986007,22.783158980636));
#35213=CARTESIAN_POINT('Ctrl Pts',(56.5351662029818,30.2426268489385,22.9294657090004));
#35214=CARTESIAN_POINT('',(56.7641637030682,29.9855001010888,22.6294657090004));
#35215=CARTESIAN_POINT('Ctrl Pts',(56.5351662029818,30.2426268489385,22.9294657090004));
#35216=CARTESIAN_POINT('Ctrl Pts',(56.6475247894728,30.1164665287319,22.783158980636));
#35217=CARTESIAN_POINT('Ctrl Pts',(56.7641637030682,29.9855001010888,22.6294657090004));
#35218=CARTESIAN_POINT('',(57.0772575393543,30.0637139379306,22.6294657090004));
#35219=CARTESIAN_POINT('Origin',(54.9397894030341,37.9543320991532,22.6294657090004));
#35220=CARTESIAN_POINT('',(57.1584332881605,30.3983249319391,22.9294657090004));
#35221=CARTESIAN_POINT('Ctrl Pts',(57.0772575393543,30.0637139379306,22.6294657090004));
#35222=CARTESIAN_POINT('Ctrl Pts',(57.1186040656154,30.2341466404863,22.783158980636));
#35223=CARTESIAN_POINT('Ctrl Pts',(57.1584332881605,30.3983249319391,22.9294657090004));
#35224=CARTESIAN_POINT('',(57.4076270349543,30.1607191742974,22.6294657090004));
#35225=CARTESIAN_POINT('Ctrl Pts',(57.1584332881605,30.3983249319391,22.9294657090004));
#35226=CARTESIAN_POINT('Ctrl Pts',(57.2807012480359,30.2817426676757,22.783158980636));
#35227=CARTESIAN_POINT('Ctrl Pts',(57.4076270349542,30.1607191742974,22.6294657090004));
#35228=CARTESIAN_POINT('',(57.7133039235241,30.264192815328,22.6294657090004));
#35229=CARTESIAN_POINT('Origin',(54.9397894030341,37.9543320991532,22.6294657090004));
#35230=CARTESIAN_POINT('',(57.766935664334,30.604306995984,22.9294657090004));
#35231=CARTESIAN_POINT('Ctrl Pts',(57.7133039235241,30.264192815328,22.6294657090004));
#35232=CARTESIAN_POINT('Ctrl Pts',(57.7406210251516,30.4374285428584,22.783158980636));
#35233=CARTESIAN_POINT('Ctrl Pts',(57.766935664334,30.604306995984,22.9294657090003));
#35234=CARTESIAN_POINT('',(58.0346673145644,30.3878034556654,22.6294657090004));
#35235=CARTESIAN_POINT('Ctrl Pts',(57.766935664334,30.604306995984,22.9294657090004));
#35236=CARTESIAN_POINT('Ctrl Pts',(57.8982993244938,30.4980786233977,22.783158980636));
#35237=CARTESIAN_POINT('Ctrl Pts',(58.0346673145644,30.3878034556654,22.6294657090004));
#35238=CARTESIAN_POINT('',(58.3308930261577,30.5158483008756,22.6294657090004));
#35239=CARTESIAN_POINT('Origin',(54.9397894030341,37.9543320991532,22.6294657090004));
#35240=CARTESIAN_POINT('',(58.356623848585,30.8592022644217,22.9294657090004));
#35241=CARTESIAN_POINT('Ctrl Pts',(58.3308930261577,30.5158483008756,22.6294657090004));
#35242=CARTESIAN_POINT('Ctrl Pts',(58.3439989123473,30.6907341981958,22.783158980636));
#35243=CARTESIAN_POINT('Ctrl Pts',(58.356623848585,30.8592022644217,22.9294657090004));
#35244=CARTESIAN_POINT('',(58.6411116922923,30.6652417367664,22.6294657090004));
#35245=CARTESIAN_POINT('Ctrl Pts',(58.356623848585,30.8592022644217,22.9294657090004));
#35246=CARTESIAN_POINT('Ctrl Pts',(58.4962090055442,30.7640347158058,22.783158980636));
#35247=CARTESIAN_POINT('Ctrl Pts',(58.6411116922923,30.6652417367664,22.6294657090004));
#35248=CARTESIAN_POINT('',(58.9259148936722,30.8170056688373,22.6294657090004));
#35249=CARTESIAN_POINT('Origin',(54.9397894030341,37.9543320991532,22.6294657090004));
#35250=CARTESIAN_POINT('',(58.9235735633387,31.1613144512955,22.9294657090004));
#35251=CARTESIAN_POINT('Ctrl Pts',(58.9259148936722,30.8170056688373,22.6294657090004));
#35252=CARTESIAN_POINT('Ctrl Pts',(58.9247223469135,30.9923778991548,22.783158980636));
#35253=CARTESIAN_POINT('Ctrl Pts',(58.9235735633387,31.1613144512955,22.9294657090004));
#35254=CARTESIAN_POINT('',(59.2229243808604,30.9911877116138,22.6294657090004));
#35255=CARTESIAN_POINT('Ctrl Pts',(58.9235735633387,31.1613144512955,22.9294657090004));
#35256=CARTESIAN_POINT('Ctrl Pts',(59.0704513009078,31.0778410509844,22.783158980636));
#35257=CARTESIAN_POINT('Ctrl Pts',(59.2229243808603,30.9911877116138,22.6294657090004));
#35258=CARTESIAN_POINT('',(59.4944097537108,31.1656607666168,22.6294657090004));
#35259=CARTESIAN_POINT('Origin',(54.9397894030341,37.9543320991532,22.6294657090004));
#35260=CARTESIAN_POINT('',(59.4640118517838,31.5086330498468,22.9294657090004));
#35261=CARTESIAN_POINT('Ctrl Pts',(59.4944097537109,31.1656607666168,22.6294657090004));
#35262=CARTESIAN_POINT('Ctrl Pts',(59.478926710206,31.3403522566732,22.783158980636));
#35263=CARTESIAN_POINT('Ctrl Pts',(59.4640118517838,31.5086330498468,22.9294657090004));
#35264=CARTESIAN_POINT('',(59.7762335128185,31.3634722635224,22.6294657090004));
#35265=CARTESIAN_POINT('Ctrl Pts',(59.4640118517839,31.5086330498468,22.9294657090004));
#35266=CARTESIAN_POINT('Ctrl Pts',(59.6172047228522,31.4374092995474,22.783158980636));
#35267=CARTESIAN_POINT('Ctrl Pts',(59.7762335128185,31.3634722635223,22.6294657090004));
#35268=CARTESIAN_POINT('',(60.0325943667752,31.5594933520624,22.6294657090004));
#35269=CARTESIAN_POINT('Origin',(54.9397894030341,37.9543320991532,22.6294657090004));
#35270=CARTESIAN_POINT('',(59.9743421862767,31.8988467121058,22.9294657090004));
#35271=CARTESIAN_POINT('Ctrl Pts',(60.0325943667752,31.5594933520624,22.6294657090004));
#35272=CARTESIAN_POINT('Ctrl Pts',(60.0029238636241,31.7323415588135,22.783158980636));
#35273=CARTESIAN_POINT('Ctrl Pts',(59.9743421862767,31.8988467121058,22.9294657090004));
#35274=CARTESIAN_POINT('',(60.2973569071831,31.7796179002217,22.6294657090004));
#35275=CARTESIAN_POINT('Ctrl Pts',(59.9743421862767,31.8988467121058,22.9294657090004));
#35276=CARTESIAN_POINT('Ctrl Pts',(60.1328307175625,31.8403465941253,22.783158980636));
#35277=CARTESIAN_POINT('Ctrl Pts',(60.2973569071831,31.7796179002217,22.6294657090004));
#35278=CARTESIAN_POINT('',(60.5368872030596,31.9958825342957,22.6294657090004));
#35279=CARTESIAN_POINT('Origin',(54.9397894030341,37.9543320991532,22.6294657090004));
#35280=CARTESIAN_POINT('',(60.4511684026397,32.3293586305308,22.9294657090004));
#35281=CARTESIAN_POINT('Ctrl Pts',(60.5368872030596,31.9958825342957,22.6294657090004));
#35282=CARTESIAN_POINT('Ctrl Pts',(60.4932266925653,32.1657371814435,22.7831589806361));
#35283=CARTESIAN_POINT('Ctrl Pts',(60.4511684026397,32.3293586305308,22.9294657090004));
#35284=CARTESIAN_POINT('',(60.7828265737441,32.2368552411588,22.6294657090004));
#35285=CARTESIAN_POINT('Ctrl Pts',(60.4511684026397,32.3293586305308,22.9294657090004));
#35286=CARTESIAN_POINT('Ctrl Pts',(60.6138978791162,32.2839714535025,22.783158980636));
#35287=CARTESIAN_POINT('Ctrl Pts',(60.7828265737441,32.2368552411588,22.6294657090004));
#35288=CARTESIAN_POINT('',(61.0039322769409,32.4719242153082,22.6294657090004));
#35289=CARTESIAN_POINT('Origin',(54.9397894030341,37.9543320991532,22.6294657090004));
#35290=CARTESIAN_POINT('',(60.891317301074,32.7973038193341,22.9294657090004));
#35291=CARTESIAN_POINT('Ctrl Pts',(61.0039322769409,32.4719242153082,22.6294657090004));
#35292=CARTESIAN_POINT('Ctrl Pts',(60.9465723125975,32.6376549481999,22.783158980636));
#35293=CARTESIAN_POINT('Ctrl Pts',(60.891317301074,32.7973038193341,22.9294657090004));
#35294=CARTESIAN_POINT('',(61.2294117919672,32.7321414472685,22.6294657090004));
#35295=CARTESIAN_POINT('Ctrl Pts',(60.891317301074,32.7973038193341,22.9294657090004));
#35296=CARTESIAN_POINT('Ctrl Pts',(61.0572047849235,32.7653316274328,22.783158980636));
#35297=CARTESIAN_POINT('Ctrl Pts',(61.2294117919672,32.7321414472685,22.6294657090004));
#35298=CARTESIAN_POINT('',(61.4306214805095,32.9844504162541,22.6294657090004));
#35299=CARTESIAN_POINT('Origin',(54.9397894030341,37.9543320991532,22.6294657090004));
#35300=CARTESIAN_POINT('',(61.2918597632797,33.2995681804899,22.9294657090004));
#35301=CARTESIAN_POINT('Ctrl Pts',(61.4306214805095,32.9844504162541,22.6294657090004));
#35302=CARTESIAN_POINT('Ctrl Pts',(61.3599437834158,33.144954324206,22.783158980636));
#35303=CARTESIAN_POINT('Ctrl Pts',(61.2918597632797,33.2995681804899,22.9294657090004));
#35304=CARTESIAN_POINT('',(61.6341406109067,33.2621804705658,22.6294657090004));
#35305=CARTESIAN_POINT('Ctrl Pts',(61.2918597632797,33.2995681804899,22.9294657090004));
#35306=CARTESIAN_POINT('Ctrl Pts',(61.4598013006668,33.2812237433776,22.783158980636));
#35307=CARTESIAN_POINT('Ctrl Pts',(61.6341406109067,33.2621804705658,22.6294657090004));
#35308=CARTESIAN_POINT('',(61.8141152675145,33.5300503598269,22.6294657090004));
#35309=CARTESIAN_POINT('Origin',(54.9397894030341,37.9543320991532,22.6294657090004));
#35310=CARTESIAN_POINT('',(61.6501302452559,33.8328092275425,22.9294657090004));
#35311=CARTESIAN_POINT('Ctrl Pts',(61.8141152675145,33.5300503598269,22.6294657090004));
#35312=CARTESIAN_POINT('Ctrl Pts',(61.7305901860837,33.6842593158128,22.783158980636));
#35313=CARTESIAN_POINT('Ctrl Pts',(61.6501302452559,33.8328092275425,22.9294657090004));
#35314=CARTESIAN_POINT('',(61.9943196270479,33.8234449888007,22.6294657090004));
#35315=CARTESIAN_POINT('Ctrl Pts',(61.6501302452559,33.8328092275425,22.9294657090004));
#35316=CARTESIAN_POINT('Ctrl Pts',(61.8190082129576,33.8282146244215,22.783158980636));
#35317=CARTESIAN_POINT('Ctrl Pts',(61.9943196270479,33.8234449888007,22.6294657090004));
#35318=CARTESIAN_POINT('',(62.1518615500752,34.1050931684198,22.6294657090004));
#35319=CARTESIAN_POINT('Origin',(54.9397894030341,37.9543320991532,22.6294657090004));
#35320=CARTESIAN_POINT('',(61.9637445160554,34.3934783293021,22.9294657090004));
#35321=CARTESIAN_POINT('Ctrl Pts',(62.1518615500752,34.1050931684198,22.6294657090004));
#35322=CARTESIAN_POINT('Ctrl Pts',(62.0560449299436,34.2519809372804,22.783158980636));
#35323=CARTESIAN_POINT('Ctrl Pts',(61.9637445160554,34.3934783293021,22.9294657090004));
#35324=CARTESIAN_POINT('',(62.3075519084639,34.4121998792067,22.6294657090004));
#35325=CARTESIAN_POINT('Ctrl Pts',(61.9637445160554,34.3934783293021,22.9294657090004));
#35326=CARTESIAN_POINT('Ctrl Pts',(62.1324350590596,34.4026641364983,22.783158980636));
#35327=CARTESIAN_POINT('Ctrl Pts',(62.3075519084639,34.4121998792067,22.6294657090004));
#35328=CARTESIAN_POINT('',(62.4416126824056,34.705752027017,22.6294657090004));
#35329=CARTESIAN_POINT('Origin',(54.9397894030341,37.9543320991532,22.6294657090004));
#35330=CARTESIAN_POINT('',(62.2306155244487,34.9778443254007,22.9294657090004));
#35331=CARTESIAN_POINT('Ctrl Pts',(62.4416126824056,34.705752027017,22.6294657090004));
#35332=CARTESIAN_POINT('Ctrl Pts',(62.3341421673715,34.8443410948853,22.783158980636));
#35333=CARTESIAN_POINT('Ctrl Pts',(62.2306155244488,34.9778443254007,22.9294657090004));
#35334=CARTESIAN_POINT('',(62.5717529460015,35.0245270751257,22.6294657090004));
#35335=CARTESIAN_POINT('Ctrl Pts',(62.2306155244487,34.9778443254006,22.9294657090003));
#35336=CARTESIAN_POINT('Ctrl Pts',(62.3979960350237,35.0007494128826,22.783158980636));
#35337=CARTESIAN_POINT('Ctrl Pts',(62.5717529460015,35.0245270751257,22.6294657090004));
#35338=CARTESIAN_POINT('',(62.6814404185254,35.3280296500162,22.6294657090004));
#35339=CARTESIAN_POINT('Origin',(54.9397894030341,37.9543320991532,22.6294657090004));
#35340=CARTESIAN_POINT('',(62.4489672879057,35.5820183565476,22.9294657090004));
#35341=CARTESIAN_POINT('Ctrl Pts',(62.6814404185254,35.3280296500163,22.6294657090004));
#35342=CARTESIAN_POINT('Ctrl Pts',(62.563031207135,35.4573977295112,22.783158980636));
#35343=CARTESIAN_POINT('Ctrl Pts',(62.4489672879057,35.5820183565476,22.9294657090003));
#35344=CARTESIAN_POINT('',(62.785164525346,35.6563516400959,22.6294657090004));
#35345=CARTESIAN_POINT('Ctrl Pts',(62.4489672879057,35.5820183565476,22.9294657090004));
#35346=CARTESIAN_POINT('Ctrl Pts',(62.6139238763694,35.6184902947372,22.783158980636));
#35347=CARTESIAN_POINT('Ctrl Pts',(62.785164525346,35.6563516400959,22.6294657090004));
#35348=CARTESIAN_POINT('',(62.8697487444197,35.9677848825051,22.6294657090004));
#35349=CARTESIAN_POINT('Origin',(54.9397894030341,37.9543320991532,22.6294657090004));
#35350=CARTESIAN_POINT('',(62.617346711466,36.2019797442473,22.9294657090004));
#35351=CARTESIAN_POINT('Ctrl Pts',(62.8697487444197,35.9677848825051,22.6294657090004));
#35352=CARTESIAN_POINT('Ctrl Pts',(62.7411888304386,36.0870710504019,22.783158980636));
#35353=CARTESIAN_POINT('Ctrl Pts',(62.617346711466,36.2019797442473,22.9294657090004));
#35354=CARTESIAN_POINT('',(62.9463664276474,36.3034688858809,22.6294657090003));
#35355=CARTESIAN_POINT('Ctrl Pts',(62.617346711466,36.2019797442473,22.9294657090004));
#35356=CARTESIAN_POINT('Ctrl Pts',(62.7787816189382,36.2517758184133,22.783158980636));
#35357=CARTESIAN_POINT('Ctrl Pts',(62.9463664276474,36.3034688858809,22.6294657090004));
#35358=CARTESIAN_POINT('',(63.0052844992482,36.6207602589636,22.6294657090003));
#35359=CARTESIAN_POINT('Origin',(54.9397894030341,37.9543320991532,22.6294657090004));
#35360=CARTESIAN_POINT('',(62.7346332578465,36.8336027477512,22.9294657090004));
#35361=CARTESIAN_POINT('Ctrl Pts',(63.0052844992482,36.6207602589636,22.6294657090004));
#35362=CARTESIAN_POINT('Ctrl Pts',(62.8674294276931,36.7291706854956,22.783158980636));
#35363=CARTESIAN_POINT('Ctrl Pts',(62.7346332578465,36.8336027477512,22.9294657090004));
#35364=CARTESIAN_POINT('',(63.0542858808421,36.9615723539771,22.6294657090003));
#35365=CARTESIAN_POINT('Ctrl Pts',(62.7346332578465,36.8336027477512,22.9294657090004));
#35366=CARTESIAN_POINT('Ctrl Pts',(62.8914721616528,36.8963915732358,22.783158980636));
#35367=CARTESIAN_POINT('Ctrl Pts',(63.0542858808421,36.9615723539771,22.6294657090004));
#35368=CARTESIAN_POINT('',(63.0871457149245,37.2826103359947,22.6294657090003));
#35369=CARTESIAN_POINT('Origin',(54.9397894030341,37.9543320991532,22.6294657090004));
#35370=CARTESIAN_POINT('',(62.8000464044319,37.4726840201813,22.9294657090004));
#35371=CARTESIAN_POINT('Ctrl Pts',(63.0871457149245,37.2826103359947,22.6294657090004));
#35372=CARTESIAN_POINT('Ctrl Pts',(62.9409128885521,37.3794235676598,22.783158980636));
#35373=CARTESIAN_POINT('Ctrl Pts',(62.8000464044319,37.4726840201813,22.9294657090004));
#35374=CARTESIAN_POINT('',(63.1082046987747,37.6262824743835,22.6294657090003));
#35375=CARTESIAN_POINT('Ctrl Pts',(62.8000464044319,37.4726840201813,22.9294657090004));
#35376=CARTESIAN_POINT('Ctrl Pts',(62.951245567544,37.5480477477104,22.783158980636));
#35377=CARTESIAN_POINT('Ctrl Pts',(63.1082046987747,37.6262824743835,22.6294657090004));
#35378=CARTESIAN_POINT('',(63.1147876185643,37.9489306105332,22.6294657090003));
#35379=CARTESIAN_POINT('Origin',(54.9397894030341,37.9543320991532,22.6294657090004));
#35380=CARTESIAN_POINT('',(63.1049749955285,37.9543320991532,22.639280116506));
#35381=CARTESIAN_POINT('Ctrl Pts',(63.1147876185642,37.9489306105333,22.6294657090004));
#35382=CARTESIAN_POINT('Ctrl Pts',(63.1098783601679,37.9516329769916,22.6343767518666));
#35383=CARTESIAN_POINT('Ctrl Pts',(63.1049749955285,37.9543320991532,22.639280116506));
#35384=CARTESIAN_POINT('',(62.7147894030341,37.9543320991532,23.0294657090004));
#35385=CARTESIAN_POINT('',(63.1147894030342,37.9543320991532,22.6294657090004));
#35386=CARTESIAN_POINT('Origin',(54.9397894030341,37.9543320991532,23.0294657090004));
#35387=CARTESIAN_POINT('',(62.8131508375241,38.1149705811106,22.9294657090004));
#35388=CARTESIAN_POINT('Ctrl Pts',(63.1049749955285,37.9543320991532,22.639280116506));
#35389=CARTESIAN_POINT('Ctrl Pts',(62.9564231974998,38.0361044085143,22.7878319145347));
#35390=CARTESIAN_POINT('Ctrl Pts',(62.8131508375241,38.1149705811106,22.9294657090004));
#35391=CARTESIAN_POINT('',(63.1077640606078,38.2931757109184,22.6294657090003));
#35392=CARTESIAN_POINT('Ctrl Pts',(62.8131508375241,38.1149705811106,22.9294657090004));
#35393=CARTESIAN_POINT('Ctrl Pts',(62.9577040544577,38.2024076775117,22.783158980636));
#35394=CARTESIAN_POINT('Ctrl Pts',(63.1077640606078,38.2931757109184,22.6294657090004));
#35395=CARTESIAN_POINT('',(63.0880262578595,38.6152868310874,22.6294657090003));
#35396=CARTESIAN_POINT('Origin',(54.9397894030341,37.9543320991532,22.6294657090004));
#35397=CARTESIAN_POINT('',(62.773859349283,38.756188119446,22.9294657090004));
#35398=CARTESIAN_POINT('Ctrl Pts',(63.0880262578595,38.6152868310874,22.6294657090004));
#35399=CARTESIAN_POINT('Ctrl Pts',(62.9280066642388,38.6870543097374,22.783158980636));
#35400=CARTESIAN_POINT('Ctrl Pts',(62.7738593492831,38.756188119446,22.9294657090004));
#35401=CARTESIAN_POINT('',(63.0529668987158,38.9578139991223,22.6294657090003));
#35402=CARTESIAN_POINT('Ctrl Pts',(62.7738593492831,38.756188119446,22.9294657090004));
#35403=CARTESIAN_POINT('Ctrl Pts',(62.910804642229,38.8551167052685,22.783158980636));
#35404=CARTESIAN_POINT('Ctrl Pts',(63.0529668987157,38.9578139991223,22.6294657090004));
#35405=CARTESIAN_POINT('',(63.0070397252503,39.2772445069504,22.6294657090003));
#35406=CARTESIAN_POINT('Origin',(54.9397894030341,37.9543320991532,22.6294657090004));
#35407=CARTESIAN_POINT('',(62.6824334180802,39.3920694382633,22.9294657090004));
#35408=CARTESIAN_POINT('Ctrl Pts',(63.0070397252503,39.2772445069504,22.6294657090004));
#35409=CARTESIAN_POINT('Ctrl Pts',(62.8417028678599,39.335730102806,22.7831589806361));
#35410=CARTESIAN_POINT('Ctrl Pts',(62.6824334180802,39.3920694382633,22.9294657090004));
#35411=CARTESIAN_POINT('',(62.94417787917,39.6157742808448,22.6294657090003));
#35412=CARTESIAN_POINT('Ctrl Pts',(62.6824334180802,39.3920694382633,22.9294657090004));
#35413=CARTESIAN_POINT('Ctrl Pts',(62.8108594387084,39.5018311600907,22.7831589806361));
#35414=CARTESIAN_POINT('Ctrl Pts',(62.94417787917,39.6157742808448,22.6294657090004));
#35415=CARTESIAN_POINT('',(62.8723669727493,39.9303984190047,22.6294657090004));
#35416=CARTESIAN_POINT('Origin',(54.9397894030341,37.9543320991532,22.6294657090004));
#35417=CARTESIAN_POINT('',(62.5394814684036,40.0183828522987,22.9294657090004));
#35418=CARTESIAN_POINT('Ctrl Pts',(62.8723669727493,39.9303984190047,22.6294657090004));
#35419=CARTESIAN_POINT('Ctrl Pts',(62.7028131410966,39.975212920075,22.783158980636));
#35420=CARTESIAN_POINT('Ctrl Pts',(62.5394814684036,40.0183828522987,22.9294657090004));
#35421=CARTESIAN_POINT('',(62.7821209749467,40.2626779389667,22.6294657090004));
#35422=CARTESIAN_POINT('Ctrl Pts',(62.5394814684036,40.0183828522987,22.9294657090004));
#35423=CARTESIAN_POINT('Ctrl Pts',(62.6585335627355,40.1382472639816,22.783158980636));
#35424=CARTESIAN_POINT('Ctrl Pts',(62.7821209749467,40.2626779389667,22.6294657090003));
#35425=CARTESIAN_POINT('',(62.6849042253051,40.5704019357284,22.6294657090004));
#35426=CARTESIAN_POINT('Origin',(54.9397894030341,37.9543320991532,22.6294657090004));
#35427=CARTESIAN_POINT('',(62.3459548218929,40.6309603491164,22.9294657090004));
#35428=CARTESIAN_POINT('Ctrl Pts',(62.6849042253051,40.5704019357284,22.6294657090004));
#35429=CARTESIAN_POINT('Ctrl Pts',(62.5122617721653,40.6012471089027,22.783158980636));
#35430=CARTESIAN_POINT('Ctrl Pts',(62.3459548218929,40.6309603491164,22.9294657090004));
#35431=CARTESIAN_POINT('',(62.5678746480059,40.894219936375,22.6294657090004));
#35432=CARTESIAN_POINT('Ctrl Pts',(62.3459548218929,40.6309603491164,22.9294657090004));
#35433=CARTESIAN_POINT('Ctrl Pts',(62.4548407178829,40.7601297727713,22.783158980636));
#35434=CARTESIAN_POINT('Ctrl Pts',(62.5678746480059,40.894219936375,22.6294657090004));
#35435=CARTESIAN_POINT('',(62.4458990165727,41.1929959393108,22.6294657090004));
#35436=CARTESIAN_POINT('Origin',(54.9397894030341,37.9543320991532,22.6294657090004));
#35437=CARTESIAN_POINT('',(62.1031413664509,41.2257253265432,22.9294657090004));
#35438=CARTESIAN_POINT('Ctrl Pts',(62.4458990165727,41.1929959393108,22.6294657090004));
#35439=CARTESIAN_POINT('Ctrl Pts',(62.2713168489873,41.2096665150507,22.783158980636));
#35440=CARTESIAN_POINT('Ctrl Pts',(62.1031413664509,41.2257253265432,22.9294657090004));
#35441=CARTESIAN_POINT('',(62.3028646723053,41.5061974652739,22.6294657090004));
#35442=CARTESIAN_POINT('Ctrl Pts',(62.1031413664509,41.2257253265432,22.9294657090004));
#35443=CARTESIAN_POINT('Ctrl Pts',(62.2011364464262,41.3633401609671,22.783158980636));
#35444=CARTESIAN_POINT('Ctrl Pts',(62.3028646723053,41.5061974652739,22.6294657090004));
#35445=CARTESIAN_POINT('',(62.1569418867831,41.7940371693789,22.6294657090004));
#35446=CARTESIAN_POINT('Origin',(54.9397894030341,37.9543320991532,22.6294657090004));
#35447=CARTESIAN_POINT('',(61.8126569855623,41.7987197217835,22.9294657090004));
#35448=CARTESIAN_POINT('Ctrl Pts',(62.156941886783,41.7940371693789,22.6294657090004));
#35449=CARTESIAN_POINT('Ctrl Pts',(61.9815818202734,41.7964222077532,22.783158980636));
#35450=CARTESIAN_POINT('Ctrl Pts',(61.8126569855623,41.7987197217835,22.9294657090004));
#35451=CARTESIAN_POINT('',(61.9888546455096,42.0945379161778,22.6294657090004));
#35452=CARTESIAN_POINT('Ctrl Pts',(61.8126569855623,41.7987197217835,22.9294657090004));
#35453=CARTESIAN_POINT('Ctrl Pts',(61.8991091084337,41.9438641629583,22.783158980636));
#35454=CARTESIAN_POINT('Ctrl Pts',(61.9888546455096,42.0945379161778,22.6294657090004));
#35455=CARTESIAN_POINT('',(61.8199557979604,42.3695257957114,22.6294657090004));
#35456=CARTESIAN_POINT('Origin',(54.9397894030341,37.9543320991532,22.6294657090004));
#35457=CARTESIAN_POINT('',(61.4764348048553,42.3461303516746,22.9294657090004));
#35458=CARTESIAN_POINT('Ctrl Pts',(61.8199557979604,42.3695257957114,22.6294657090004));
#35459=CARTESIAN_POINT('Ctrl Pts',(61.6449848248368,42.3576094246833,22.783158980636));
#35460=CARTESIAN_POINT('Ctrl Pts',(61.4764348048553,42.3461303516746,22.9294657090004));
#35461=CARTESIAN_POINT('',(61.6279342525392,42.6553259804552,22.6294657090004));
#35462=CARTESIAN_POINT('Ctrl Pts',(61.4764348048553,42.3461303516746,22.9294657090004));
#35463=CARTESIAN_POINT('Ctrl Pts',(61.5507686460086,42.4978384872913,22.783158980636));
#35464=CARTESIAN_POINT('Ctrl Pts',(61.6279342525392,42.6553259804552,22.6294657090004));
#35465=CARTESIAN_POINT('',(61.4371833369271,42.915632036449,22.6294657090004));
#35466=CARTESIAN_POINT('Origin',(54.9397894030341,37.9543320991532,22.6294657090004));
#35467=CARTESIAN_POINT('',(61.0967123274698,42.8643142887908,22.9294657090004));
#35468=CARTESIAN_POINT('Ctrl Pts',(61.4371833369271,42.915632036449,22.6294657090004));
#35469=CARTESIAN_POINT('Ctrl Pts',(61.2637658601475,42.8894935575016,22.783158980636));
#35470=CARTESIAN_POINT('Ctrl Pts',(61.0967123274698,42.8643142887908,22.9294657090004));
#35471=CARTESIAN_POINT('',(61.2225053590615,43.184829706062,22.6294657090004));
#35472=CARTESIAN_POINT('Ctrl Pts',(61.0967123274698,42.8643142887908,22.9294657090004));
#35473=CARTESIAN_POINT('Ctrl Pts',(61.1584332074564,43.021576526237,22.783158980636));
#35474=CARTESIAN_POINT('Ctrl Pts',(61.2225053590615,43.184829706062,22.6294657090004));
#35475=CARTESIAN_POINT('',(61.0111717912583,43.4287216446607,22.6294657090004));
#35476=CARTESIAN_POINT('Origin',(54.9397894030341,37.9543320991532,22.6294657090004));
#35477=CARTESIAN_POINT('',(60.6760165438429,43.3498231045251,22.9294657090004));
#35478=CARTESIAN_POINT('Ctrl Pts',(61.0111717912583,43.4287216446607,22.6294657090004));
#35479=CARTESIAN_POINT('Ctrl Pts',(60.8404618755187,43.3885350050589,22.783158980636));
#35480=CARTESIAN_POINT('Ctrl Pts',(60.6760165438429,43.3498231045251,22.9294657090004));
#35481=CARTESIAN_POINT('',(60.7752660274717,43.6795253330662,22.6294657090004));
#35482=CARTESIAN_POINT('Ctrl Pts',(60.6760165438429,43.3498231045251,22.9294657090004));
#35483=CARTESIAN_POINT('Ctrl Pts',(60.7247137203897,43.5115928895569,22.783158980636));
#35484=CARTESIAN_POINT('Ctrl Pts',(60.7752660274716,43.6795253330662,22.6294657090004));
#35485=CARTESIAN_POINT('',(60.5447561975034,43.9053800936578,22.6294657090004));
#35486=CARTESIAN_POINT('Origin',(54.9397894030341,37.9543320991532,22.6294657090004));
#35487=CARTESIAN_POINT('',(60.2171471150049,43.7994258178119,22.9294657090004));
#35488=CARTESIAN_POINT('Ctrl Pts',(60.5447561975034,43.9053800936578,22.6294657090004));
#35489=CARTESIAN_POINT('Ctrl Pts',(60.377889889128,43.8514127288578,22.783158980636));
#35490=CARTESIAN_POINT('Ctrl Pts',(60.2171471150049,43.7994258178119,22.9294657090004));
#35491=CARTESIAN_POINT('',(60.289192561732,44.1361207436891,22.6294657090004));
#35492=CARTESIAN_POINT('Ctrl Pts',(60.2171471150049,43.7994258178119,22.9294657090004));
#35493=CARTESIAN_POINT('Ctrl Pts',(60.2524965164364,43.9646265992003,22.783158980636));
#35494=CARTESIAN_POINT('Ctrl Pts',(60.2891925617321,44.1361207436891,22.6294657090004));
#35495=CARTESIAN_POINT('',(60.0410404744858,44.3424353001052,22.6294657090004));
#35496=CARTESIAN_POINT('Origin',(54.9397894030341,37.9543320991532,22.6294657090004));
#35497=CARTESIAN_POINT('',(59.7231577412963,44.2101303967737,22.9294657090004));
#35498=CARTESIAN_POINT('Ctrl Pts',(60.0410404744858,44.3424353001052,22.6294657090004));
#35499=CARTESIAN_POINT('Ctrl Pts',(59.8791282412257,44.2750463540158,22.783158980636));
#35500=CARTESIAN_POINT('Ctrl Pts',(59.7231577412963,44.2101303967737,22.9294657090004));
#35501=CARTESIAN_POINT('',(59.7675197005607,44.551577370806,22.6294657090004));
#35502=CARTESIAN_POINT('Ctrl Pts',(59.7231577412963,44.2101303967737,22.9294657090004));
#35503=CARTESIAN_POINT('Ctrl Pts',(59.7449241231784,44.3776627905746,22.783158980636));
#35504=CARTESIAN_POINT('Ctrl Pts',(59.7675197005607,44.551577370806,22.6294657090004));
#35505=CARTESIAN_POINT('',(59.5033767672348,44.7369787337132,22.6294657090004));
#35506=CARTESIAN_POINT('Origin',(54.9397894030341,37.9543320991532,22.6294657090004));
#35507=CARTESIAN_POINT('',(59.1973358404969,44.5792036701988,22.9294657090004));
#35508=CARTESIAN_POINT('Ctrl Pts',(59.5033767672348,44.7369787337132,22.6294657090004));
#35509=CARTESIAN_POINT('Ctrl Pts',(59.3474961082889,44.6566166686521,22.7831589806361));
#35510=CARTESIAN_POINT('Ctrl Pts',(59.1973358404969,44.5792036701988,22.9294657090004));
#35511=CARTESIAN_POINT('',(59.2137190907787,44.9231304191088,22.6294657090004));
#35512=CARTESIAN_POINT('Ctrl Pts',(59.1973358404969,44.5792036701988,22.9294657090004));
#35513=CARTESIAN_POINT('Ctrl Pts',(59.2053743511492,44.7479527759724,22.783158980636));
#35514=CARTESIAN_POINT('Ctrl Pts',(59.2137190907787,44.9231304191088,22.6294657090004));
#35515=CARTESIAN_POINT('',(58.935343139014,45.0863847730261,22.6294657090004));
#35516=CARTESIAN_POINT('Origin',(54.9397894030341,37.9543320991532,22.6294657090004));
#35517=CARTESIAN_POINT('',(58.6431806706019,44.9041895163456,22.9294657090004));
#35518=CARTESIAN_POINT('Ctrl Pts',(58.935343139014,45.0863847730261,22.6294657090004));
#35519=CARTESIAN_POINT('Ctrl Pts',(58.7865314144489,44.9935843852776,22.783158980636));
#35520=CARTESIAN_POINT('Ctrl Pts',(58.6431806706019,44.9041895163456,22.9294657090004));
#35521=CARTESIAN_POINT('',(58.6314761840735,45.2483072643631,22.6294657090004));
#35522=CARTESIAN_POINT('Ctrl Pts',(58.6431806706019,44.9041895163456,22.9294657090004));
#35523=CARTESIAN_POINT('Ctrl Pts',(58.6374378150623,45.0730323366345,22.783158980636));
#35524=CARTESIAN_POINT('Ctrl Pts',(58.6314761840736,45.2483072643631,22.6294657090004));
#35525=CARTESIAN_POINT('',(58.3407197599002,45.3883281785002,22.6294657090004));
#35526=CARTESIAN_POINT('Origin',(54.9397894030341,37.9543320991532,22.6294657090004));
#35527=CARTESIAN_POINT('',(58.0643800428377,45.1829252080266,22.9294657090004));
#35528=CARTESIAN_POINT('Ctrl Pts',(58.3407197599002,45.3883281785002,22.6294657090004));
#35529=CARTESIAN_POINT('Ctrl Pts',(58.1999672871908,45.2837070393338,22.7831589806361));
#35530=CARTESIAN_POINT('Ctrl Pts',(58.0643800428377,45.1829252080266,22.9294657090004));
#35531=CARTESIAN_POINT('',(58.024665710926,45.5249439083142,22.6294657090004));
#35532=CARTESIAN_POINT('Ctrl Pts',(58.0643800428377,45.1829252080266,22.9294657090004));
#35533=CARTESIAN_POINT('Ctrl Pts',(58.0448940388624,45.3507381217191,22.783158980636));
#35534=CARTESIAN_POINT('Ctrl Pts',(58.024665710926,45.5249439083142,22.6294657090004));
#35535=CARTESIAN_POINT('',(57.7234637503755,45.6407995665893,22.6294657090004));
#35536=CARTESIAN_POINT('Origin',(54.9397894030341,37.9543320991532,22.6294657090004));
#35537=CARTESIAN_POINT('',(57.4647857798868,45.413555805202,22.9294657090004));
#35538=CARTESIAN_POINT('Ctrl Pts',(57.7234637503755,45.6407995665893,22.6294657090004));
#35539=CARTESIAN_POINT('Ctrl Pts',(57.5917072140051,45.5250539124248,22.783158980636));
#35540=CARTESIAN_POINT('Ctrl Pts',(57.4647857798868,45.4135558052021,22.9294657090004));
#35541=CARTESIAN_POINT('',(57.3973258949183,45.7511993797383,22.6294657090004));
#35542=CARTESIAN_POINT('Ctrl Pts',(57.4647857798868,45.413555805202,22.9294657090003));
#35543=CARTESIAN_POINT('Ctrl Pts',(57.4316863036172,45.5792220450446,22.783158980636));
#35544=CARTESIAN_POINT('Ctrl Pts',(57.3973258949183,45.7511993797383,22.6294657090004));
#35545=CARTESIAN_POINT('',(57.0876828473432,45.8421187818605,22.6294657090004));
#35546=CARTESIAN_POINT('Origin',(54.9397894030341,37.9543320991532,22.6294657090004));
#35547=CARTESIAN_POINT('',(56.8483880826431,45.594546499299,22.9294657090004));
#35548=CARTESIAN_POINT('Ctrl Pts',(57.0876828473432,45.8421187818605,22.6294657090004));
#35549=CARTESIAN_POINT('Ctrl Pts',(56.9657990653231,45.7160188809296,22.783158980636));
#35550=CARTESIAN_POINT('Ctrl Pts',(56.8483880826431,45.594546499299,22.9294657090004));
#35551=CARTESIAN_POINT('',(56.753631579022,45.9255679858027,22.6294657090004));
#35552=CARTESIAN_POINT('Ctrl Pts',(56.8483880826431,45.594546499299,22.9294657090004));
#35553=CARTESIAN_POINT('Ctrl Pts',(56.8018954056327,45.7569635837985,22.783158980636));
#35554=CARTESIAN_POINT('Ctrl Pts',(56.753631579022,45.9255679858026,22.6294657090004));
#35555=CARTESIAN_POINT('',(56.4376080678164,45.9909460781515,22.6294657090004));
#35556=CARTESIAN_POINT('Origin',(54.9397894030341,37.9543320991532,22.6294657090004));
#35557=CARTESIAN_POINT('',(56.2192889760832,45.7246928271096,22.9294657090004));
#35558=CARTESIAN_POINT('Ctrl Pts',(56.4376080678164,45.9909460781514,22.6294657090004));
#35559=CARTESIAN_POINT('Ctrl Pts',(56.3264081566065,45.85533110449,22.783158980636));
#35560=CARTESIAN_POINT('Ctrl Pts',(56.2192889760832,45.7246928271096,22.9294657090003));
#35561=CARTESIAN_POINT('',(56.0978664427074,46.0468893322027,22.6294657090004));
#35562=CARTESIAN_POINT('Ctrl Pts',(56.2192889760832,45.7246928271096,22.9294657090004));
#35563=CARTESIAN_POINT('Ctrl Pts',(56.1597124994268,45.8827798973656,22.783158980636));
#35564=CARTESIAN_POINT('Ctrl Pts',(56.0978664427074,46.0468893322027,22.6294657090004));
#35565=CARTESIAN_POINT('',(55.7775655521983,46.0862910343602,22.6294657090004));
#35566=CARTESIAN_POINT('Origin',(54.9397894030341,37.9543320991532,22.6294657090004));
#35567=CARTESIAN_POINT('',(55.5816750109672,45.803128686295,22.9294657090004));
#35568=CARTESIAN_POINT('Ctrl Pts',(55.7775655521982,46.0862910343601,22.6294657090004));
#35569=CARTESIAN_POINT('Ctrl Pts',(55.6777895288609,45.9420634832429,22.783158980636));
#35570=CARTESIAN_POINT('Ctrl Pts',(55.5816750109672,45.803128686295,22.9294657090003));
#35571=CARTESIAN_POINT('',(55.434394494763,46.1143560453948,22.6294657090004));
#35572=CARTESIAN_POINT('Ctrl Pts',(55.5816750109672,45.803128686295,22.9294657090003));
#35573=CARTESIAN_POINT('Ctrl Pts',(55.5094112062876,45.9558336989374,22.783158980636));
#35574=CARTESIAN_POINT('Ctrl Pts',(55.434394494763,46.1143560453948,22.6294657090004));
#35575=CARTESIAN_POINT('',(55.1119477745308,46.1275191455338,22.6294657090004));
#35576=CARTESIAN_POINT('Origin',(54.9397894030341,37.9543320991532,22.6294657090004));
#35577=CARTESIAN_POINT('',(54.9397894030341,45.8293320991532,22.9294657090004));
#35578=CARTESIAN_POINT('Ctrl Pts',(55.1119477745308,46.1275191455338,22.6294657090004));
#35579=CARTESIAN_POINT('Ctrl Pts',(55.0242596320395,45.9756388275175,22.783158980636));
#35580=CARTESIAN_POINT('Ctrl Pts',(54.9397894030341,45.8293320991532,22.9294657090004));
#35581=CARTESIAN_POINT('',(54.7676310315374,46.1275191455338,22.6294657090004));
#35582=CARTESIAN_POINT('Ctrl Pts',(54.9397894030341,45.8293320991532,22.9294657090004));
#35583=CARTESIAN_POINT('Ctrl Pts',(54.8553191740288,45.9756388275175,22.7831589806361));
#35584=CARTESIAN_POINT('Ctrl Pts',(54.7676310315374,46.1275191455338,22.6294657090004));
#35585=CARTESIAN_POINT('',(54.4451843113051,46.1143560453948,22.6294657090004));
#35586=CARTESIAN_POINT('Origin',(54.9397894030341,37.9543320991532,22.6294657090004));
#35587=CARTESIAN_POINT('',(54.297903795101,45.803128686295,22.9294657090004));
#35588=CARTESIAN_POINT('Ctrl Pts',(54.4451843113051,46.1143560453948,22.6294657090004));
#35589=CARTESIAN_POINT('Ctrl Pts',(54.3701675997806,45.9558336989374,22.783158980636));
#35590=CARTESIAN_POINT('Ctrl Pts',(54.297903795101,45.803128686295,22.9294657090004));
#35591=CARTESIAN_POINT('',(54.1020132538699,46.0862910343601,22.6294657090004));
#35592=CARTESIAN_POINT('Ctrl Pts',(54.297903795101,45.803128686295,22.9294657090004));
#35593=CARTESIAN_POINT('Ctrl Pts',(54.2017892772072,45.9420634832428,22.783158980636));
#35594=CARTESIAN_POINT('Ctrl Pts',(54.1020132538699,46.0862910343601,22.6294657090004));
#35595=CARTESIAN_POINT('',(53.7817123633608,46.0468893322027,22.6294657090004));
#35596=CARTESIAN_POINT('Origin',(54.9397894030341,37.9543320991532,22.6294657090004));
#35597=CARTESIAN_POINT('',(53.660289829985,45.7246928271096,22.9294657090004));
#35598=CARTESIAN_POINT('Ctrl Pts',(53.7817123633608,46.0468893322027,22.6294657090004));
#35599=CARTESIAN_POINT('Ctrl Pts',(53.7198663066414,45.8827798973656,22.7831589806361));
#35600=CARTESIAN_POINT('Ctrl Pts',(53.660289829985,45.7246928271096,22.9294657090004));
#35601=CARTESIAN_POINT('',(53.4419707382517,45.9909460781514,22.6294657090004));
#35602=CARTESIAN_POINT('Ctrl Pts',(53.660289829985,45.7246928271096,22.9294657090004));
#35603=CARTESIAN_POINT('Ctrl Pts',(53.5531706494617,45.8553311044899,22.783158980636));
#35604=CARTESIAN_POINT('Ctrl Pts',(53.4419707382517,45.9909460781514,22.6294657090004));
#35605=CARTESIAN_POINT('',(53.1259472270462,45.9255679858026,22.6294657090004));
#35606=CARTESIAN_POINT('Origin',(54.9397894030341,37.9543320991532,22.6294657090004));
#35607=CARTESIAN_POINT('',(53.0311907234251,45.594546499299,22.9294657090004));
#35608=CARTESIAN_POINT('Ctrl Pts',(53.1259472270462,45.9255679858026,22.6294657090004));
#35609=CARTESIAN_POINT('Ctrl Pts',(53.0776834004354,45.7569635837984,22.783158980636));
#35610=CARTESIAN_POINT('Ctrl Pts',(53.0311907234251,45.594546499299,22.9294657090004));
#35611=CARTESIAN_POINT('',(52.791895958725,45.8421187818605,22.6294657090004));
#35612=CARTESIAN_POINT('Ctrl Pts',(53.0311907234251,45.594546499299,22.9294657090004));
#35613=CARTESIAN_POINT('Ctrl Pts',(52.9137797407451,45.7160188809296,22.783158980636));
#35614=CARTESIAN_POINT('Ctrl Pts',(52.791895958725,45.8421187818605,22.6294657090004));
#35615=CARTESIAN_POINT('',(52.4822529111499,45.7511993797382,22.6294657090004));
#35616=CARTESIAN_POINT('Origin',(54.9397894030341,37.9543320991532,22.6294657090004));
#35617=CARTESIAN_POINT('',(52.4147930261813,45.413555805202,22.9294657090004));
#35618=CARTESIAN_POINT('Ctrl Pts',(52.4822529111499,45.7511993797382,22.6294657090004));
#35619=CARTESIAN_POINT('Ctrl Pts',(52.447892502451,45.5792220450445,22.783158980636));
#35620=CARTESIAN_POINT('Ctrl Pts',(52.4147930261813,45.413555805202,22.9294657090004));
#35621=CARTESIAN_POINT('',(52.1561150556927,45.6407995665893,22.6294657090004));
#35622=CARTESIAN_POINT('Ctrl Pts',(52.4147930261813,45.413555805202,22.9294657090004));
#35623=CARTESIAN_POINT('Ctrl Pts',(52.2878715920631,45.5250539124247,22.783158980636));
#35624=CARTESIAN_POINT('Ctrl Pts',(52.1561150556927,45.6407995665893,22.6294657090004));
#35625=CARTESIAN_POINT('',(51.8549130951421,45.5249439083141,22.6294657090004));
#35626=CARTESIAN_POINT('Origin',(54.9397894030341,37.9543320991532,22.6294657090004));
#35627=CARTESIAN_POINT('',(51.8151987632305,45.1829252080266,22.9294657090004));
#35628=CARTESIAN_POINT('Ctrl Pts',(51.8549130951421,45.5249439083141,22.6294657090004));
#35629=CARTESIAN_POINT('Ctrl Pts',(51.8346847672058,45.3507381217191,22.783158980636));
#35630=CARTESIAN_POINT('Ctrl Pts',(51.8151987632305,45.1829252080266,22.9294657090004));
#35631=CARTESIAN_POINT('',(51.5388590461679,45.3883281785002,22.6294657090004));
#35632=CARTESIAN_POINT('Ctrl Pts',(51.8151987632305,45.1829252080266,22.9294657090004));
#35633=CARTESIAN_POINT('Ctrl Pts',(51.6796115188774,45.2837070393337,22.783158980636));
#35634=CARTESIAN_POINT('Ctrl Pts',(51.5388590461679,45.3883281785002,22.6294657090004));
#35635=CARTESIAN_POINT('',(51.2481026219946,45.2483072643631,22.6294657090004));
#35636=CARTESIAN_POINT('Origin',(54.9397894030341,37.9543320991532,22.6294657090004));
#35637=CARTESIAN_POINT('',(51.2363981354663,44.9041895163455,22.9294657090004));
#35638=CARTESIAN_POINT('Ctrl Pts',(51.2481026219946,45.2483072643631,22.6294657090004));
#35639=CARTESIAN_POINT('Ctrl Pts',(51.2421409910059,45.0730323366345,22.783158980636));
#35640=CARTESIAN_POINT('Ctrl Pts',(51.2363981354663,44.9041895163455,22.9294657090004));
#35641=CARTESIAN_POINT('',(50.9442356670542,45.086384773026,22.6294657090004));
#35642=CARTESIAN_POINT('Ctrl Pts',(51.2363981354663,44.9041895163455,22.9294657090004));
#35643=CARTESIAN_POINT('Ctrl Pts',(51.0930473916193,44.9935843852776,22.783158980636));
#35644=CARTESIAN_POINT('Ctrl Pts',(50.9442356670542,45.0863847730261,22.6294657090004));
#35645=CARTESIAN_POINT('',(50.6658597152895,44.9231304191087,22.6294657090004));
#35646=CARTESIAN_POINT('Origin',(54.9397894030341,37.9543320991532,22.6294657090004));
#35647=CARTESIAN_POINT('',(50.6822429655713,44.5792036701988,22.9294657090004));
#35648=CARTESIAN_POINT('Ctrl Pts',(50.6658597152895,44.9231304191087,22.6294657090004));
#35649=CARTESIAN_POINT('Ctrl Pts',(50.674204454919,44.7479527759724,22.783158980636));
#35650=CARTESIAN_POINT('Ctrl Pts',(50.6822429655713,44.5792036701988,22.9294657090004));
#35651=CARTESIAN_POINT('',(50.3762020388334,44.7369787337131,22.6294657090004));
#35652=CARTESIAN_POINT('Ctrl Pts',(50.6822429655713,44.5792036701988,22.9294657090004));
#35653=CARTESIAN_POINT('Ctrl Pts',(50.5320826977793,44.6566166686521,22.783158980636));
#35654=CARTESIAN_POINT('Ctrl Pts',(50.3762020388334,44.7369787337131,22.6294657090004));
#35655=CARTESIAN_POINT('',(50.1120591055075,44.5515773708059,22.6294657090004));
#35656=CARTESIAN_POINT('Origin',(54.9397894030341,37.9543320991532,22.6294657090004));
#35657=CARTESIAN_POINT('',(50.1564210647719,44.2101303967736,22.9294657090004));
#35658=CARTESIAN_POINT('Ctrl Pts',(50.1120591055075,44.5515773708059,22.6294657090004));
#35659=CARTESIAN_POINT('Ctrl Pts',(50.1346546828898,44.3776627905745,22.783158980636));
#35660=CARTESIAN_POINT('Ctrl Pts',(50.1564210647719,44.2101303967736,22.9294657090004));
#35661=CARTESIAN_POINT('',(49.8385383315824,44.3424353001052,22.6294657090004));
#35662=CARTESIAN_POINT('Ctrl Pts',(50.1564210647719,44.2101303967736,22.9294657090004));
#35663=CARTESIAN_POINT('Ctrl Pts',(50.0004505648425,44.2750463540157,22.783158980636));
#35664=CARTESIAN_POINT('Ctrl Pts',(49.8385383315824,44.3424353001052,22.6294657090004));
#35665=CARTESIAN_POINT('',(49.5903862443362,44.1361207436891,22.6294657090004));
#35666=CARTESIAN_POINT('Origin',(54.9397894030341,37.9543320991532,22.6294657090004));
#35667=CARTESIAN_POINT('',(49.6624316910633,43.7994258178118,22.9294657090004));
#35668=CARTESIAN_POINT('Ctrl Pts',(49.5903862443362,44.1361207436891,22.6294657090004));
#35669=CARTESIAN_POINT('Ctrl Pts',(49.6270822896318,43.9646265992002,22.783158980636));
#35670=CARTESIAN_POINT('Ctrl Pts',(49.6624316910633,43.7994258178118,22.9294657090004));
#35671=CARTESIAN_POINT('',(49.3348226085648,43.9053800936577,22.6294657090004));
#35672=CARTESIAN_POINT('Ctrl Pts',(49.6624316910633,43.7994258178118,22.9294657090004));
#35673=CARTESIAN_POINT('Ctrl Pts',(49.5016889169402,43.8514127288577,22.783158980636));
#35674=CARTESIAN_POINT('Ctrl Pts',(49.3348226085648,43.9053800936577,22.6294657090004));
#35675=CARTESIAN_POINT('',(49.1043127785965,43.6795253330662,22.6294657090004));
#35676=CARTESIAN_POINT('Origin',(54.9397894030341,37.9543320991532,22.6294657090004));
#35677=CARTESIAN_POINT('',(49.2035622622253,43.349823104525,22.9294657090004));
#35678=CARTESIAN_POINT('Ctrl Pts',(49.1043127785965,43.6795253330662,22.6294657090004));
#35679=CARTESIAN_POINT('Ctrl Pts',(49.1548650856785,43.5115928895569,22.7831589806361));
#35680=CARTESIAN_POINT('Ctrl Pts',(49.2035622622253,43.349823104525,22.9294657090004));
#35681=CARTESIAN_POINT('',(48.8684070148099,43.4287216446606,22.6294657090004));
#35682=CARTESIAN_POINT('Ctrl Pts',(49.2035622622253,43.349823104525,22.9294657090004));
#35683=CARTESIAN_POINT('Ctrl Pts',(49.0391169305495,43.3885350050588,22.783158980636));
#35684=CARTESIAN_POINT('Ctrl Pts',(48.8684070148099,43.4287216446606,22.6294657090004));
#35685=CARTESIAN_POINT('',(48.6570734470067,43.184829706062,22.6294657090004));
#35686=CARTESIAN_POINT('Origin',(54.9397894030341,37.9543320991532,22.6294657090004));
#35687=CARTESIAN_POINT('',(48.7828664785984,42.8643142887907,22.9294657090004));
#35688=CARTESIAN_POINT('Ctrl Pts',(48.6570734470067,43.184829706062,22.6294657090004));
#35689=CARTESIAN_POINT('Ctrl Pts',(48.7211455986118,43.0215765262369,22.7831589806361));
#35690=CARTESIAN_POINT('Ctrl Pts',(48.7828664785984,42.8643142887908,22.9294657090004));
#35691=CARTESIAN_POINT('',(48.4423954691411,42.9156320364489,22.6294657090004));
#35692=CARTESIAN_POINT('Ctrl Pts',(48.7828664785984,42.8643142887907,22.9294657090004));
#35693=CARTESIAN_POINT('Ctrl Pts',(48.6158129459207,42.8894935575015,22.783158980636));
#35694=CARTESIAN_POINT('Ctrl Pts',(48.4423954691411,42.9156320364489,22.6294657090004));
#35695=CARTESIAN_POINT('',(48.251644553529,42.6553259804552,22.6294657090004));
#35696=CARTESIAN_POINT('Origin',(54.9397894030341,37.9543320991532,22.6294657090004));
#35697=CARTESIAN_POINT('',(48.4031440012129,42.3461303516745,22.9294657090004));
#35698=CARTESIAN_POINT('Ctrl Pts',(48.251644553529,42.6553259804551,22.6294657090004));
#35699=CARTESIAN_POINT('Ctrl Pts',(48.3288101600596,42.4978384872912,22.7831589806361));
#35700=CARTESIAN_POINT('Ctrl Pts',(48.4031440012129,42.3461303516745,22.9294657090004));
#35701=CARTESIAN_POINT('',(48.0596230081078,42.3695257957113,22.6294657090004));
#35702=CARTESIAN_POINT('Ctrl Pts',(48.4031440012129,42.3461303516745,22.9294657090004));
#35703=CARTESIAN_POINT('Ctrl Pts',(48.2345939812314,42.3576094246832,22.783158980636));
#35704=CARTESIAN_POINT('Ctrl Pts',(48.0596230081078,42.3695257957113,22.6294657090004));
#35705=CARTESIAN_POINT('',(47.8907241605586,42.0945379161777,22.6294657090004));
#35706=CARTESIAN_POINT('Origin',(54.9397894030341,37.9543320991532,22.6294657090004));
#35707=CARTESIAN_POINT('',(48.0669218205059,41.7987197217834,22.9294657090004));
#35708=CARTESIAN_POINT('Ctrl Pts',(47.8907241605586,42.0945379161777,22.6294657090004));
#35709=CARTESIAN_POINT('Ctrl Pts',(47.9804696976345,41.9438641629582,22.783158980636));
#35710=CARTESIAN_POINT('Ctrl Pts',(48.0669218205059,41.7987197217834,22.9294657090004));
#35711=CARTESIAN_POINT('',(47.7226369192852,41.7940371693788,22.6294657090004));
#35712=CARTESIAN_POINT('Ctrl Pts',(48.0669218205059,41.7987197217834,22.9294657090003));
#35713=CARTESIAN_POINT('Ctrl Pts',(47.8979969857948,41.7964222077531,22.783158980636));
#35714=CARTESIAN_POINT('Ctrl Pts',(47.7226369192852,41.7940371693788,22.6294657090003));
#35715=CARTESIAN_POINT('',(47.5767141337629,41.5061974652738,22.6294657090004));
#35716=CARTESIAN_POINT('Origin',(54.9397894030341,37.9543320991532,22.6294657090004));
#35717=CARTESIAN_POINT('',(47.7764374396173,41.2257253265431,22.9294657090004));
#35718=CARTESIAN_POINT('Ctrl Pts',(47.5767141337629,41.5061974652738,22.6294657090004));
#35719=CARTESIAN_POINT('Ctrl Pts',(47.678442359642,41.363340160967,22.783158980636));
#35720=CARTESIAN_POINT('Ctrl Pts',(47.7764374396173,41.225725326543,22.9294657090003));
#35721=CARTESIAN_POINT('',(47.4336797894956,41.1929959393107,22.6294657090004));
#35722=CARTESIAN_POINT('Ctrl Pts',(47.7764374396173,41.2257253265431,22.9294657090004));
#35723=CARTESIAN_POINT('Ctrl Pts',(47.6082619570809,41.2096665150506,22.783158980636));
#35724=CARTESIAN_POINT('Ctrl Pts',(47.4336797894956,41.1929959393107,22.6294657090004));
#35725=CARTESIAN_POINT('',(47.3117041580624,40.8942199363749,22.6294657090004));
#35726=CARTESIAN_POINT('Origin',(54.9397894030341,37.9543320991532,22.6294657090004));
#35727=CARTESIAN_POINT('',(47.5336239841754,40.6309603491163,22.9294657090004));
#35728=CARTESIAN_POINT('Ctrl Pts',(47.3117041580624,40.8942199363749,22.6294657090004));
#35729=CARTESIAN_POINT('Ctrl Pts',(47.4247380881853,40.7601297727712,22.7831589806361));
#35730=CARTESIAN_POINT('Ctrl Pts',(47.5336239841754,40.6309603491163,22.9294657090004));
#35731=CARTESIAN_POINT('',(47.1946745807631,40.5704019357283,22.6294657090004));
#35732=CARTESIAN_POINT('Ctrl Pts',(47.5336239841754,40.6309603491163,22.9294657090004));
#35733=CARTESIAN_POINT('Ctrl Pts',(47.367317033903,40.6012471089026,22.7831589806361));
#35734=CARTESIAN_POINT('Ctrl Pts',(47.1946745807631,40.5704019357283,22.6294657090004));
#35735=CARTESIAN_POINT('',(47.0974578311216,40.2626779389666,22.6294657090004));
#35736=CARTESIAN_POINT('Origin',(54.9397894030341,37.9543320991532,22.6294657090004));
#35737=CARTESIAN_POINT('',(47.3400973376647,40.0183828522986,22.9294657090004));
#35738=CARTESIAN_POINT('Ctrl Pts',(47.0974578311216,40.2626779389666,22.6294657090004));
#35739=CARTESIAN_POINT('Ctrl Pts',(47.2210452433328,40.1382472639815,22.783158980636));
#35740=CARTESIAN_POINT('Ctrl Pts',(47.3400973376646,40.0183828522986,22.9294657090004));
#35741=CARTESIAN_POINT('',(47.0072118333189,39.9303984190046,22.6294657090004));
#35742=CARTESIAN_POINT('Ctrl Pts',(47.3400973376647,40.0183828522986,22.9294657090004));
#35743=CARTESIAN_POINT('Ctrl Pts',(47.1767656649717,39.9752129200749,22.783158980636));
#35744=CARTESIAN_POINT('Ctrl Pts',(47.0072118333189,39.9303984190046,22.6294657090004));
#35745=CARTESIAN_POINT('',(46.9354009268983,39.6157742808447,22.6294657090004));
#35746=CARTESIAN_POINT('Origin',(54.9397894030341,37.9543320991532,22.6294657090004));
#35747=CARTESIAN_POINT('',(47.197145387988,39.3920694382632,22.9294657090004));
#35748=CARTESIAN_POINT('Ctrl Pts',(46.9354009268983,39.6157742808447,22.6294657090004));
#35749=CARTESIAN_POINT('Ctrl Pts',(47.0687193673599,39.5018311600905,22.7831589806361));
#35750=CARTESIAN_POINT('Ctrl Pts',(47.1971453879881,39.3920694382632,22.9294657090004));
#35751=CARTESIAN_POINT('',(46.872539080818,39.2772445069503,22.6294657090004));
#35752=CARTESIAN_POINT('Ctrl Pts',(47.197145387988,39.3920694382632,22.9294657090004));
#35753=CARTESIAN_POINT('Ctrl Pts',(47.0378759382083,39.3357301028059,22.783158980636));
#35754=CARTESIAN_POINT('Ctrl Pts',(46.872539080818,39.2772445069503,22.6294657090004));
#35755=CARTESIAN_POINT('',(46.8266119073525,38.9578139991222,22.6294657090004));
#35756=CARTESIAN_POINT('Origin',(54.9397894030341,37.9543320991532,22.6294657090004));
#35757=CARTESIAN_POINT('',(47.1057194567852,38.7561881194459,22.9294657090004));
#35758=CARTESIAN_POINT('Ctrl Pts',(46.8266119073525,38.9578139991222,22.6294657090004));
#35759=CARTESIAN_POINT('Ctrl Pts',(46.9687741638393,38.8551167052684,22.783158980636));
#35760=CARTESIAN_POINT('Ctrl Pts',(47.1057194567852,38.7561881194459,22.9294657090004));
#35761=CARTESIAN_POINT('',(46.7915525482088,38.6152868310873,22.6294657090004));
#35762=CARTESIAN_POINT('Ctrl Pts',(47.1057194567852,38.7561881194459,22.9294657090004));
#35763=CARTESIAN_POINT('Ctrl Pts',(46.9515721418295,38.6870543097372,22.783158980636));
#35764=CARTESIAN_POINT('Ctrl Pts',(46.7915525482088,38.6152868310873,22.6294657090004));
#35765=CARTESIAN_POINT('',(46.7718147454605,38.2931757109183,22.6294657090004));
#35766=CARTESIAN_POINT('Origin',(54.9397894030341,37.9543320991532,22.6294657090004));
#35767=CARTESIAN_POINT('Ctrl Pts',(46.7718147454605,38.2931757109183,22.6294657090004));
#35768=CARTESIAN_POINT('Ctrl Pts',(46.9218747516106,38.2024076775115,22.783158980636));
#35769=CARTESIAN_POINT('Ctrl Pts',(47.0664279685441,38.1149705811105,22.9294657090004));
#35770=CARTESIAN_POINT('Origin',(54.9397894030341,37.9543320991532,8.12867690713751));
#35771=CARTESIAN_POINT('',(56.9397894030341,37.9543320991532,8.12867690713751));
#35772=CARTESIAN_POINT('Origin',(54.9397894030341,37.9543320991532,8.12867690713751));
#35773=CARTESIAN_POINT('',(53.7817123633608,46.0468893322027,35.0304657090004));
#35774=CARTESIAN_POINT('',(54.1020132538699,46.0862910343601,35.0304657090004));
#35775=CARTESIAN_POINT('Origin',(54.9397894030341,37.9543320991532,8.12867690713751));
#35776=CARTESIAN_POINT('',(53.4419707382517,45.9909460781514,35.0304657090004));
#35777=CARTESIAN_POINT('',(53.1259472270462,45.9255679858026,35.0304657090004));
#35778=CARTESIAN_POINT('Origin',(54.9397894030341,37.9543320991532,8.12867690713751));
#35779=CARTESIAN_POINT('',(52.791895958725,45.8421187818605,35.0304657090004));
#35780=CARTESIAN_POINT('',(52.4822529111499,45.7511993797382,35.0304657090004));
#35781=CARTESIAN_POINT('Origin',(54.9397894030341,37.9543320991532,8.12867690713751));
#35782=CARTESIAN_POINT('',(52.1561150556927,45.6407995665893,35.0304657090004));
#35783=CARTESIAN_POINT('',(51.8549130951421,45.5249439083141,35.0304657090004));
#35784=CARTESIAN_POINT('Origin',(54.9397894030341,37.9543320991532,8.12867690713751));
#35785=CARTESIAN_POINT('',(51.5388590461679,45.3883281785002,35.0304657090004));
#35786=CARTESIAN_POINT('',(51.2481026219946,45.2483072643631,35.0304657090004));
#35787=CARTESIAN_POINT('Origin',(54.9397894030341,37.9543320991532,8.12867690713751));
#35788=CARTESIAN_POINT('',(50.9442356670542,45.086384773026,35.0304657090004));
#35789=CARTESIAN_POINT('',(50.6658597152895,44.9231304191087,35.0304657090004));
#35790=CARTESIAN_POINT('Origin',(54.9397894030341,37.9543320991532,8.12867690713751));
#35791=CARTESIAN_POINT('',(50.3762020388334,44.7369787337131,35.0304657090004));
#35792=CARTESIAN_POINT('',(50.1120591055075,44.5515773708059,35.0304657090004));
#35793=CARTESIAN_POINT('Origin',(54.9397894030341,37.9543320991532,8.12867690713751));
#35794=CARTESIAN_POINT('',(49.8385383315824,44.3424353001052,35.0304657090004));
#35795=CARTESIAN_POINT('',(49.5903862443362,44.1361207436891,35.0304657090004));
#35796=CARTESIAN_POINT('Origin',(54.9397894030341,37.9543320991532,8.12867690713751));
#35797=CARTESIAN_POINT('',(49.3348226085648,43.9053800936577,35.0304657090004));
#35798=CARTESIAN_POINT('',(49.1043127785965,43.6795253330662,35.0304657090004));
#35799=CARTESIAN_POINT('Origin',(54.9397894030341,37.9543320991532,8.12867690713751));
#35800=CARTESIAN_POINT('',(48.8684070148099,43.4287216446606,35.0304657090004));
#35801=CARTESIAN_POINT('',(48.6570734470067,43.184829706062,35.0304657090004));
#35802=CARTESIAN_POINT('Origin',(54.9397894030341,37.9543320991532,8.12867690713751));
#35803=CARTESIAN_POINT('',(48.4423954691411,42.9156320364489,35.0304657090004));
#35804=CARTESIAN_POINT('',(48.251644553529,42.6553259804552,35.0304657090004));
#35805=CARTESIAN_POINT('Origin',(54.9397894030341,37.9543320991532,8.12867690713751));
#35806=CARTESIAN_POINT('',(48.0596230081078,42.3695257957113,35.0304657090004));
#35807=CARTESIAN_POINT('',(47.8907241605586,42.0945379161777,35.0304657090004));
#35808=CARTESIAN_POINT('Origin',(54.9397894030341,37.9543320991532,8.12867690713751));
#35809=CARTESIAN_POINT('',(47.7226369192852,41.7940371693788,35.0304657090004));
#35810=CARTESIAN_POINT('',(47.5767141337629,41.5061974652738,35.0304657090004));
#35811=CARTESIAN_POINT('Origin',(54.9397894030341,37.9543320991532,8.12867690713751));
#35812=CARTESIAN_POINT('',(47.4336797894956,41.1929959393107,35.0304657090004));
#35813=CARTESIAN_POINT('',(47.3117041580624,40.8942199363749,35.0304657090004));
#35814=CARTESIAN_POINT('Origin',(54.9397894030341,37.9543320991532,8.12867690713751));
#35815=CARTESIAN_POINT('',(47.1946745807631,40.5704019357283,35.0304657090004));
#35816=CARTESIAN_POINT('',(47.0974578311216,40.2626779389666,35.0304657090004));
#35817=CARTESIAN_POINT('Origin',(54.9397894030341,37.9543320991532,8.12867690713751));
#35818=CARTESIAN_POINT('',(47.0072118333189,39.9303984190046,35.0304657090004));
#35819=CARTESIAN_POINT('',(46.9354009268983,39.6157742808447,35.0304657090004));
#35820=CARTESIAN_POINT('Origin',(54.9397894030341,37.9543320991532,8.12867690713751));
#35821=CARTESIAN_POINT('',(46.872539080818,39.2772445069503,35.0304657090004));
#35822=CARTESIAN_POINT('',(46.8266119073525,38.9578139991222,35.0304657090004));
#35823=CARTESIAN_POINT('Origin',(54.9397894030341,37.9543320991532,8.12867690713751));
#35824=CARTESIAN_POINT('',(46.7915525482088,38.6152868310873,35.0304657090004));
#35825=CARTESIAN_POINT('',(46.7718147454605,38.2931757109183,35.0304657090004));
#35826=CARTESIAN_POINT('Origin',(54.9397894030341,37.9543320991532,8.12867690713751));
#35827=CARTESIAN_POINT('',(46.764791187504,37.9489306105331,35.0304657090004));
#35828=CARTESIAN_POINT('',(46.7713741072936,37.6262824743834,35.0304657090004));
#35829=CARTESIAN_POINT('Origin',(54.9397894030341,37.9543320991532,8.12867690713751));
#35830=CARTESIAN_POINT('',(46.7924330911438,37.2826103359946,35.0304657090004));
#35831=CARTESIAN_POINT('',(46.8252929252262,36.961572353977,35.0304657090004));
#35832=CARTESIAN_POINT('Origin',(54.9397894030341,37.9543320991532,8.12867690713751));
#35833=CARTESIAN_POINT('',(46.8742943068201,36.6207602589635,35.0304657090004));
#35834=CARTESIAN_POINT('',(46.9332123784209,36.3034688858808,35.0304657090004));
#35835=CARTESIAN_POINT('Origin',(54.9397894030341,37.9543320991532,8.12867690713751));
#35836=CARTESIAN_POINT('',(47.0098300616486,35.967784882505,35.0304657090004));
#35837=CARTESIAN_POINT('',(47.0944142807223,35.6563516400958,35.0304657090004));
#35838=CARTESIAN_POINT('Origin',(54.9397894030341,37.9543320991532,8.12867690713751));
#35839=CARTESIAN_POINT('',(47.1981383875429,35.3280296500161,35.0304657090004));
#35840=CARTESIAN_POINT('',(47.3078258600668,35.0245270751256,35.0304657090004));
#35841=CARTESIAN_POINT('Origin',(54.9397894030341,37.9543320991532,8.12867690713751));
#35842=CARTESIAN_POINT('',(47.4379661236628,34.7057520270169,35.0304657090004));
#35843=CARTESIAN_POINT('',(47.5720268976044,34.4121998792066,35.0304657090004));
#35844=CARTESIAN_POINT('Origin',(54.9397894030341,37.9543320991532,8.12867690713751));
#35845=CARTESIAN_POINT('',(47.7277172559931,34.1050931684197,35.0304657090004));
#35846=CARTESIAN_POINT('',(47.8852591790204,33.8234449888006,35.0304657090004));
#35847=CARTESIAN_POINT('Origin',(54.9397894030341,37.9543320991532,8.12867690713751));
#35848=CARTESIAN_POINT('',(48.0654635385539,33.5300503598268,35.0304657090004));
#35849=CARTESIAN_POINT('',(48.2454381951617,33.2621804705657,35.0304657090004));
#35850=CARTESIAN_POINT('Origin',(54.9397894030341,37.9543320991532,8.12867690713751));
#35851=CARTESIAN_POINT('',(48.4489573255588,32.984450416254,35.0304657090004));
#35852=CARTESIAN_POINT('',(48.6501670141011,32.7321414472684,35.0304657090004));
#35853=CARTESIAN_POINT('Origin',(54.9397894030341,37.9543320991532,8.12867690713751));
#35854=CARTESIAN_POINT('',(48.8756465291274,32.4719242153081,35.0304657090004));
#35855=CARTESIAN_POINT('',(49.0967522323243,32.2368552411587,35.0304657090004));
#35856=CARTESIAN_POINT('Origin',(54.9397894030341,37.9543320991532,8.12867690713751));
#35857=CARTESIAN_POINT('',(49.3426916030088,31.9958825342957,35.0304657090004));
#35858=CARTESIAN_POINT('',(49.5822218988852,31.7796179002216,35.0304657090004));
#35859=CARTESIAN_POINT('Origin',(54.9397894030341,37.9543320991532,8.12867690713751));
#35860=CARTESIAN_POINT('',(49.8469844392931,31.5594933520623,35.0304657090004));
#35861=CARTESIAN_POINT('',(50.1033452932499,31.3634722635223,35.0304657090004));
#35862=CARTESIAN_POINT('Origin',(54.9397894030341,37.9543320991532,8.12867690713751));
#35863=CARTESIAN_POINT('',(50.3851690523575,31.1656607666167,35.0304657090004));
#35864=CARTESIAN_POINT('',(50.656654425208,30.9911877116138,35.0304657090004));
#35865=CARTESIAN_POINT('Origin',(54.9397894030341,37.9543320991532,8.12867690713751));
#35866=CARTESIAN_POINT('',(50.9536639123962,30.8170056688373,35.0304657090004));
#35867=CARTESIAN_POINT('',(51.2384671137761,30.6652417367663,35.0304657090004));
#35868=CARTESIAN_POINT('Origin',(54.9397894030341,37.9543320991532,8.12867690713751));
#35869=CARTESIAN_POINT('',(51.5486857799107,30.5158483008756,35.0304657090004));
#35870=CARTESIAN_POINT('',(51.844911491504,30.3878034556653,35.0304657090004));
#35871=CARTESIAN_POINT('Origin',(54.9397894030341,37.9543320991532,8.12867690713751));
#35872=CARTESIAN_POINT('',(52.1662748825443,30.264192815328,35.0304657090004));
#35873=CARTESIAN_POINT('',(52.4719517711141,30.1607191742974,35.0304657090004));
#35874=CARTESIAN_POINT('Origin',(54.9397894030341,37.9543320991532,8.12867690713751));
#35875=CARTESIAN_POINT('',(52.8023212667141,30.0637139379306,35.0304657090004));
#35876=CARTESIAN_POINT('',(53.1154151030002,29.9855001010888,35.0304657090004));
#35877=CARTESIAN_POINT('Origin',(54.9397894030341,37.9543320991532,8.12867690713751));
#35878=CARTESIAN_POINT('',(53.4525921486737,29.9157458225357,35.0304657090004));
#35879=CARTESIAN_POINT('',(53.7710193448524,29.8633122900625,35.0304657090004));
#35880=CARTESIAN_POINT('Origin',(54.9397894030341,37.9543320991532,8.12867690713751));
#35881=CARTESIAN_POINT('',(54.1127600829908,29.8212731725384,35.0304657090004));
#35882=CARTESIAN_POINT('',(54.4344015586084,29.7949688809415,35.0304657090004));
#35883=CARTESIAN_POINT('Origin',(54.9397894030341,37.9543320991532,8.12867690713751));
#35884=CARTESIAN_POINT('',(54.7784317609826,29.7809246878375,35.0304657090004));
#35885=CARTESIAN_POINT('',(55.1011470450858,29.7809246878375,35.0304657090004));
#35886=CARTESIAN_POINT('Origin',(54.9397894030341,37.9543320991532,8.12867690713751));
#35887=CARTESIAN_POINT('',(55.44517724746,29.7949688809415,35.0304657090004));
#35888=CARTESIAN_POINT('',(55.7668187230776,29.8212731725384,35.0304657090004));
#35889=CARTESIAN_POINT('Origin',(54.9397894030341,37.9543320991532,8.12867690713751));
#35890=CARTESIAN_POINT('',(56.108559461216,29.8633122900625,35.0304657090004));
#35891=CARTESIAN_POINT('',(56.4269866573947,29.9157458225358,35.0304657090004));
#35892=CARTESIAN_POINT('Origin',(54.9397894030341,37.9543320991532,8.12867690713751));
#35893=CARTESIAN_POINT('',(56.7641637030682,29.9855001010888,35.0304657090004));
#35894=CARTESIAN_POINT('',(57.0772575393543,30.0637139379306,35.0304657090004));
#35895=CARTESIAN_POINT('Origin',(54.9397894030341,37.9543320991532,8.12867690713751));
#35896=CARTESIAN_POINT('',(57.4076270349543,30.1607191742974,35.0304657090004));
#35897=CARTESIAN_POINT('',(57.7133039235241,30.264192815328,35.0304657090004));
#35898=CARTESIAN_POINT('Origin',(54.9397894030341,37.9543320991532,8.12867690713751));
#35899=CARTESIAN_POINT('',(58.0346673145645,30.3878034556654,35.0304657090004));
#35900=CARTESIAN_POINT('',(58.3308930261577,30.5158483008756,35.0304657090004));
#35901=CARTESIAN_POINT('Origin',(54.9397894030341,37.9543320991532,8.12867690713751));
#35902=CARTESIAN_POINT('',(58.6411116922923,30.6652417367664,35.0304657090004));
#35903=CARTESIAN_POINT('',(58.9259148936722,30.8170056688373,35.0304657090004));
#35904=CARTESIAN_POINT('Origin',(54.9397894030341,37.9543320991532,8.12867690713751));
#35905=CARTESIAN_POINT('',(59.2229243808604,30.9911877116138,35.0304657090004));
#35906=CARTESIAN_POINT('',(59.4944097537108,31.1656607666168,35.0304657090004));
#35907=CARTESIAN_POINT('Origin',(54.9397894030341,37.9543320991532,8.12867690713751));
#35908=CARTESIAN_POINT('',(59.7762335128185,31.3634722635224,35.0304657090004));
#35909=CARTESIAN_POINT('',(60.0325943667752,31.5594933520624,35.0304657090004));
#35910=CARTESIAN_POINT('Origin',(54.9397894030341,37.9543320991532,8.12867690713751));
#35911=CARTESIAN_POINT('',(60.2973569071831,31.7796179002217,35.0304657090004));
#35912=CARTESIAN_POINT('',(60.5368872030596,31.9958825342957,35.0304657090004));
#35913=CARTESIAN_POINT('Origin',(54.9397894030341,37.9543320991532,8.12867690713751));
#35914=CARTESIAN_POINT('',(60.7828265737441,32.2368552411588,35.0304657090004));
#35915=CARTESIAN_POINT('',(61.0039322769409,32.4719242153082,35.0304657090004));
#35916=CARTESIAN_POINT('Origin',(54.9397894030341,37.9543320991532,8.12867690713751));
#35917=CARTESIAN_POINT('',(61.2294117919672,32.7321414472685,35.0304657090004));
#35918=CARTESIAN_POINT('',(61.4306214805095,32.9844504162541,35.0304657090004));
#35919=CARTESIAN_POINT('Origin',(54.9397894030341,37.9543320991532,8.12867690713751));
#35920=CARTESIAN_POINT('',(61.6341406109067,33.2621804705658,35.0304657090004));
#35921=CARTESIAN_POINT('',(61.8141152675145,33.5300503598269,35.0304657090004));
#35922=CARTESIAN_POINT('Origin',(54.9397894030341,37.9543320991532,8.12867690713751));
#35923=CARTESIAN_POINT('',(61.9943196270479,33.8234449888007,35.0304657090004));
#35924=CARTESIAN_POINT('',(62.1518615500752,34.1050931684198,35.0304657090004));
#35925=CARTESIAN_POINT('Origin',(54.9397894030341,37.9543320991532,8.12867690713751));
#35926=CARTESIAN_POINT('',(62.3075519084639,34.4121998792067,35.0304657090004));
#35927=CARTESIAN_POINT('',(62.4416126824056,34.705752027017,35.0304657090004));
#35928=CARTESIAN_POINT('Origin',(54.9397894030341,37.9543320991532,8.12867690713751));
#35929=CARTESIAN_POINT('',(62.5717529460015,35.0245270751257,35.0304657090004));
#35930=CARTESIAN_POINT('',(62.6814404185254,35.3280296500162,35.0304657090004));
#35931=CARTESIAN_POINT('Origin',(54.9397894030341,37.9543320991532,8.12867690713751));
#35932=CARTESIAN_POINT('',(62.785164525346,35.6563516400959,35.0304657090004));
#35933=CARTESIAN_POINT('',(62.8697487444197,35.9677848825051,35.0304657090004));
#35934=CARTESIAN_POINT('Origin',(54.9397894030341,37.9543320991532,8.12867690713751));
#35935=CARTESIAN_POINT('',(62.9463664276474,36.3034688858809,35.0304657090004));
#35936=CARTESIAN_POINT('',(63.0052844992482,36.6207602589636,35.0304657090004));
#35937=CARTESIAN_POINT('Origin',(54.9397894030341,37.9543320991532,8.12867690713751));
#35938=CARTESIAN_POINT('',(63.0542858808421,36.9615723539771,35.0304657090004));
#35939=CARTESIAN_POINT('',(63.0871457149245,37.2826103359947,35.0304657090004));
#35940=CARTESIAN_POINT('Origin',(54.9397894030341,37.9543320991532,8.12867690713751));
#35941=CARTESIAN_POINT('',(63.1082046987747,37.6262824743835,35.0304657090004));
#35942=CARTESIAN_POINT('',(63.1147876185643,37.9489306105332,35.0304657090004));
#35943=CARTESIAN_POINT('Origin',(54.9397894030341,37.9543320991532,8.12867690713751));
#35944=CARTESIAN_POINT('',(63.1077640606078,38.2931757109184,35.0304657090004));
#35945=CARTESIAN_POINT('',(63.0880262578595,38.6152868310874,35.0304657090004));
#35946=CARTESIAN_POINT('Origin',(54.9397894030341,37.9543320991532,8.12867690713751));
#35947=CARTESIAN_POINT('',(63.0529668987158,38.9578139991223,35.0304657090004));
#35948=CARTESIAN_POINT('',(63.0070397252503,39.2772445069504,35.0304657090004));
#35949=CARTESIAN_POINT('Origin',(54.9397894030341,37.9543320991532,8.12867690713751));
#35950=CARTESIAN_POINT('',(62.94417787917,39.6157742808448,35.0304657090004));
#35951=CARTESIAN_POINT('',(62.8723669727493,39.9303984190047,35.0304657090004));
#35952=CARTESIAN_POINT('Origin',(54.9397894030341,37.9543320991532,8.12867690713751));
#35953=CARTESIAN_POINT('',(62.7821209749467,40.2626779389667,35.0304657090004));
#35954=CARTESIAN_POINT('',(62.6849042253051,40.5704019357284,35.0304657090004));
#35955=CARTESIAN_POINT('Origin',(54.9397894030341,37.9543320991532,8.12867690713751));
#35956=CARTESIAN_POINT('',(62.5678746480059,40.894219936375,35.0304657090004));
#35957=CARTESIAN_POINT('',(62.4458990165727,41.1929959393108,35.0304657090004));
#35958=CARTESIAN_POINT('Origin',(54.9397894030341,37.9543320991532,8.12867690713751));
#35959=CARTESIAN_POINT('',(62.3028646723053,41.5061974652739,35.0304657090004));
#35960=CARTESIAN_POINT('',(62.1569418867831,41.7940371693789,35.0304657090004));
#35961=CARTESIAN_POINT('Origin',(54.9397894030341,37.9543320991532,8.12867690713751));
#35962=CARTESIAN_POINT('',(61.9888546455096,42.0945379161778,35.0304657090004));
#35963=CARTESIAN_POINT('',(61.8199557979604,42.3695257957114,35.0304657090004));
#35964=CARTESIAN_POINT('Origin',(54.9397894030341,37.9543320991532,8.12867690713751));
#35965=CARTESIAN_POINT('',(61.6279342525392,42.6553259804552,35.0304657090004));
#35966=CARTESIAN_POINT('',(61.4371833369271,42.915632036449,35.0304657090004));
#35967=CARTESIAN_POINT('Origin',(54.9397894030341,37.9543320991532,8.12867690713751));
#35968=CARTESIAN_POINT('',(61.2225053590615,43.184829706062,35.0304657090004));
#35969=CARTESIAN_POINT('',(61.0111717912583,43.4287216446607,35.0304657090004));
#35970=CARTESIAN_POINT('Origin',(54.9397894030341,37.9543320991532,8.12867690713751));
#35971=CARTESIAN_POINT('',(60.7752660274717,43.6795253330662,35.0304657090004));
#35972=CARTESIAN_POINT('',(60.5447561975034,43.9053800936578,35.0304657090004));
#35973=CARTESIAN_POINT('Origin',(54.9397894030341,37.9543320991532,8.12867690713751));
#35974=CARTESIAN_POINT('',(60.289192561732,44.1361207436891,35.0304657090004));
#35975=CARTESIAN_POINT('',(60.0410404744858,44.3424353001052,35.0304657090004));
#35976=CARTESIAN_POINT('Origin',(54.9397894030341,37.9543320991532,8.12867690713751));
#35977=CARTESIAN_POINT('',(59.7675197005607,44.551577370806,35.0304657090004));
#35978=CARTESIAN_POINT('',(59.5033767672348,44.7369787337132,35.0304657090004));
#35979=CARTESIAN_POINT('Origin',(54.9397894030341,37.9543320991532,8.12867690713751));
#35980=CARTESIAN_POINT('',(59.2137190907787,44.9231304191088,35.0304657090004));
#35981=CARTESIAN_POINT('',(58.935343139014,45.0863847730261,35.0304657090004));
#35982=CARTESIAN_POINT('Origin',(54.9397894030341,37.9543320991532,8.12867690713751));
#35983=CARTESIAN_POINT('',(58.6314761840736,45.2483072643631,35.0304657090004));
#35984=CARTESIAN_POINT('',(58.3407197599002,45.3883281785002,35.0304657090004));
#35985=CARTESIAN_POINT('Origin',(54.9397894030341,37.9543320991532,8.12867690713751));
#35986=CARTESIAN_POINT('',(58.024665710926,45.5249439083142,35.0304657090004));
#35987=CARTESIAN_POINT('',(57.7234637503755,45.6407995665893,35.0304657090004));
#35988=CARTESIAN_POINT('Origin',(54.9397894030341,37.9543320991532,8.12867690713751));
#35989=CARTESIAN_POINT('',(57.3973258949183,45.7511993797383,35.0304657090004));
#35990=CARTESIAN_POINT('',(57.0876828473432,45.8421187818605,35.0304657090004));
#35991=CARTESIAN_POINT('Origin',(54.9397894030341,37.9543320991532,8.12867690713751));
#35992=CARTESIAN_POINT('',(56.753631579022,45.9255679858027,35.0304657090004));
#35993=CARTESIAN_POINT('',(56.4376080678165,45.9909460781515,35.0304657090004));
#35994=CARTESIAN_POINT('Origin',(54.9397894030341,37.9543320991532,8.12867690713751));
#35995=CARTESIAN_POINT('',(56.0978664427074,46.0468893322027,35.0304657090004));
#35996=CARTESIAN_POINT('',(55.7775655521983,46.0862910343602,35.0304657090004));
#35997=CARTESIAN_POINT('Origin',(54.9397894030341,37.9543320991532,8.12867690713751));
#35998=CARTESIAN_POINT('',(54.4451843113051,46.1143560453948,35.0304657090004));
#35999=CARTESIAN_POINT('',(54.7676310315374,46.1275191455338,35.0304657090004));
#36000=CARTESIAN_POINT('Origin',(54.9397894030341,39.9543320991532,23.0294657090004));
#36001=CARTESIAN_POINT('Origin',(54.9397894030341,37.9543320991532,8.12867690713751));
#36002=CARTESIAN_POINT('',(55.4343944947631,46.1143560453948,35.0304657090004));
#36003=CARTESIAN_POINT('',(55.1119477745308,46.1275191455338,35.0304657090004));
#36004=CARTESIAN_POINT('Origin',(54.9397894030341,37.9543320991532,19.5294657090004));
#36005=CARTESIAN_POINT('Origin',(54.9397894030341,39.5643320991532,35.0294657090004));
#36006=CARTESIAN_POINT('Origin',(54.9397894030341,45.8293320991532,35.0304657090004));
#36007=CARTESIAN_POINT('',(54.9397894030341,45.8293320991532,35.0304657090004));
#36008=CARTESIAN_POINT('Origin',(54.9397894030341,45.8293320991532,35.0304657090004));
#36009=CARTESIAN_POINT('Origin',(54.297903795101,45.803128686295,35.0304657090004));
#36010=CARTESIAN_POINT('',(54.297903795101,45.803128686295,35.0304657090004));
#36011=CARTESIAN_POINT('Origin',(54.297903795101,45.803128686295,35.0304657090004));
#36012=CARTESIAN_POINT('Origin',(55.5816750109672,45.803128686295,35.0304657090004));
#36013=CARTESIAN_POINT('',(55.5816750109672,45.803128686295,35.0304657090004));
#36014=CARTESIAN_POINT('Origin',(55.5816750109672,45.803128686295,35.0304657090004));
#36015=CARTESIAN_POINT('Origin',(56.2192889760832,45.7246928271096,35.0304657090004));
#36016=CARTESIAN_POINT('',(56.2192889760832,45.7246928271096,35.0304657090004));
#36017=CARTESIAN_POINT('Origin',(56.2192889760832,45.7246928271096,35.0304657090004));
#36018=CARTESIAN_POINT('Origin',(56.8483880826431,45.594546499299,35.0304657090004));
#36019=CARTESIAN_POINT('',(56.8483880826431,45.594546499299,35.0304657090004));
#36020=CARTESIAN_POINT('Origin',(56.8483880826431,45.594546499299,35.0304657090004));
#36021=CARTESIAN_POINT('Origin',(57.4647857798868,45.413555805202,35.0304657090004));
#36022=CARTESIAN_POINT('',(57.4647857798868,45.413555805202,35.0304657090004));
#36023=CARTESIAN_POINT('Origin',(57.4647857798868,45.413555805202,35.0304657090004));
#36024=CARTESIAN_POINT('Origin',(58.0643800428377,45.1829252080266,35.0304657090004));
#36025=CARTESIAN_POINT('',(58.0643800428377,45.1829252080266,35.0304657090004));
#36026=CARTESIAN_POINT('Origin',(58.0643800428377,45.1829252080266,35.0304657090004));
#36027=CARTESIAN_POINT('Origin',(58.6431806706019,44.9041895163456,35.0304657090004));
#36028=CARTESIAN_POINT('',(58.6431806706019,44.9041895163456,35.0304657090004));
#36029=CARTESIAN_POINT('Origin',(58.6431806706019,44.9041895163456,35.0304657090004));
#36030=CARTESIAN_POINT('Origin',(59.1973358404969,44.5792036701988,35.0304657090004));
#36031=CARTESIAN_POINT('',(59.1973358404969,44.5792036701988,35.0304657090004));
#36032=CARTESIAN_POINT('Origin',(59.1973358404969,44.5792036701988,35.0304657090004));
#36033=CARTESIAN_POINT('Origin',(59.7231577412963,44.2101303967737,35.0304657090004));
#36034=CARTESIAN_POINT('',(59.7231577412963,44.2101303967737,35.0304657090004));
#36035=CARTESIAN_POINT('Origin',(59.7231577412963,44.2101303967737,35.0304657090004));
#36036=CARTESIAN_POINT('Origin',(60.2171471150049,43.7994258178119,35.0304657090004));
#36037=CARTESIAN_POINT('',(60.2171471150049,43.7994258178119,35.0304657090004));
#36038=CARTESIAN_POINT('Origin',(60.2171471150049,43.7994258178119,35.0304657090004));
#36039=CARTESIAN_POINT('Origin',(60.6760165438429,43.3498231045251,35.0304657090004));
#36040=CARTESIAN_POINT('',(60.6760165438429,43.3498231045251,35.0304657090004));
#36041=CARTESIAN_POINT('Origin',(60.6760165438429,43.3498231045251,35.0304657090004));
#36042=CARTESIAN_POINT('Origin',(61.0967123274698,42.8643142887908,35.0304657090004));
#36043=CARTESIAN_POINT('',(61.0967123274698,42.8643142887908,35.0304657090004));
#36044=CARTESIAN_POINT('Origin',(61.0967123274698,42.8643142887908,35.0304657090004));
#36045=CARTESIAN_POINT('Origin',(61.4764348048554,42.3461303516746,35.0304657090004));
#36046=CARTESIAN_POINT('',(61.4764348048554,42.3461303516746,35.0304657090004));
#36047=CARTESIAN_POINT('Origin',(61.4764348048554,42.3461303516746,35.0304657090004));
#36048=CARTESIAN_POINT('Origin',(61.8126569855623,41.7987197217835,35.0304657090004));
#36049=CARTESIAN_POINT('',(61.8126569855623,41.7987197217835,35.0304657090004));
#36050=CARTESIAN_POINT('Origin',(61.8126569855623,41.7987197217835,35.0304657090004));
#36051=CARTESIAN_POINT('Origin',(62.1031413664509,41.2257253265432,35.0304657090004));
#36052=CARTESIAN_POINT('',(62.1031413664509,41.2257253265432,35.0304657090004));
#36053=CARTESIAN_POINT('Origin',(62.1031413664509,41.2257253265432,35.0304657090004));
#36054=CARTESIAN_POINT('Origin',(62.3459548218929,40.6309603491164,35.0304657090004));
#36055=CARTESIAN_POINT('',(62.3459548218929,40.6309603491164,35.0304657090004));
#36056=CARTESIAN_POINT('Origin',(62.3459548218929,40.6309603491164,35.0304657090004));
#36057=CARTESIAN_POINT('Origin',(62.5394814684036,40.0183828522987,35.0304657090004));
#36058=CARTESIAN_POINT('',(62.5394814684036,40.0183828522987,35.0304657090004));
#36059=CARTESIAN_POINT('Origin',(62.5394814684036,40.0183828522987,35.0304657090004));
#36060=CARTESIAN_POINT('Origin',(62.6824334180802,39.3920694382633,35.0304657090004));
#36061=CARTESIAN_POINT('',(62.6824334180802,39.3920694382633,35.0304657090004));
#36062=CARTESIAN_POINT('Origin',(62.6824334180802,39.3920694382633,35.0304657090004));
#36063=CARTESIAN_POINT('Origin',(62.773859349283,38.756188119446,35.0304657090004));
#36064=CARTESIAN_POINT('',(62.773859349283,38.756188119446,35.0304657090004));
#36065=CARTESIAN_POINT('Origin',(62.773859349283,38.756188119446,35.0304657090004));
#36066=CARTESIAN_POINT('Origin',(62.8131508375241,38.1149705811106,35.0304657090004));
#36067=CARTESIAN_POINT('',(62.8131508375241,38.1149705811106,35.0304657090004));
#36068=CARTESIAN_POINT('Origin',(62.8131508375241,38.1149705811106,35.0304657090004));
#36069=CARTESIAN_POINT('Origin',(62.8000464044319,37.4726840201813,35.0304657090004));
#36070=CARTESIAN_POINT('',(62.8000464044319,37.4726840201813,35.0304657090004));
#36071=CARTESIAN_POINT('Origin',(62.8000464044319,37.4726840201813,35.0304657090004));
#36072=CARTESIAN_POINT('Origin',(62.7346332578465,36.8336027477512,35.0304657090004));
#36073=CARTESIAN_POINT('',(62.7346332578465,36.8336027477512,35.0304657090004));
#36074=CARTESIAN_POINT('Origin',(62.7346332578465,36.8336027477512,35.0304657090004));
#36075=CARTESIAN_POINT('Origin',(62.617346711466,36.2019797442473,35.0304657090004));
#36076=CARTESIAN_POINT('',(62.617346711466,36.2019797442473,35.0304657090004));
#36077=CARTESIAN_POINT('Origin',(62.617346711466,36.2019797442473,35.0304657090004));
#36078=CARTESIAN_POINT('Origin',(62.4489672879057,35.5820183565476,35.0304657090004));
#36079=CARTESIAN_POINT('',(62.4489672879057,35.5820183565476,35.0304657090004));
#36080=CARTESIAN_POINT('Origin',(62.4489672879057,35.5820183565476,35.0304657090004));
#36081=CARTESIAN_POINT('Origin',(62.2306155244487,34.9778443254007,35.0304657090004));
#36082=CARTESIAN_POINT('',(62.2306155244487,34.9778443254007,35.0304657090004));
#36083=CARTESIAN_POINT('Origin',(62.2306155244487,34.9778443254007,35.0304657090004));
#36084=CARTESIAN_POINT('Origin',(61.9637445160554,34.3934783293021,35.0304657090004));
#36085=CARTESIAN_POINT('',(61.9637445160554,34.3934783293021,35.0304657090004));
#36086=CARTESIAN_POINT('Origin',(61.9637445160554,34.3934783293021,35.0304657090004));
#36087=CARTESIAN_POINT('Origin',(61.6501302452559,33.8328092275425,35.0304657090004));
#36088=CARTESIAN_POINT('',(61.6501302452559,33.8328092275425,35.0304657090004));
#36089=CARTESIAN_POINT('Origin',(61.6501302452559,33.8328092275425,35.0304657090004));
#36090=CARTESIAN_POINT('Origin',(61.2918597632797,33.2995681804899,35.0304657090004));
#36091=CARTESIAN_POINT('',(61.2918597632797,33.2995681804899,35.0304657090004));
#36092=CARTESIAN_POINT('Origin',(61.2918597632797,33.2995681804899,35.0304657090004));
#36093=CARTESIAN_POINT('Origin',(60.891317301074,32.7973038193341,35.0304657090004));
#36094=CARTESIAN_POINT('',(60.891317301074,32.7973038193341,35.0304657090004));
#36095=CARTESIAN_POINT('Origin',(60.891317301074,32.7973038193341,35.0304657090004));
#36096=CARTESIAN_POINT('Origin',(60.4511684026397,32.3293586305308,35.0304657090004));
#36097=CARTESIAN_POINT('',(60.4511684026397,32.3293586305308,35.0304657090004));
#36098=CARTESIAN_POINT('Origin',(60.4511684026397,32.3293586305308,35.0304657090004));
#36099=CARTESIAN_POINT('Origin',(59.9743421862767,31.8988467121058,35.0304657090004));
#36100=CARTESIAN_POINT('',(59.9743421862767,31.8988467121058,35.0304657090004));
#36101=CARTESIAN_POINT('Origin',(59.9743421862767,31.8988467121058,35.0304657090004));
#36102=CARTESIAN_POINT('Origin',(59.4640118517838,31.5086330498468,35.0304657090004));
#36103=CARTESIAN_POINT('',(59.4640118517838,31.5086330498468,35.0304657090004));
#36104=CARTESIAN_POINT('Origin',(59.4640118517838,31.5086330498468,35.0304657090004));
#36105=CARTESIAN_POINT('Origin',(58.9235735633388,31.1613144512955,35.0304657090004));
#36106=CARTESIAN_POINT('',(58.9235735633388,31.1613144512955,35.0304657090004));
#36107=CARTESIAN_POINT('Origin',(58.9235735633388,31.1613144512955,35.0304657090004));
#36108=CARTESIAN_POINT('Origin',(58.356623848585,30.8592022644217,35.0304657090004));
#36109=CARTESIAN_POINT('',(58.356623848585,30.8592022644217,35.0304657090004));
#36110=CARTESIAN_POINT('Origin',(58.356623848585,30.8592022644217,35.0304657090004));
#36111=CARTESIAN_POINT('Origin',(57.766935664334,30.604306995984,35.0304657090004));
#36112=CARTESIAN_POINT('',(57.766935664334,30.604306995984,35.0304657090004));
#36113=CARTESIAN_POINT('Origin',(57.766935664334,30.604306995984,35.0304657090004));
#36114=CARTESIAN_POINT('Origin',(57.1584332881605,30.3983249319391,35.0304657090004));
#36115=CARTESIAN_POINT('',(57.1584332881605,30.3983249319391,35.0304657090004));
#36116=CARTESIAN_POINT('Origin',(57.1584332881605,30.3983249319391,35.0304657090004));
#36117=CARTESIAN_POINT('Origin',(56.5351662029818,30.2426268489385,35.0304657090004));
#36118=CARTESIAN_POINT('',(56.5351662029818,30.2426268489385,35.0304657090004));
#36119=CARTESIAN_POINT('Origin',(56.5351662029818,30.2426268489385,35.0304657090004));
#36120=CARTESIAN_POINT('Origin',(55.9012821484182,30.1382488920364,35.0304657090004));
#36121=CARTESIAN_POINT('',(55.9012821484182,30.1382488920364,35.0304657090004));
#36122=CARTESIAN_POINT('Origin',(55.9012821484182,30.1382488920364,35.0304657090004));
#36123=CARTESIAN_POINT('Origin',(55.2609995182692,30.0858856793146,35.0304657090004));
#36124=CARTESIAN_POINT('',(55.2609995182692,30.0858856793146,35.0304657090004));
#36125=CARTESIAN_POINT('Origin',(55.2609995182692,30.0858856793146,35.0304657090004));
#36126=CARTESIAN_POINT('Origin',(54.6185792877992,30.0858856793146,35.0304657090004));
#36127=CARTESIAN_POINT('',(54.6185792877992,30.0858856793146,35.0304657090004));
#36128=CARTESIAN_POINT('Origin',(54.6185792877992,30.0858856793146,35.0304657090004));
#36129=CARTESIAN_POINT('Origin',(53.9782966576502,30.1382488920364,35.0304657090004));
#36130=CARTESIAN_POINT('',(53.9782966576502,30.1382488920364,35.0304657090004));
#36131=CARTESIAN_POINT('Origin',(53.9782966576502,30.1382488920364,35.0304657090004));
#36132=CARTESIAN_POINT('Origin',(53.3444126030866,30.2426268489385,35.0304657090004));
#36133=CARTESIAN_POINT('',(53.3444126030866,30.2426268489385,35.0304657090004));
#36134=CARTESIAN_POINT('Origin',(53.3444126030866,30.2426268489385,35.0304657090004));
#36135=CARTESIAN_POINT('Origin',(52.7211455179079,30.398324931939,35.0304657090004));
#36136=CARTESIAN_POINT('',(52.7211455179079,30.398324931939,35.0304657090004));
#36137=CARTESIAN_POINT('Origin',(52.7211455179079,30.398324931939,35.0304657090004));
#36138=CARTESIAN_POINT('Origin',(52.1126431417343,30.6043069959839,35.0304657090004));
#36139=CARTESIAN_POINT('',(52.1126431417343,30.6043069959839,35.0304657090004));
#36140=CARTESIAN_POINT('Origin',(52.1126431417343,30.6043069959839,35.0304657090004));
#36141=CARTESIAN_POINT('Origin',(51.5229549574834,30.8592022644217,35.0304657090004));
#36142=CARTESIAN_POINT('',(51.5229549574834,30.8592022644217,35.0304657090004));
#36143=CARTESIAN_POINT('Origin',(51.5229549574834,30.8592022644217,35.0304657090004));
#36144=CARTESIAN_POINT('Origin',(50.9560052427296,31.1613144512955,35.0304657090004));
#36145=CARTESIAN_POINT('',(50.9560052427296,31.1613144512955,35.0304657090004));
#36146=CARTESIAN_POINT('Origin',(50.9560052427296,31.1613144512955,35.0304657090004));
#36147=CARTESIAN_POINT('Origin',(50.4155669542845,31.5086330498468,35.0304657090004));
#36148=CARTESIAN_POINT('',(50.4155669542845,31.5086330498468,35.0304657090004));
#36149=CARTESIAN_POINT('Origin',(50.4155669542845,31.5086330498468,35.0304657090004));
#36150=CARTESIAN_POINT('Origin',(49.9052366197917,31.8988467121057,35.0304657090004));
#36151=CARTESIAN_POINT('',(49.9052366197917,31.8988467121057,35.0304657090004));
#36152=CARTESIAN_POINT('Origin',(49.9052366197917,31.8988467121057,35.0304657090004));
#36153=CARTESIAN_POINT('Origin',(49.4284104034286,32.3293586305307,35.0304657090004));
#36154=CARTESIAN_POINT('',(49.4284104034286,32.3293586305307,35.0304657090004));
#36155=CARTESIAN_POINT('Origin',(49.4284104034286,32.3293586305307,35.0304657090004));
#36156=CARTESIAN_POINT('Origin',(48.9882615049944,32.7973038193341,35.0304657090004));
#36157=CARTESIAN_POINT('',(48.9882615049944,32.7973038193341,35.0304657090004));
#36158=CARTESIAN_POINT('Origin',(48.9882615049944,32.7973038193341,35.0304657090004));
#36159=CARTESIAN_POINT('Origin',(48.5877190427886,33.2995681804899,35.0304657090004));
#36160=CARTESIAN_POINT('',(48.5877190427886,33.2995681804899,35.0304657090004));
#36161=CARTESIAN_POINT('Origin',(48.5877190427886,33.2995681804899,35.0304657090004));
#36162=CARTESIAN_POINT('Origin',(48.2294485608124,33.8328092275424,35.0304657090004));
#36163=CARTESIAN_POINT('',(48.2294485608124,33.8328092275424,35.0304657090004));
#36164=CARTESIAN_POINT('Origin',(48.2294485608124,33.8328092275424,35.0304657090004));
#36165=CARTESIAN_POINT('Origin',(47.9158342900129,34.393478329302,35.0304657090004));
#36166=CARTESIAN_POINT('',(47.9158342900129,34.393478329302,35.0304657090004));
#36167=CARTESIAN_POINT('Origin',(47.9158342900129,34.393478329302,35.0304657090004));
#36168=CARTESIAN_POINT('Origin',(47.6489632816196,34.9778443254006,35.0304657090004));
#36169=CARTESIAN_POINT('',(47.6489632816196,34.9778443254006,35.0304657090004));
#36170=CARTESIAN_POINT('Origin',(47.6489632816196,34.9778443254006,35.0304657090004));
#36171=CARTESIAN_POINT('Origin',(47.4306115181626,35.5820183565475,35.0304657090004));
#36172=CARTESIAN_POINT('',(47.4306115181626,35.5820183565475,35.0304657090004));
#36173=CARTESIAN_POINT('Origin',(47.4306115181626,35.5820183565475,35.0304657090004));
#36174=CARTESIAN_POINT('Origin',(47.2622320946023,36.2019797442472,35.0304657090004));
#36175=CARTESIAN_POINT('',(47.2622320946023,36.2019797442472,35.0304657090004));
#36176=CARTESIAN_POINT('Origin',(47.2622320946023,36.2019797442472,35.0304657090004));
#36177=CARTESIAN_POINT('Origin',(47.1449455482218,36.8336027477511,35.0304657090004));
#36178=CARTESIAN_POINT('',(47.1449455482218,36.8336027477511,35.0304657090004));
#36179=CARTESIAN_POINT('Origin',(47.1449455482218,36.8336027477511,35.0304657090004));
#36180=CARTESIAN_POINT('Origin',(47.0795324016364,37.4726840201812,35.0304657090004));
#36181=CARTESIAN_POINT('',(47.0795324016364,37.4726840201812,35.0304657090004));
#36182=CARTESIAN_POINT('Origin',(47.0795324016364,37.4726840201812,35.0304657090004));
#36183=CARTESIAN_POINT('Origin',(47.0664279685441,38.1149705811105,35.0304657090004));
#36184=CARTESIAN_POINT('',(47.0664279685441,38.1149705811105,35.0304657090004));
#36185=CARTESIAN_POINT('Origin',(47.0664279685441,38.1149705811105,35.0304657090004));
#36186=CARTESIAN_POINT('Origin',(47.1057194567852,38.7561881194459,35.0304657090004));
#36187=CARTESIAN_POINT('',(47.1057194567852,38.7561881194459,35.0304657090004));
#36188=CARTESIAN_POINT('Origin',(47.1057194567852,38.7561881194459,35.0304657090004));
#36189=CARTESIAN_POINT('Origin',(47.197145387988,39.3920694382632,35.0304657090004));
#36190=CARTESIAN_POINT('',(47.197145387988,39.3920694382632,35.0304657090004));
#36191=CARTESIAN_POINT('Origin',(47.197145387988,39.3920694382632,35.0304657090004));
#36192=CARTESIAN_POINT('Origin',(47.3400973376647,40.0183828522986,35.0304657090004));
#36193=CARTESIAN_POINT('',(47.3400973376647,40.0183828522986,35.0304657090004));
#36194=CARTESIAN_POINT('Origin',(47.3400973376647,40.0183828522986,35.0304657090004));
#36195=CARTESIAN_POINT('Origin',(47.5336239841754,40.6309603491163,35.0304657090004));
#36196=CARTESIAN_POINT('',(47.5336239841754,40.6309603491163,35.0304657090004));
#36197=CARTESIAN_POINT('Origin',(47.5336239841754,40.6309603491163,35.0304657090004));
#36198=CARTESIAN_POINT('Origin',(47.7764374396173,41.2257253265431,35.0304657090004));
#36199=CARTESIAN_POINT('',(47.7764374396173,41.2257253265431,35.0304657090004));
#36200=CARTESIAN_POINT('Origin',(47.7764374396173,41.2257253265431,35.0304657090004));
#36201=CARTESIAN_POINT('Origin',(48.0669218205059,41.7987197217834,35.0304657090004));
#36202=CARTESIAN_POINT('',(48.0669218205059,41.7987197217834,35.0304657090004));
#36203=CARTESIAN_POINT('Origin',(48.0669218205059,41.7987197217834,35.0304657090004));
#36204=CARTESIAN_POINT('Origin',(48.4031440012129,42.3461303516745,35.0304657090004));
#36205=CARTESIAN_POINT('',(48.4031440012129,42.3461303516745,35.0304657090004));
#36206=CARTESIAN_POINT('Origin',(48.4031440012129,42.3461303516745,35.0304657090004));
#36207=CARTESIAN_POINT('Origin',(48.7828664785984,42.8643142887907,35.0304657090004));
#36208=CARTESIAN_POINT('',(48.7828664785984,42.8643142887907,35.0304657090004));
#36209=CARTESIAN_POINT('Origin',(48.7828664785984,42.8643142887907,35.0304657090004));
#36210=CARTESIAN_POINT('Origin',(49.2035622622253,43.349823104525,35.0304657090004));
#36211=CARTESIAN_POINT('',(49.2035622622253,43.349823104525,35.0304657090004));
#36212=CARTESIAN_POINT('Origin',(49.2035622622253,43.349823104525,35.0304657090004));
#36213=CARTESIAN_POINT('Origin',(49.6624316910634,43.7994258178118,35.0304657090004));
#36214=CARTESIAN_POINT('',(49.6624316910634,43.7994258178118,35.0304657090004));
#36215=CARTESIAN_POINT('Origin',(49.6624316910634,43.7994258178118,35.0304657090004));
#36216=CARTESIAN_POINT('Origin',(50.1564210647719,44.2101303967736,35.0304657090004));
#36217=CARTESIAN_POINT('',(50.1564210647719,44.2101303967736,35.0304657090004));
#36218=CARTESIAN_POINT('Origin',(50.1564210647719,44.2101303967736,35.0304657090004));
#36219=CARTESIAN_POINT('Origin',(50.6822429655713,44.5792036701988,35.0304657090004));
#36220=CARTESIAN_POINT('',(50.6822429655713,44.5792036701988,35.0304657090004));
#36221=CARTESIAN_POINT('Origin',(50.6822429655713,44.5792036701988,35.0304657090004));
#36222=CARTESIAN_POINT('Origin',(51.2363981354663,44.9041895163455,35.0304657090004));
#36223=CARTESIAN_POINT('',(51.2363981354663,44.9041895163455,35.0304657090004));
#36224=CARTESIAN_POINT('Origin',(51.2363981354663,44.9041895163455,35.0304657090004));
#36225=CARTESIAN_POINT('Origin',(51.8151987632305,45.1829252080266,35.0304657090004));
#36226=CARTESIAN_POINT('',(51.8151987632305,45.1829252080266,35.0304657090004));
#36227=CARTESIAN_POINT('Origin',(51.8151987632305,45.1829252080266,35.0304657090004));
#36228=CARTESIAN_POINT('Origin',(52.4147930261813,45.413555805202,35.0304657090004));
#36229=CARTESIAN_POINT('',(52.4147930261813,45.413555805202,35.0304657090004));
#36230=CARTESIAN_POINT('Origin',(52.4147930261813,45.413555805202,35.0304657090004));
#36231=CARTESIAN_POINT('Origin',(53.0311907234251,45.594546499299,35.0304657090004));
#36232=CARTESIAN_POINT('',(53.0311907234251,45.594546499299,35.0304657090004));
#36233=CARTESIAN_POINT('Origin',(53.0311907234251,45.594546499299,35.0304657090004));
#36234=CARTESIAN_POINT('Origin',(53.660289829985,45.7246928271096,35.0304657090004));
#36235=CARTESIAN_POINT('',(53.660289829985,45.7246928271096,35.0304657090004));
#36236=CARTESIAN_POINT('Origin',(53.660289829985,45.7246928271096,35.0304657090004));
#36237=CARTESIAN_POINT('Origin',(43.4397894030341,37.9543320991532,41.9294657090004));
#36238=CARTESIAN_POINT('',(46.1052618504143,38.3543320991532,42.1294657090004));
#36239=CARTESIAN_POINT('',(46.1052618504143,37.5543320991532,42.1294657090004));
#36240=CARTESIAN_POINT('Origin',(43.4397894030341,37.9543320991532,42.1294657090004));
#36241=CARTESIAN_POINT('',(45.2130570344595,37.5543320991532,42.8294657090004));
#36242=CARTESIAN_POINT('Ctrl Pts',(45.2130570344595,37.5543320991532,42.8294657090004));
#36243=CARTESIAN_POINT('Ctrl Pts',(45.3272286490232,37.5543320991532,42.8294657090004));
#36244=CARTESIAN_POINT('Ctrl Pts',(45.461704750062,37.5543320991532,42.8032587413542));
#36245=CARTESIAN_POINT('Ctrl Pts',(45.6711920890012,37.5543320991532,42.717234203378));
#36246=CARTESIAN_POINT('Ctrl Pts',(45.783598159642,37.5543320991532,42.6429232657692));
#36247=CARTESIAN_POINT('Ctrl Pts',(45.9421647319298,37.5543320991532,42.4854573905017));
#36248=CARTESIAN_POINT('Ctrl Pts',(46.0166939687517,37.5543320991532,42.3748001680524));
#36249=CARTESIAN_POINT('Ctrl Pts',(46.0776692182323,37.5543320991532,42.2284287129193));
#36250=CARTESIAN_POINT('Ctrl Pts',(46.0936789385295,37.5543320991532,42.1797227805058));
#36251=CARTESIAN_POINT('Ctrl Pts',(46.1052618504143,37.5543320991532,42.1294657090004));
#36252=CARTESIAN_POINT('',(41.6665217716088,37.5543320991532,42.8294657090004));
#36253=CARTESIAN_POINT('Origin',(43.4397894030341,37.9543320991532,42.8294657090004));
#36254=CARTESIAN_POINT('',(40.7743169556539,37.5543320991532,42.1294657090004));
#36255=CARTESIAN_POINT('Ctrl Pts',(40.7743169556539,37.5543320991532,42.1294657090003));
#36256=CARTESIAN_POINT('Ctrl Pts',(40.7858998675388,37.5543320991532,42.1797227805058));
#36257=CARTESIAN_POINT('Ctrl Pts',(40.801909587836,37.5543320991532,42.2284287129193));
#36258=CARTESIAN_POINT('Ctrl Pts',(40.8628848373166,37.5543320991532,42.3748001680524));
#36259=CARTESIAN_POINT('Ctrl Pts',(40.9374140741385,37.5543320991532,42.4854573905017));
#36260=CARTESIAN_POINT('Ctrl Pts',(41.0959806464263,37.5543320991532,42.6429232657692));
#36261=CARTESIAN_POINT('Ctrl Pts',(41.2083867170671,37.5543320991532,42.717234203378));
#36262=CARTESIAN_POINT('Ctrl Pts',(41.4178740560063,37.5543320991532,42.8032587413542));
#36263=CARTESIAN_POINT('Ctrl Pts',(41.5523501570451,37.5543320991532,42.8294657090004));
#36264=CARTESIAN_POINT('Ctrl Pts',(41.6665217716088,37.5543320991532,42.8294657090004));
#36265=CARTESIAN_POINT('',(40.7444706152573,37.9543320991532,42.1294657090004));
#36266=CARTESIAN_POINT('Origin',(43.4397894030341,37.9543320991532,42.1294657090004));
#36267=CARTESIAN_POINT('',(40.7253918257139,37.9543320991532,42.0079058774732));
#36268=CARTESIAN_POINT('Origin',(41.6219670539965,37.9543320991532,41.9294657090004));
#36269=CARTESIAN_POINT('',(46.1541869803544,37.9543320991532,42.0079058774732));
#36270=CARTESIAN_POINT('Origin',(43.4397894030341,37.9543320991532,42.0079058774732));
#36271=CARTESIAN_POINT('Origin',(43.4397894030341,37.9543320991532,42.0079058774732));
#36272=CARTESIAN_POINT('',(40.7743169556539,38.3543320991532,42.1294657090004));
#36273=CARTESIAN_POINT('Origin',(43.4397894030341,37.9543320991532,42.1294657090004));
#36274=CARTESIAN_POINT('',(41.6665217716088,38.3543320991532,42.8294657090004));
#36275=CARTESIAN_POINT('Ctrl Pts',(41.6665217716088,38.3543320991532,42.8294657090004));
#36276=CARTESIAN_POINT('Ctrl Pts',(41.5523501570451,38.3543320991532,42.8294657090004));
#36277=CARTESIAN_POINT('Ctrl Pts',(41.4178740560063,38.3543320991532,42.8032587413542));
#36278=CARTESIAN_POINT('Ctrl Pts',(41.2083867170671,38.3543320991532,42.717234203378));
#36279=CARTESIAN_POINT('Ctrl Pts',(41.0959806464263,38.3543320991532,42.6429232657692));
#36280=CARTESIAN_POINT('Ctrl Pts',(40.9374140741385,38.3543320991532,42.4854573905017));
#36281=CARTESIAN_POINT('Ctrl Pts',(40.8628848373166,38.3543320991532,42.3748001680524));
#36282=CARTESIAN_POINT('Ctrl Pts',(40.801909587836,38.3543320991532,42.2284287129193));
#36283=CARTESIAN_POINT('Ctrl Pts',(40.7858998675388,38.3543320991532,42.1797227805058));
#36284=CARTESIAN_POINT('Ctrl Pts',(40.7743169556539,38.3543320991532,42.1294657090004));
#36285=CARTESIAN_POINT('',(45.2130570344595,38.3543320991532,42.8294657090004));
#36286=CARTESIAN_POINT('Origin',(43.4397894030341,37.9543320991532,42.8294657090004));
#36287=CARTESIAN_POINT('Ctrl Pts',(46.1052618504143,38.3543320991532,42.1294657090004));
#36288=CARTESIAN_POINT('Ctrl Pts',(46.0936789385295,38.3543320991532,42.1797227805058));
#36289=CARTESIAN_POINT('Ctrl Pts',(46.0776692182323,38.3543320991532,42.2284287129193));
#36290=CARTESIAN_POINT('Ctrl Pts',(46.0166939687517,38.3543320991532,42.3748001680524));
#36291=CARTESIAN_POINT('Ctrl Pts',(45.9421647319298,38.3543320991532,42.4854573905017));
#36292=CARTESIAN_POINT('Ctrl Pts',(45.783598159642,38.3543320991532,42.6429232657692));
#36293=CARTESIAN_POINT('Ctrl Pts',(45.6711920890012,38.3543320991532,42.717234203378));
#36294=CARTESIAN_POINT('Ctrl Pts',(45.461704750062,38.3543320991532,42.8032587413542));
#36295=CARTESIAN_POINT('Ctrl Pts',(45.3272286490232,38.3543320991532,42.8294657090004));
#36296=CARTESIAN_POINT('Ctrl Pts',(45.2130570344595,38.3543320991532,42.8294657090004));
#36297=CARTESIAN_POINT('Origin',(43.4397894030341,37.9543320991532,42.8294657090004));
#36298=CARTESIAN_POINT('',(46.2397894030341,37.9543320991532,41.0294657090004));
#36299=CARTESIAN_POINT('Origin',(43.4397894030341,37.9543320991532,41.0294657090004));
#36300=CARTESIAN_POINT('',(46.0823098086875,37.9543320991532,42.8294657090004));
#36301=CARTESIAN_POINT('Origin',(43.4397894030341,37.9543320991532,68.2294657090003));
#36302=CARTESIAN_POINT('',(41.9397894030341,37.9543320991532,41.0294657090004));
#36303=CARTESIAN_POINT('Origin',(43.4397894030341,37.9543320991532,41.0294657090004));
#36304=CARTESIAN_POINT('',(41.9397894030341,37.9543320991532,31.0294657090004));
#36305=CARTESIAN_POINT('',(41.9397894030341,37.9543320991532,68.2294657090003));
#36306=CARTESIAN_POINT('Origin',(43.4397894030341,37.9543320991532,31.0294657090004));
#36307=CARTESIAN_POINT('Origin',(43.4397894030341,37.9543320991532,42.8294657090004));
#36308=CARTESIAN_POINT('',(46.2397894030341,38.3543320991532,42.8294657090004));
#36309=CARTESIAN_POINT('Origin',(43.4397894030341,39.4543320991532,31.0294657090004));
#36310=CARTESIAN_POINT('Origin',(43.4397894030341,37.9543320991532,42.8294657090004));
#36311=CARTESIAN_POINT('',(40.6397894030341,37.5543320991532,42.8294657090004));
#36312=CARTESIAN_POINT('Origin',(43.4397894030341,39.4543320991532,41.0294657090004));
#36313=CARTESIAN_POINT('Origin',(46.2397894030341,38.3543320991532,42.1294657090004));
#36314=CARTESIAN_POINT('',(46.2397894030341,38.3543320991532,42.1294657090004));
#36315=CARTESIAN_POINT('Origin',(40.6397894030341,37.5543320991532,42.1294657090004));
#36316=CARTESIAN_POINT('',(40.6397894030341,37.5543320991532,42.1294657090004));
#36317=CARTESIAN_POINT('Origin',(40.6397894030341,38.3543320991532,42.1294657090004));
#36318=CARTESIAN_POINT('Origin',(16.1460502915689,27.3543320991532,35.0294657090004));
#36319=CARTESIAN_POINT('',(16.1460502915689,26.8543320991532,30.5294657090004));
#36320=CARTESIAN_POINT('Origin',(16.1460502915689,26.8543320991532,35.0294657090004));
#36321=CARTESIAN_POINT('',(16.1460502915689,27.3543320991532,31.0294657090004));
#36322=CARTESIAN_POINT('Origin',(16.1460502915689,27.3543320991532,30.5294657090004));
#36323=CARTESIAN_POINT('Origin',(16.1460502915689,27.3543320991532,35.0294657090004));
#36324=CARTESIAN_POINT('Origin',(16.1460502915689,42.4643320991532,35.0294657090004));
#36325=CARTESIAN_POINT('',(18.145143062111,42.4652393286112,35.0294657090004));
#36326=CARTESIAN_POINT('',(16.1460502915689,42.4652393286112,33.0303729384583));
#36327=CARTESIAN_POINT('Origin',(16.1460502915689,42.4652393286112,35.0294657090004));
#36328=CARTESIAN_POINT('Origin',(16.1460502915689,42.4652393286112,35.0294657090004));
#36329=CARTESIAN_POINT('',(16.1460502915689,42.8543320991532,33.4194657090004));
#36330=CARTESIAN_POINT('',(16.1460502915689,42.4643320991532,33.0294657090004));
#36331=CARTESIAN_POINT('Origin',(16.1460502915689,42.8543320991532,35.0294657090004));
#36332=CARTESIAN_POINT('Origin',(16.1460502915689,42.1927936376148,35.0294657090004));
#36333=CARTESIAN_POINT('',(16.1460502915689,41.919712697713,33.0294657090004));
#36334=CARTESIAN_POINT('',(14.1460502915689,41.919712697713,35.0294657090004));
#36335=CARTESIAN_POINT('Origin',(16.1460502915689,41.919712697713,35.0294657090004));
#36336=CARTESIAN_POINT('Origin',(16.1460502915689,41.919712697713,35.0294657090004));
#36337=CARTESIAN_POINT('',(14.5360502915689,42.1927936376148,35.0294657090004));
#36338=CARTESIAN_POINT('',(14.5360502915689,42.1927936376148,35.0294657090004));
#36339=CARTESIAN_POINT('',(17.7560502915689,42.1927936376148,35.0294657090004));
#36340=CARTESIAN_POINT('Origin',(16.1460502915689,42.1927936376148,35.0294657090004));
#36341=CARTESIAN_POINT('Origin',(16.1460502915689,42.1927936376148,35.0294657090004));
#36342=CARTESIAN_POINT('Origin',(16.1460502915689,42.4658745775166,35.0294657090004));
#36343=CARTESIAN_POINT('',(18.1460502915689,42.4658745775166,35.0294657090004));
#36344=CARTESIAN_POINT('Origin',(16.1460502915689,-2.04566790084674,35.0294657090004));
#36345=CARTESIAN_POINT('',(18.1460502915689,41.8043361159781,35.0294657090004));
#36346=CARTESIAN_POINT('',(16.1460502915689,41.8043361159781,33.0294657090004));
#36347=CARTESIAN_POINT('Origin',(16.1460502915689,41.8043361159781,35.0294657090004));
#36348=CARTESIAN_POINT('Origin',(16.1460502915689,41.8043361159781,35.0294657090004));
#36349=CARTESIAN_POINT('',(16.1460502915689,-2.04566790084674,33.0294657090004));
#36350=CARTESIAN_POINT('Origin',(16.1460502915689,41.5312551760763,35.0294657090004));
#36351=CARTESIAN_POINT('',(16.1460502915689,41.2581742361745,33.0294657090004));
#36352=CARTESIAN_POINT('',(14.1460502915689,41.2581742361745,35.0294657090004));
#36353=CARTESIAN_POINT('Origin',(16.1460502915689,41.2581742361745,35.0294657090004));
#36354=CARTESIAN_POINT('Origin',(16.1460502915689,41.2581742361745,35.0294657090004));
#36355=CARTESIAN_POINT('',(14.5360502915689,41.5312551760763,35.0294657090004));
#36356=CARTESIAN_POINT('',(14.5360502915689,41.5312551760763,35.0294657090004));
#36357=CARTESIAN_POINT('',(17.7560502915689,41.5312551760763,35.0294657090004));
#36358=CARTESIAN_POINT('Origin',(16.1460502915689,41.5312551760763,35.0294657090004));
#36359=CARTESIAN_POINT('Origin',(16.1460502915689,41.5312551760763,35.0294657090004));
#36360=CARTESIAN_POINT('Origin',(16.1460502915689,41.8043361159781,35.0294657090004));
#36361=CARTESIAN_POINT('',(18.1460502915689,41.8043361159781,35.0294657090004));
#36362=CARTESIAN_POINT('Origin',(16.1460502915689,-2.04566790084674,35.0294657090004));
#36363=CARTESIAN_POINT('',(18.1460502915689,41.1427976544396,35.0294657090004));
#36364=CARTESIAN_POINT('',(16.1460502915689,41.1427976544396,33.0294657090004));
#36365=CARTESIAN_POINT('Origin',(16.1460502915689,41.1427976544396,35.0294657090004));
#36366=CARTESIAN_POINT('Origin',(16.1460502915689,41.1427976544396,35.0294657090004));
#36367=CARTESIAN_POINT('',(16.1460502915689,-2.04566790084674,33.0294657090004));
#36368=CARTESIAN_POINT('Origin',(16.1460502915689,40.8697167145378,35.0294657090004));
#36369=CARTESIAN_POINT('',(16.1460502915689,40.5966357746361,33.0294657090004));
#36370=CARTESIAN_POINT('',(14.1460502915689,40.5966357746361,35.0294657090004));
#36371=CARTESIAN_POINT('Origin',(16.1460502915689,40.5966357746361,35.0294657090004));
#36372=CARTESIAN_POINT('Origin',(16.1460502915689,40.5966357746361,35.0294657090004));
#36373=CARTESIAN_POINT('',(14.5360502915689,40.8697167145378,35.0294657090004));
#36374=CARTESIAN_POINT('',(14.5360502915689,40.8697167145378,35.0294657090004));
#36375=CARTESIAN_POINT('',(17.7560502915689,40.8697167145378,35.0294657090004));
#36376=CARTESIAN_POINT('Origin',(16.1460502915689,40.8697167145378,35.0294657090004));
#36377=CARTESIAN_POINT('Origin',(16.1460502915689,40.8697167145378,35.0294657090004));
#36378=CARTESIAN_POINT('Origin',(16.1460502915689,41.1427976544396,35.0294657090004));
#36379=CARTESIAN_POINT('',(18.1460502915689,41.1427976544396,35.0294657090004));
#36380=CARTESIAN_POINT('Origin',(16.1460502915689,-2.04566790084674,35.0294657090004));
#36381=CARTESIAN_POINT('',(18.1460502915689,40.4812591929012,35.0294657090004));
#36382=CARTESIAN_POINT('',(16.1460502915689,40.4812591929012,33.0294657090004));
#36383=CARTESIAN_POINT('Origin',(16.1460502915689,40.4812591929012,35.0294657090004));
#36384=CARTESIAN_POINT('Origin',(16.1460502915689,40.4812591929012,35.0294657090004));
#36385=CARTESIAN_POINT('',(16.1460502915689,-2.04566790084674,33.0294657090004));
#36386=CARTESIAN_POINT('Origin',(16.1460502915689,40.2081782529994,35.0294657090004));
#36387=CARTESIAN_POINT('',(16.1460502915689,39.9350973130976,33.0294657090004));
#36388=CARTESIAN_POINT('',(14.1460502915689,39.9350973130976,35.0294657090004));
#36389=CARTESIAN_POINT('Origin',(16.1460502915689,39.9350973130976,35.0294657090004));
#36390=CARTESIAN_POINT('Origin',(16.1460502915689,39.9350973130976,35.0294657090004));
#36391=CARTESIAN_POINT('',(14.5360502915689,40.2081782529994,35.0294657090004));
#36392=CARTESIAN_POINT('',(14.5360502915689,40.2081782529994,35.0294657090004));
#36393=CARTESIAN_POINT('',(17.7560502915689,40.2081782529994,35.0294657090004));
#36394=CARTESIAN_POINT('Origin',(16.1460502915689,40.2081782529994,35.0294657090004));
#36395=CARTESIAN_POINT('Origin',(16.1460502915689,40.2081782529994,35.0294657090004));
#36396=CARTESIAN_POINT('Origin',(16.1460502915689,40.4812591929012,35.0294657090004));
#36397=CARTESIAN_POINT('',(18.1460502915689,40.4812591929012,35.0294657090004));
#36398=CARTESIAN_POINT('Origin',(16.1460502915689,-2.04566790084674,35.0294657090004));
#36399=CARTESIAN_POINT('',(18.1460502915689,39.8197207313627,35.0294657090004));
#36400=CARTESIAN_POINT('',(16.1460502915689,39.8197207313627,33.0294657090004));
#36401=CARTESIAN_POINT('Origin',(16.1460502915689,39.8197207313627,35.0294657090004));
#36402=CARTESIAN_POINT('Origin',(16.1460502915689,39.8197207313627,35.0294657090004));
#36403=CARTESIAN_POINT('',(16.1460502915689,-2.04566790084674,33.0294657090004));
#36404=CARTESIAN_POINT('Origin',(16.1460502915689,39.5466397914609,35.0294657090004));
#36405=CARTESIAN_POINT('',(16.1460502915689,39.2735588515591,33.0294657090004));
#36406=CARTESIAN_POINT('',(14.1460502915689,39.2735588515591,35.0294657090004));
#36407=CARTESIAN_POINT('Origin',(16.1460502915689,39.2735588515591,35.0294657090004));
#36408=CARTESIAN_POINT('Origin',(16.1460502915689,39.2735588515591,35.0294657090004));
#36409=CARTESIAN_POINT('',(14.5360502915689,39.5466397914609,35.0294657090004));
#36410=CARTESIAN_POINT('',(14.5360502915689,39.5466397914609,35.0294657090004));
#36411=CARTESIAN_POINT('',(17.7560502915689,39.5466397914609,35.0294657090004));
#36412=CARTESIAN_POINT('Origin',(16.1460502915689,39.5466397914609,35.0294657090004));
#36413=CARTESIAN_POINT('Origin',(16.1460502915689,39.5466397914609,35.0294657090004));
#36414=CARTESIAN_POINT('Origin',(16.1460502915689,39.8197207313627,35.0294657090004));
#36415=CARTESIAN_POINT('',(18.1460502915689,39.8197207313627,35.0294657090004));
#36416=CARTESIAN_POINT('Origin',(16.1460502915689,-2.04566790084674,35.0294657090004));
#36417=CARTESIAN_POINT('',(18.1460502915689,39.1581822698242,35.0294657090004));
#36418=CARTESIAN_POINT('',(16.1460502915689,39.1581822698242,33.0294657090004));
#36419=CARTESIAN_POINT('Origin',(16.1460502915689,39.1581822698242,35.0294657090004));
#36420=CARTESIAN_POINT('Origin',(16.1460502915689,39.1581822698242,35.0294657090004));
#36421=CARTESIAN_POINT('',(16.1460502915689,-2.04566790084674,33.0294657090004));
#36422=CARTESIAN_POINT('Origin',(16.1460502915689,38.8851013299225,35.0294657090004));
#36423=CARTESIAN_POINT('',(16.1460502915689,38.6120203900207,33.0294657090004));
#36424=CARTESIAN_POINT('',(14.1460502915689,38.6120203900207,35.0294657090004));
#36425=CARTESIAN_POINT('Origin',(16.1460502915689,38.6120203900207,35.0294657090004));
#36426=CARTESIAN_POINT('Origin',(16.1460502915689,38.6120203900207,35.0294657090004));
#36427=CARTESIAN_POINT('',(14.5360502915689,38.8851013299225,35.0294657090004));
#36428=CARTESIAN_POINT('',(14.5360502915689,38.8851013299225,35.0294657090004));
#36429=CARTESIAN_POINT('',(17.7560502915689,38.8851013299225,35.0294657090004));
#36430=CARTESIAN_POINT('Origin',(16.1460502915689,38.8851013299225,35.0294657090004));
#36431=CARTESIAN_POINT('Origin',(16.1460502915689,38.8851013299225,35.0294657090004));
#36432=CARTESIAN_POINT('Origin',(16.1460502915689,39.1581822698242,35.0294657090004));
#36433=CARTESIAN_POINT('',(18.1460502915689,39.1581822698242,35.0294657090004));
#36434=CARTESIAN_POINT('Origin',(16.1460502915689,-2.04566790084674,35.0294657090004));
#36435=CARTESIAN_POINT('',(18.1460502915689,38.4966438082858,35.0294657090004));
#36436=CARTESIAN_POINT('',(16.1460502915689,38.4966438082858,33.0294657090004));
#36437=CARTESIAN_POINT('Origin',(16.1460502915689,38.4966438082858,35.0294657090004));
#36438=CARTESIAN_POINT('Origin',(16.1460502915689,38.4966438082858,35.0294657090004));
#36439=CARTESIAN_POINT('',(16.1460502915689,-2.04566790084674,33.0294657090004));
#36440=CARTESIAN_POINT('Origin',(16.1460502915689,38.223562868384,35.0294657090004));
#36441=CARTESIAN_POINT('',(16.1460502915689,37.9504819284822,33.0294657090004));
#36442=CARTESIAN_POINT('',(14.1460502915689,37.9504819284822,35.0294657090004));
#36443=CARTESIAN_POINT('Origin',(16.1460502915689,37.9504819284822,35.0294657090004));
#36444=CARTESIAN_POINT('Origin',(16.1460502915689,37.9504819284822,35.0294657090004));
#36445=CARTESIAN_POINT('',(14.5360502915689,38.223562868384,35.0294657090004));
#36446=CARTESIAN_POINT('',(14.5360502915689,38.223562868384,35.0294657090004));
#36447=CARTESIAN_POINT('',(17.7560502915689,38.223562868384,35.0294657090004));
#36448=CARTESIAN_POINT('Origin',(16.1460502915689,38.223562868384,35.0294657090004));
#36449=CARTESIAN_POINT('Origin',(16.1460502915689,38.223562868384,35.0294657090004));
#36450=CARTESIAN_POINT('Origin',(16.1460502915689,38.4966438082858,35.0294657090004));
#36451=CARTESIAN_POINT('',(18.1460502915689,38.4966438082858,35.0294657090004));
#36452=CARTESIAN_POINT('Origin',(16.1460502915689,-2.04566790084674,35.0294657090004));
#36453=CARTESIAN_POINT('',(18.1460502915689,37.8351053467473,35.0294657090004));
#36454=CARTESIAN_POINT('',(16.1460502915689,37.8351053467473,33.0294657090004));
#36455=CARTESIAN_POINT('Origin',(16.1460502915689,37.8351053467473,35.0294657090004));
#36456=CARTESIAN_POINT('Origin',(16.1460502915689,37.8351053467473,35.0294657090004));
#36457=CARTESIAN_POINT('',(16.1460502915689,-2.04566790084674,33.0294657090004));
#36458=CARTESIAN_POINT('Origin',(16.1460502915689,37.5620244068455,35.0294657090004));
#36459=CARTESIAN_POINT('',(16.1460502915689,37.2889434669437,33.0294657090004));
#36460=CARTESIAN_POINT('',(14.1460502915689,37.2889434669437,35.0294657090004));
#36461=CARTESIAN_POINT('Origin',(16.1460502915689,37.2889434669437,35.0294657090004));
#36462=CARTESIAN_POINT('Origin',(16.1460502915689,37.2889434669437,35.0294657090004));
#36463=CARTESIAN_POINT('',(14.5360502915689,37.5620244068455,35.0294657090004));
#36464=CARTESIAN_POINT('',(14.5360502915689,37.5620244068455,35.0294657090004));
#36465=CARTESIAN_POINT('',(17.7560502915689,37.5620244068455,35.0294657090004));
#36466=CARTESIAN_POINT('Origin',(16.1460502915689,37.5620244068455,35.0294657090004));
#36467=CARTESIAN_POINT('Origin',(16.1460502915689,37.5620244068455,35.0294657090004));
#36468=CARTESIAN_POINT('Origin',(16.1460502915689,37.8351053467473,35.0294657090004));
#36469=CARTESIAN_POINT('',(18.1460502915689,37.8351053467473,35.0294657090004));
#36470=CARTESIAN_POINT('Origin',(16.1460502915689,-2.04566790084674,35.0294657090004));
#36471=CARTESIAN_POINT('',(18.1460502915689,37.1735668852089,35.0294657090004));
#36472=CARTESIAN_POINT('',(16.1460502915689,37.1735668852089,33.0294657090004));
#36473=CARTESIAN_POINT('Origin',(16.1460502915689,37.1735668852089,35.0294657090004));
#36474=CARTESIAN_POINT('Origin',(16.1460502915689,37.1735668852089,35.0294657090004));
#36475=CARTESIAN_POINT('',(16.1460502915689,-2.04566790084674,33.0294657090004));
#36476=CARTESIAN_POINT('Origin',(16.1460502915689,36.9004859453071,35.0294657090004));
#36477=CARTESIAN_POINT('',(16.1460502915689,36.6274050054053,33.0294657090004));
#36478=CARTESIAN_POINT('',(14.1460502915689,36.6274050054053,35.0294657090004));
#36479=CARTESIAN_POINT('Origin',(16.1460502915689,36.6274050054053,35.0294657090004));
#36480=CARTESIAN_POINT('Origin',(16.1460502915689,36.6274050054053,35.0294657090004));
#36481=CARTESIAN_POINT('',(14.5360502915689,36.9004859453071,35.0294657090004));
#36482=CARTESIAN_POINT('',(14.5360502915689,36.9004859453071,35.0294657090004));
#36483=CARTESIAN_POINT('',(17.7560502915689,36.9004859453071,35.0294657090004));
#36484=CARTESIAN_POINT('Origin',(16.1460502915689,36.9004859453071,35.0294657090004));
#36485=CARTESIAN_POINT('Origin',(16.1460502915689,36.9004859453071,35.0294657090004));
#36486=CARTESIAN_POINT('Origin',(16.1460502915689,37.1735668852089,35.0294657090004));
#36487=CARTESIAN_POINT('',(18.1460502915689,37.1735668852089,35.0294657090004));
#36488=CARTESIAN_POINT('Origin',(16.1460502915689,-2.04566790084674,35.0294657090004));
#36489=CARTESIAN_POINT('',(18.1460502915689,36.5120284236704,35.0294657090004));
#36490=CARTESIAN_POINT('',(16.1460502915689,36.5120284236704,33.0294657090004));
#36491=CARTESIAN_POINT('Origin',(16.1460502915689,36.5120284236704,35.0294657090004));
#36492=CARTESIAN_POINT('Origin',(16.1460502915689,36.5120284236704,35.0294657090004));
#36493=CARTESIAN_POINT('',(16.1460502915689,-2.04566790084674,33.0294657090004));
#36494=CARTESIAN_POINT('Origin',(16.1460502915689,36.2389474837686,35.0294657090004));
#36495=CARTESIAN_POINT('',(16.1460502915689,35.9658665438668,33.0294657090004));
#36496=CARTESIAN_POINT('',(14.1460502915689,35.9658665438668,35.0294657090004));
#36497=CARTESIAN_POINT('Origin',(16.1460502915689,35.9658665438668,35.0294657090004));
#36498=CARTESIAN_POINT('Origin',(16.1460502915689,35.9658665438668,35.0294657090004));
#36499=CARTESIAN_POINT('',(14.5360502915689,36.2389474837686,35.0294657090004));
#36500=CARTESIAN_POINT('',(14.5360502915689,36.2389474837686,35.0294657090004));
#36501=CARTESIAN_POINT('',(17.7560502915689,36.2389474837686,35.0294657090004));
#36502=CARTESIAN_POINT('Origin',(16.1460502915689,36.2389474837686,35.0294657090004));
#36503=CARTESIAN_POINT('Origin',(16.1460502915689,36.2389474837686,35.0294657090004));
#36504=CARTESIAN_POINT('Origin',(16.1460502915689,36.5120284236704,35.0294657090004));
#36505=CARTESIAN_POINT('',(18.1460502915689,36.5120284236704,35.0294657090004));
#36506=CARTESIAN_POINT('Origin',(16.1460502915689,-2.04566790084674,35.0294657090004));
#36507=CARTESIAN_POINT('',(18.1460502915689,35.8504899621319,35.0294657090004));
#36508=CARTESIAN_POINT('',(16.1460502915689,35.8504899621319,33.0294657090004));
#36509=CARTESIAN_POINT('Origin',(16.1460502915689,35.8504899621319,35.0294657090004));
#36510=CARTESIAN_POINT('Origin',(16.1460502915689,35.8504899621319,35.0294657090004));
#36511=CARTESIAN_POINT('',(16.1460502915689,-2.04566790084674,33.0294657090004));
#36512=CARTESIAN_POINT('Origin',(16.1460502915689,35.5774090222301,35.0294657090004));
#36513=CARTESIAN_POINT('',(16.1460502915689,35.3043280823284,33.0294657090004));
#36514=CARTESIAN_POINT('',(14.1460502915689,35.3043280823284,35.0294657090004));
#36515=CARTESIAN_POINT('Origin',(16.1460502915689,35.3043280823284,35.0294657090004));
#36516=CARTESIAN_POINT('Origin',(16.1460502915689,35.3043280823284,35.0294657090004));
#36517=CARTESIAN_POINT('',(14.5360502915689,35.5774090222301,35.0294657090004));
#36518=CARTESIAN_POINT('',(14.5360502915689,35.5774090222301,35.0294657090004));
#36519=CARTESIAN_POINT('',(17.7560502915689,35.5774090222301,35.0294657090004));
#36520=CARTESIAN_POINT('Origin',(16.1460502915689,35.5774090222301,35.0294657090004));
#36521=CARTESIAN_POINT('Origin',(16.1460502915689,35.5774090222301,35.0294657090004));
#36522=CARTESIAN_POINT('Origin',(16.1460502915689,35.8504899621319,35.0294657090004));
#36523=CARTESIAN_POINT('',(18.1460502915689,35.8504899621319,35.0294657090004));
#36524=CARTESIAN_POINT('Origin',(16.1460502915689,-2.04566790084674,35.0294657090004));
#36525=CARTESIAN_POINT('',(18.1460502915689,35.1889515005935,35.0294657090004));
#36526=CARTESIAN_POINT('',(16.1460502915689,35.1889515005935,33.0294657090004));
#36527=CARTESIAN_POINT('Origin',(16.1460502915689,35.1889515005935,35.0294657090004));
#36528=CARTESIAN_POINT('Origin',(16.1460502915689,35.1889515005935,35.0294657090004));
#36529=CARTESIAN_POINT('',(16.1460502915689,-2.04566790084674,33.0294657090004));
#36530=CARTESIAN_POINT('Origin',(16.1460502915689,34.9158705606917,35.0294657090004));
#36531=CARTESIAN_POINT('',(16.1460502915689,34.6427896207899,33.0294657090004));
#36532=CARTESIAN_POINT('',(14.1460502915689,34.6427896207899,35.0294657090004));
#36533=CARTESIAN_POINT('Origin',(16.1460502915689,34.6427896207899,35.0294657090004));
#36534=CARTESIAN_POINT('Origin',(16.1460502915689,34.6427896207899,35.0294657090004));
#36535=CARTESIAN_POINT('',(14.5360502915689,34.9158705606917,35.0294657090004));
#36536=CARTESIAN_POINT('',(14.5360502915689,34.9158705606917,35.0294657090004));
#36537=CARTESIAN_POINT('',(17.7560502915689,34.9158705606917,35.0294657090004));
#36538=CARTESIAN_POINT('Origin',(16.1460502915689,34.9158705606917,35.0294657090004));
#36539=CARTESIAN_POINT('Origin',(16.1460502915689,34.9158705606917,35.0294657090004));
#36540=CARTESIAN_POINT('Origin',(16.1460502915689,35.1889515005935,35.0294657090004));
#36541=CARTESIAN_POINT('',(18.1460502915689,35.1889515005935,35.0294657090004));
#36542=CARTESIAN_POINT('Origin',(16.1460502915689,-2.04566790084674,35.0294657090004));
#36543=CARTESIAN_POINT('',(18.1460502915689,34.527413039055,35.0294657090004));
#36544=CARTESIAN_POINT('',(16.1460502915689,34.527413039055,33.0294657090004));
#36545=CARTESIAN_POINT('Origin',(16.1460502915689,34.527413039055,35.0294657090004));
#36546=CARTESIAN_POINT('Origin',(16.1460502915689,34.527413039055,35.0294657090004));
#36547=CARTESIAN_POINT('',(16.1460502915689,-2.04566790084674,33.0294657090004));
#36548=CARTESIAN_POINT('Origin',(16.1460502915689,34.2543320991532,35.0294657090004));
#36549=CARTESIAN_POINT('',(16.1460502915689,33.9812511592514,33.0294657090004));
#36550=CARTESIAN_POINT('',(14.1460502915689,33.9812511592514,35.0294657090004));
#36551=CARTESIAN_POINT('Origin',(16.1460502915689,33.9812511592514,35.0294657090004));
#36552=CARTESIAN_POINT('Origin',(16.1460502915689,33.9812511592514,35.0294657090004));
#36553=CARTESIAN_POINT('',(14.5360502915689,34.2543320991532,35.0294657090004));
#36554=CARTESIAN_POINT('',(14.5360502915689,34.2543320991532,35.0294657090004));
#36555=CARTESIAN_POINT('',(17.7560502915689,34.2543320991532,35.0294657090004));
#36556=CARTESIAN_POINT('Origin',(16.1460502915689,34.2543320991532,35.0294657090004));
#36557=CARTESIAN_POINT('Origin',(16.1460502915689,34.2543320991532,35.0294657090004));
#36558=CARTESIAN_POINT('Origin',(16.1460502915689,34.527413039055,35.0294657090004));
#36559=CARTESIAN_POINT('',(18.1460502915689,34.527413039055,35.0294657090004));
#36560=CARTESIAN_POINT('Origin',(16.1460502915689,-2.04566790084674,35.0294657090004));
#36561=CARTESIAN_POINT('',(16.1460502915689,32.8543320991532,31.0294657090004));
#36562=CARTESIAN_POINT('',(16.1460502915689,-2.04566790084674,31.0294657090004));
#36563=CARTESIAN_POINT('Origin',(16.1460502915689,32.8543320991532,35.0294657090004));
#36564=CARTESIAN_POINT('Origin',(16.1460502915689,26.4543320991532,35.0294657090004));
#36565=CARTESIAN_POINT('',(15.9854118096116,26.7543320991532,42.9028271434904));
#36566=CARTESIAN_POINT('',(16.151451780189,26.4543320991532,43.2044639245305));
#36567=CARTESIAN_POINT('Ctrl Pts',(16.151451780189,26.4543320991532,43.2044639245305));
#36568=CARTESIAN_POINT('Ctrl Pts',(16.0668800194744,26.6080253707889,43.0508264986736));
#36569=CARTESIAN_POINT('Ctrl Pts',(15.9854118096116,26.7543320991532,42.9028271434904));
#36570=CARTESIAN_POINT('',(16.4740999163387,26.4543320991532,43.1978810047409));
#36571=CARTESIAN_POINT('Origin',(16.1460502915689,26.4543320991532,35.0294657090004));
#36572=CARTESIAN_POINT('',(16.627698370541,26.7543320991532,42.8897227103981));
#36573=CARTESIAN_POINT('Ctrl Pts',(16.4740999163387,26.4543320991532,43.1978810047409));
#36574=CARTESIAN_POINT('Ctrl Pts',(16.5523346430118,26.6080253707889,43.0409218735102));
#36575=CARTESIAN_POINT('Ctrl Pts',(16.627698370541,26.7543320991532,42.8897227103981));
#36576=CARTESIAN_POINT('',(16.8177720547276,26.4543320991532,43.1768220208907));
#36577=CARTESIAN_POINT('Ctrl Pts',(16.627698370541,26.7543320991532,42.8897227103981));
#36578=CARTESIAN_POINT('Ctrl Pts',(16.7209588230625,26.6080253707889,43.0305891945183));
#36579=CARTESIAN_POINT('Ctrl Pts',(16.8177720547276,26.4543320991532,43.1768220208907));
#36580=CARTESIAN_POINT('',(17.1388100367452,26.4543320991532,43.1439621868083));
#36581=CARTESIAN_POINT('Origin',(16.1460502915689,26.4543320991532,35.0294657090004));
#36582=CARTESIAN_POINT('',(17.2667796429711,26.7543320991532,42.8243095638127));
#36583=CARTESIAN_POINT('Ctrl Pts',(17.1388100367452,26.4543320991532,43.1439621868083));
#36584=CARTESIAN_POINT('Ctrl Pts',(17.2039908174864,26.6080253707889,42.981148467619));
#36585=CARTESIAN_POINT('Ctrl Pts',(17.2667796429711,26.7543320991532,42.8243095638127));
#36586=CARTESIAN_POINT('',(17.4796221317587,26.4543320991532,43.0949608052144));
#36587=CARTESIAN_POINT('Ctrl Pts',(17.2667796429711,26.7543320991532,42.8243095638127));
#36588=CARTESIAN_POINT('Ctrl Pts',(17.3712117052267,26.6080253707889,42.9571057336593));
#36589=CARTESIAN_POINT('Ctrl Pts',(17.4796221317587,26.4543320991532,43.0949608052144));
#36590=CARTESIAN_POINT('',(17.7969135048413,26.4543320991532,43.0360427336136));
#36591=CARTESIAN_POINT('Origin',(16.1460502915689,26.4543320991532,35.0294657090004));
#36592=CARTESIAN_POINT('',(17.8984026464749,26.7543320991532,42.7070230174322));
#36593=CARTESIAN_POINT('Ctrl Pts',(17.7969135048413,26.4543320991532,43.0360427336136));
#36594=CARTESIAN_POINT('Ctrl Pts',(17.8486065723089,26.6080253707889,42.8684579249044));
#36595=CARTESIAN_POINT('Ctrl Pts',(17.8984026464749,26.7543320991532,42.7070230174322));
#36596=CARTESIAN_POINT('',(18.1325975082171,26.4543320991532,42.9594250503859));
#36597=CARTESIAN_POINT('Ctrl Pts',(17.8984026464749,26.7543320991532,42.7070230174322));
#36598=CARTESIAN_POINT('Ctrl Pts',(18.0133113403204,26.6080253707889,42.8308651364048));
#36599=CARTESIAN_POINT('Ctrl Pts',(18.1325975082171,26.4543320991532,42.9594250503859));
#36600=CARTESIAN_POINT('',(18.4440307506264,26.4543320991532,42.8748408313122));
#36601=CARTESIAN_POINT('Origin',(16.1460502915689,26.4543320991532,35.0294657090004));
#36602=CARTESIAN_POINT('',(18.5183640341747,26.7543320991532,42.5386435938719));
#36603=CARTESIAN_POINT('Ctrl Pts',(18.4440307506264,26.4543320991532,42.8748408313122));
#36604=CARTESIAN_POINT('Ctrl Pts',(18.4818920959851,26.6080253707889,42.7036001823356));
#36605=CARTESIAN_POINT('Ctrl Pts',(18.5183640341747,26.7543320991532,42.5386435938719));
#36606=CARTESIAN_POINT('',(18.772352740706,26.4543320991532,42.7711167244916));
#36607=CARTESIAN_POINT('Ctrl Pts',(18.5183640341747,26.7543320991532,42.5386435938719));
#36608=CARTESIAN_POINT('Ctrl Pts',(18.6429846612111,26.6080253707889,42.6527075131012));
#36609=CARTESIAN_POINT('Ctrl Pts',(18.772352740706,26.4543320991532,42.7711167244916));
#36610=CARTESIAN_POINT('',(19.0758553155965,26.4543320991532,42.6614292519677));
#36611=CARTESIAN_POINT('Origin',(16.1460502915689,26.4543320991532,35.0294657090004));
#36612=CARTESIAN_POINT('',(19.1225380653216,26.7543320991532,42.3202918304149));
#36613=CARTESIAN_POINT('Ctrl Pts',(19.0758553155965,26.4543320991532,42.6614292519677));
#36614=CARTESIAN_POINT('Ctrl Pts',(19.0996329778397,26.6080253707889,42.4876723409899));
#36615=CARTESIAN_POINT('Ctrl Pts',(19.1225380653216,26.7543320991532,42.3202918304149));
#36616=CARTESIAN_POINT('',(19.3946303637053,26.4543320991532,42.5312889883718));
#36617=CARTESIAN_POINT('Ctrl Pts',(19.1225380653216,26.7543320991532,42.3202918304149));
#36618=CARTESIAN_POINT('Ctrl Pts',(19.256041295837,26.6080253707889,42.4238184733377));
#36619=CARTESIAN_POINT('Ctrl Pts',(19.3946303637053,26.4543320991532,42.5312889883718));
#36620=CARTESIAN_POINT('',(19.6881825115155,26.4543320991532,42.3972282144301));
#36621=CARTESIAN_POINT('Origin',(16.1460502915689,26.4543320991532,35.0294657090004));
#36622=CARTESIAN_POINT('',(19.7069040614201,26.7543320991532,42.0534208220216));
#36623=CARTESIAN_POINT('Ctrl Pts',(19.6881825115155,26.4543320991532,42.3972282144301));
#36624=CARTESIAN_POINT('Ctrl Pts',(19.697718254224,26.6080253707889,42.2221113650258));
#36625=CARTESIAN_POINT('Ctrl Pts',(19.7069040614201,26.7543320991532,42.0534208220216));
#36626=CARTESIAN_POINT('',(19.9952892223025,26.4543320991532,42.2415378560414));
#36627=CARTESIAN_POINT('Ctrl Pts',(19.7069040614201,26.7543320991532,42.0534208220216));
#36628=CARTESIAN_POINT('Ctrl Pts',(19.8484014534418,26.6080253707889,42.1457212359098));
#36629=CARTESIAN_POINT('Ctrl Pts',(19.9952892223025,26.4543320991532,42.2415378560414));
#36630=CARTESIAN_POINT('',(20.2769374019215,26.4543320991532,42.0839959330141));
#36631=CARTESIAN_POINT('Origin',(16.1460502915689,26.4543320991532,35.0294657090004));
#36632=CARTESIAN_POINT('',(20.2675731631798,26.7543320991532,41.7398065512221));
#36633=CARTESIAN_POINT('Ctrl Pts',(20.2769374019215,26.4543320991532,42.0839959330141));
#36634=CARTESIAN_POINT('Ctrl Pts',(20.2721677663007,26.6080253707889,41.9086845189238));
#36635=CARTESIAN_POINT('Ctrl Pts',(20.2675731631798,26.7543320991532,41.7398065512221));
#36636=CARTESIAN_POINT('',(20.5703320308954,26.4543320991532,41.9037915734806));
#36637=CARTESIAN_POINT('Ctrl Pts',(20.2675731631798,26.7543320991532,41.7398065512221));
#36638=CARTESIAN_POINT('Ctrl Pts',(20.4161230749094,26.6080253707889,41.8202664920499));
#36639=CARTESIAN_POINT('Ctrl Pts',(20.5703320308954,26.4543320991532,41.9037915734806));
#36640=CARTESIAN_POINT('',(20.8382019201565,26.4543320991532,41.7238169168728));
#36641=CARTESIAN_POINT('Origin',(16.1460502915689,26.4543320991532,35.0294657090004));
#36642=CARTESIAN_POINT('',(20.8008142102323,26.7543320991532,41.3815360692459));
#36643=CARTESIAN_POINT('Ctrl Pts',(20.8382019201565,26.4543320991532,41.7238169168728));
#36644=CARTESIAN_POINT('Ctrl Pts',(20.8191586473446,26.6080253707889,41.5494776066329));
#36645=CARTESIAN_POINT('Ctrl Pts',(20.8008142102323,26.7543320991532,41.3815360692459));
#36646=CARTESIAN_POINT('',(21.1159319744682,26.4543320991532,41.5202977864757));
#36647=CARTESIAN_POINT('Ctrl Pts',(20.8008142102323,26.7543320991532,41.3815360692459));
#36648=CARTESIAN_POINT('Ctrl Pts',(20.9554280665163,26.6080253707889,41.449620089382));
#36649=CARTESIAN_POINT('Ctrl Pts',(21.1159319744682,26.4543320991532,41.5202977864757));
#36650=CARTESIAN_POINT('',(21.3682409434537,26.4543320991532,41.3190880979334));
#36651=CARTESIAN_POINT('Origin',(16.1460502915689,26.4543320991532,35.0294657090004));
#36652=CARTESIAN_POINT('',(21.3030785713881,26.7543320991532,40.9809936070401));
#36653=CARTESIAN_POINT('Ctrl Pts',(21.3682409434537,26.4543320991532,41.3190880979334));
#36654=CARTESIAN_POINT('Ctrl Pts',(21.3350507632894,26.6080253707889,41.1468810908896));
#36655=CARTESIAN_POINT('Ctrl Pts',(21.3030785713881,26.7543320991532,40.9809936070401));
#36656=CARTESIAN_POINT('',(21.628458175414,26.4543320991532,41.0936085829071));
#36657=CARTESIAN_POINT('Ctrl Pts',(21.3030785713881,26.7543320991532,40.9809936070401));
#36658=CARTESIAN_POINT('Ctrl Pts',(21.4627274425223,26.6080253707889,41.0362486185636));
#36659=CARTESIAN_POINT('Ctrl Pts',(21.628458175414,26.4543320991532,41.0936085829071));
#36660=CARTESIAN_POINT('',(21.8635271495635,26.4543320991532,40.8725028797102));
#36661=CARTESIAN_POINT('Origin',(16.1460502915689,26.4543320991532,35.0294657090004));
#36662=CARTESIAN_POINT('',(21.7710237601915,26.7543320991532,40.5408447086059));
#36663=CARTESIAN_POINT('Ctrl Pts',(21.8635271495635,26.4543320991532,40.8725028797102));
#36664=CARTESIAN_POINT('Ctrl Pts',(21.8164109372198,26.6080253707889,40.7035741850823));
#36665=CARTESIAN_POINT('Ctrl Pts',(21.7710237601915,26.7543320991532,40.5408447086059));
#36666=CARTESIAN_POINT('',(22.1044998564265,26.4543320991532,40.6265635090257));
#36667=CARTESIAN_POINT('Ctrl Pts',(21.7710237601915,26.7543320991532,40.5408447086059));
#36668=CARTESIAN_POINT('Ctrl Pts',(21.9346452092787,26.6080253707889,40.5829029985315));
#36669=CARTESIAN_POINT('Ctrl Pts',(22.1044998564265,26.4543320991532,40.6265635090257));
#36670=CARTESIAN_POINT('',(22.3207644905006,26.4543320991532,40.3870332131493));
#36671=CARTESIAN_POINT('Origin',(16.1460502915689,26.4543320991532,35.0294657090004));
#36672=CARTESIAN_POINT('',(22.2015356786164,26.7543320991532,40.0640184922428));
#36673=CARTESIAN_POINT('Ctrl Pts',(22.3207644905005,26.4543320991532,40.3870332131493));
#36674=CARTESIAN_POINT('Ctrl Pts',(22.260035796597,26.6080253707889,40.2225070235287));
#36675=CARTESIAN_POINT('Ctrl Pts',(22.2015356786164,26.7543320991532,40.0640184922428));
#36676=CARTESIAN_POINT('',(22.5408890386598,26.4543320991532,40.1222706727414));
#36677=CARTESIAN_POINT('Ctrl Pts',(22.2015356786164,26.7543320991532,40.0640184922428));
#36678=CARTESIAN_POINT('Ctrl Pts',(22.3680408319088,26.6080253707889,40.0926001695902));
#36679=CARTESIAN_POINT('Ctrl Pts',(22.5408890386598,26.4543320991532,40.1222706727413));
#36680=CARTESIAN_POINT('',(22.7369101271999,26.4543320991532,39.8659098187846));
#36681=CARTESIAN_POINT('Origin',(16.1460502915689,26.4543320991532,35.0294657090004));
#36682=CARTESIAN_POINT('',(22.5917493408754,26.7543320991532,39.55368815775));
#36683=CARTESIAN_POINT('Ctrl Pts',(22.7369101271999,26.4543320991532,39.8659098187846));
#36684=CARTESIAN_POINT('Ctrl Pts',(22.6629730911748,26.6080253707889,39.7068810288184));
#36685=CARTESIAN_POINT('Ctrl Pts',(22.5917493408754,26.7543320991532,39.55368815775));
#36686=CARTESIAN_POINT('',(22.9347216241054,26.4543320991532,39.584086059677));
#36687=CARTESIAN_POINT('Ctrl Pts',(22.5917493408754,26.7543320991532,39.55368815775));
#36688=CARTESIAN_POINT('Ctrl Pts',(22.760030134049,26.6080253707889,39.5686030161721));
#36689=CARTESIAN_POINT('Ctrl Pts',(22.9347216241054,26.4543320991532,39.584086059677));
#36690=CARTESIAN_POINT('',(23.1091946791084,26.4543320991532,39.3126006868265));
#36691=CARTESIAN_POINT('Origin',(16.1460502915689,26.4543320991532,35.0294657090004));
#36692=CARTESIAN_POINT('',(22.9390679394267,26.7543320991532,39.0132498693049));
#36693=CARTESIAN_POINT('Ctrl Pts',(23.1091946791084,26.4543320991532,39.3126006868265));
#36694=CARTESIAN_POINT('Ctrl Pts',(23.0225413397378,26.6080253707889,39.1601276068739));
#36695=CARTESIAN_POINT('Ctrl Pts',(22.9390679394267,26.7543320991532,39.0132498693049));
#36696=CARTESIAN_POINT('',(23.2833767218849,26.4543320991532,39.0155911996383));
#36697=CARTESIAN_POINT('Ctrl Pts',(22.9390679394267,26.7543320991532,39.0132498693049));
#36698=CARTESIAN_POINT('Ctrl Pts',(23.1080044915674,26.6080253707889,39.0143986528797));
#36699=CARTESIAN_POINT('Ctrl Pts',(23.2833767218849,26.4543320991532,39.0155911996383));
#36700=CARTESIAN_POINT('',(23.4351406539558,26.4543320991532,38.7307879982584));
#36701=CARTESIAN_POINT('Origin',(16.1460502915689,26.4543320991532,35.0294657090004));
#36702=CARTESIAN_POINT('',(23.2411801263005,26.7543320991532,38.4463001545511));
#36703=CARTESIAN_POINT('Ctrl Pts',(23.4351406539558,26.4543320991532,38.7307879982584));
#36704=CARTESIAN_POINT('Ctrl Pts',(23.3363476749164,26.6080253707889,38.5858853115103));
#36705=CARTESIAN_POINT('Ctrl Pts',(23.2411801263005,26.7543320991532,38.4463001545511));
#36706=CARTESIAN_POINT('',(23.5845340898466,26.4543320991532,38.4205693321238));
#36707=CARTESIAN_POINT('Ctrl Pts',(23.2411801263005,26.7543320991532,38.4463001545511));
#36708=CARTESIAN_POINT('Ctrl Pts',(23.4096481925264,26.6080253707889,38.4336752183134));
#36709=CARTESIAN_POINT('Ctrl Pts',(23.5845340898466,26.4543320991532,38.4205693321238));
#36710=CARTESIAN_POINT('',(23.7125789350568,26.4543320991532,38.1243436205306));
#36711=CARTESIAN_POINT('Origin',(16.1460502915689,26.4543320991532,35.0294657090004));
#36712=CARTESIAN_POINT('',(23.4960753947382,26.7543320991532,37.8566119703002));
#36713=CARTESIAN_POINT('Ctrl Pts',(23.7125789350568,26.4543320991532,38.1243436205305));
#36714=CARTESIAN_POINT('Ctrl Pts',(23.6023037673244,26.6080253707889,37.9879756304599));
#36715=CARTESIAN_POINT('Ctrl Pts',(23.4960753947382,26.7543320991532,37.8566119703002));
#36716=CARTESIAN_POINT('',(23.8361895753942,26.4543320991532,37.8029802294902));
#36717=CARTESIAN_POINT('Ctrl Pts',(23.4960753947382,26.7543320991532,37.8566119703002));
#36718=CARTESIAN_POINT('Ctrl Pts',(23.6629538478638,26.6080253707889,37.8302973311177));
#36719=CARTESIAN_POINT('Ctrl Pts',(23.8361895753942,26.4543320991532,37.8029802294902));
#36720=CARTESIAN_POINT('',(23.9396632164247,26.4543320991532,37.4973033409204));
#36721=CARTESIAN_POINT('Origin',(16.1460502915689,26.4543320991532,35.0294657090004));
#36722=CARTESIAN_POINT('',(23.7020574587831,26.7543320991532,37.2481095941266));
#36723=CARTESIAN_POINT('Ctrl Pts',(23.9396632164247,26.4543320991532,37.4973033409204));
#36724=CARTESIAN_POINT('Ctrl Pts',(23.8186397230465,26.6080253707889,37.370377554002));
#36725=CARTESIAN_POINT('Ctrl Pts',(23.7020574587831,26.7543320991532,37.2481095941266));
#36726=CARTESIAN_POINT('',(24.0366684527916,26.4543320991532,37.1669338453204));
#36727=CARTESIAN_POINT('Ctrl Pts',(23.7020574587831,26.7543320991532,37.2481095941266));
#36728=CARTESIAN_POINT('Ctrl Pts',(23.8662357502359,26.6080253707889,37.2082803715815));
#36729=CARTESIAN_POINT('Ctrl Pts',(24.0366684527916,26.4543320991532,37.1669338453204));
#36730=CARTESIAN_POINT('',(24.1148822896334,26.4543320991532,36.8538400090343));
#36731=CARTESIAN_POINT('Origin',(16.1460502915689,26.4543320991532,35.0294657090004));
#36732=CARTESIAN_POINT('',(23.8577555417836,26.7543320991532,36.6248425089479));
#36733=CARTESIAN_POINT('Ctrl Pts',(24.1148822896334,26.4543320991532,36.8538400090343));
#36734=CARTESIAN_POINT('Ctrl Pts',(23.9839158619903,26.6080253707889,36.7372010954389));
#36735=CARTESIAN_POINT('Ctrl Pts',(23.8577555417836,26.7543320991532,36.6248425089479));
#36736=CARTESIAN_POINT('',(24.1846365681864,26.4543320991532,36.5166629633608));
#36737=CARTESIAN_POINT('Ctrl Pts',(23.8577555417836,26.7543320991532,36.624842508948));
#36738=CARTESIAN_POINT('Ctrl Pts',(24.0181410921214,26.6080253707889,36.5717637599449));
#36739=CARTESIAN_POINT('Ctrl Pts',(24.1846365681864,26.4543320991532,36.5166629633608));
#36740=CARTESIAN_POINT('',(24.2370701006596,26.4543320991532,36.1982357671821));
#36741=CARTESIAN_POINT('Origin',(16.1460502915689,26.4543320991532,35.0294657090004));
#36742=CARTESIAN_POINT('',(23.9621334986858,26.7543320991532,35.9909584543843));
#36743=CARTESIAN_POINT('Ctrl Pts',(24.2370701006596,26.4543320991532,36.1982357671821));
#36744=CARTESIAN_POINT('Ctrl Pts',(24.0970322987197,26.6080253707889,36.0926599396356));
#36745=CARTESIAN_POINT('Ctrl Pts',(23.9621334986858,26.7543320991532,35.9909584543843));
#36746=CARTESIAN_POINT('',(24.2791092181837,26.4543320991532,35.8564950290437));
#36747=CARTESIAN_POINT('Ctrl Pts',(23.9621334986858,26.7543320991532,35.9909584543843));
#36748=CARTESIAN_POINT('Ctrl Pts',(24.1176589685329,26.6080253707889,35.9249834092406));
#36749=CARTESIAN_POINT('Ctrl Pts',(24.2791092181837,26.4543320991532,35.8564950290437));
#36750=CARTESIAN_POINT('',(24.3054135097807,26.4543320991532,35.5348535534261));
#36751=CARTESIAN_POINT('Origin',(16.1460502915689,26.4543320991532,35.0294657090004));
#36752=CARTESIAN_POINT('',(24.0144967114075,26.7543320991532,35.3506758242353));
#36753=CARTESIAN_POINT('Ctrl Pts',(24.3054135097807,26.4543320991532,35.5348535534261));
#36754=CARTESIAN_POINT('Ctrl Pts',(24.1572362620112,26.6080253707889,35.441043401642));
#36755=CARTESIAN_POINT('Ctrl Pts',(24.0144967114075,26.7543320991532,35.3506758242353));
#36756=CARTESIAN_POINT('',(24.3194577028847,26.4543320991532,35.1908233510519));
#36757=CARTESIAN_POINT('Ctrl Pts',(24.0144967114075,26.7543320991532,35.3506758242353));
#36758=CARTESIAN_POINT('Ctrl Pts',(24.164127104422,26.6080253707889,35.2722435359911));
#36759=CARTESIAN_POINT('Ctrl Pts',(24.3194577028847,26.4543320991532,35.1908233510519));
#36760=CARTESIAN_POINT('',(24.3194577028847,26.4543320991532,34.8681080669487));
#36761=CARTESIAN_POINT('Origin',(16.1460502915689,26.4543320991532,35.0294657090004));
#36762=CARTESIAN_POINT('',(24.0144967114075,26.7543320991532,34.7082555937653));
#36763=CARTESIAN_POINT('Ctrl Pts',(24.3194577028847,26.4543320991532,34.8681080669487));
#36764=CARTESIAN_POINT('Ctrl Pts',(24.164127104422,26.6080253707889,34.7866878820095));
#36765=CARTESIAN_POINT('Ctrl Pts',(24.0144967114075,26.7543320991532,34.7082555937653));
#36766=CARTESIAN_POINT('',(24.3054135097807,26.4543320991532,34.5240778645745));
#36767=CARTESIAN_POINT('Ctrl Pts',(24.0144967114075,26.7543320991532,34.7082555937653));
#36768=CARTESIAN_POINT('Ctrl Pts',(24.1572362620112,26.6080253707889,34.6178880163586));
#36769=CARTESIAN_POINT('Ctrl Pts',(24.3054135097807,26.4543320991532,34.5240778645745));
#36770=CARTESIAN_POINT('',(24.2791092181837,26.4543320991532,34.2024363889569));
#36771=CARTESIAN_POINT('Origin',(16.1460502915689,26.4543320991532,35.0294657090004));
#36772=CARTESIAN_POINT('',(23.9621334986858,26.7543320991532,34.0679729636163));
#36773=CARTESIAN_POINT('Ctrl Pts',(24.2791092181837,26.4543320991532,34.2024363889569));
#36774=CARTESIAN_POINT('Ctrl Pts',(24.1176589685329,26.6080253707889,34.1339480087601));
#36775=CARTESIAN_POINT('Ctrl Pts',(23.9621334986858,26.7543320991532,34.0679729636163));
#36776=CARTESIAN_POINT('',(24.2370701006596,26.4543320991532,33.8606956508185));
#36777=CARTESIAN_POINT('Ctrl Pts',(23.9621334986858,26.7543320991532,34.0679729636163));
#36778=CARTESIAN_POINT('Ctrl Pts',(24.0970322987197,26.6080253707889,33.9662714783651));
#36779=CARTESIAN_POINT('Ctrl Pts',(24.2370701006596,26.4543320991532,33.8606956508185));
#36780=CARTESIAN_POINT('',(24.1846365681864,26.4543320991532,33.5422684546398));
#36781=CARTESIAN_POINT('Origin',(16.1460502915689,26.4543320991532,35.0294657090004));
#36782=CARTESIAN_POINT('',(23.8577555417836,26.7543320991532,33.4340889090527));
#36783=CARTESIAN_POINT('Ctrl Pts',(24.1846365681864,26.4543320991532,33.5422684546398));
#36784=CARTESIAN_POINT('Ctrl Pts',(24.0181410921214,26.6080253707889,33.4871676580557));
#36785=CARTESIAN_POINT('Ctrl Pts',(23.8577555417836,26.7543320991532,33.4340889090527));
#36786=CARTESIAN_POINT('',(24.1148822896334,26.4543320991532,33.2050914089663));
#36787=CARTESIAN_POINT('Ctrl Pts',(23.8577555417836,26.7543320991532,33.4340889090527));
#36788=CARTESIAN_POINT('Ctrl Pts',(23.9839158619903,26.6080253707889,33.3217303225617));
#36789=CARTESIAN_POINT('Ctrl Pts',(24.1148822896333,26.4543320991532,33.2050914089663));
#36790=CARTESIAN_POINT('',(24.0366684527916,26.4543320991532,32.8919975726802));
#36791=CARTESIAN_POINT('Origin',(16.1460502915689,26.4543320991532,35.0294657090004));
#36792=CARTESIAN_POINT('',(23.7020574587831,26.7543320991532,32.8108218238741));
#36793=CARTESIAN_POINT('Ctrl Pts',(24.0366684527915,26.4543320991532,32.8919975726802));
#36794=CARTESIAN_POINT('Ctrl Pts',(23.8662357502358,26.6080253707889,32.8506510464192));
#36795=CARTESIAN_POINT('Ctrl Pts',(23.7020574587831,26.7543320991532,32.8108218238741));
#36796=CARTESIAN_POINT('',(23.9396632164247,26.4543320991532,32.5616280770803));
#36797=CARTESIAN_POINT('Ctrl Pts',(23.7020574587831,26.7543320991532,32.8108218238741));
#36798=CARTESIAN_POINT('Ctrl Pts',(23.8186397230465,26.6080253707889,32.6885538639986));
#36799=CARTESIAN_POINT('Ctrl Pts',(23.9396632164247,26.4543320991532,32.5616280770803));
#36800=CARTESIAN_POINT('',(23.8361895753941,26.4543320991532,32.2559511885104));
#36801=CARTESIAN_POINT('Origin',(16.1460502915689,26.4543320991532,35.0294657090004));
#36802=CARTESIAN_POINT('',(23.4960753947382,26.7543320991532,32.2023194477005));
#36803=CARTESIAN_POINT('Ctrl Pts',(23.8361895753941,26.4543320991532,32.2559511885104));
#36804=CARTESIAN_POINT('Ctrl Pts',(23.6629538478638,26.6080253707889,32.2286340868829));
#36805=CARTESIAN_POINT('Ctrl Pts',(23.4960753947382,26.7543320991532,32.2023194477005));
#36806=CARTESIAN_POINT('',(23.7125789350568,26.4543320991532,31.9345877974701));
#36807=CARTESIAN_POINT('Ctrl Pts',(23.4960753947382,26.7543320991532,32.2023194477005));
#36808=CARTESIAN_POINT('Ctrl Pts',(23.6023037673244,26.6080253707889,32.0709557875407));
#36809=CARTESIAN_POINT('Ctrl Pts',(23.7125789350568,26.4543320991532,31.9345877974701));
#36810=CARTESIAN_POINT('',(23.5845340898465,26.4543320991532,31.6383620858768));
#36811=CARTESIAN_POINT('Origin',(16.1460502915689,26.4543320991532,35.0294657090004));
#36812=CARTESIAN_POINT('',(23.2411801263005,26.7543320991532,31.6126312634495));
#36813=CARTESIAN_POINT('Ctrl Pts',(23.5845340898465,26.4543320991532,31.6383620858768));
#36814=CARTESIAN_POINT('Ctrl Pts',(23.4096481925263,26.6080253707889,31.6252561996872));
#36815=CARTESIAN_POINT('Ctrl Pts',(23.2411801263005,26.7543320991532,31.6126312634495));
#36816=CARTESIAN_POINT('',(23.4351406539558,26.4543320991532,31.3281434197422));
#36817=CARTESIAN_POINT('Ctrl Pts',(23.2411801263005,26.7543320991532,31.6126312634495));
#36818=CARTESIAN_POINT('Ctrl Pts',(23.3363476749164,26.6080253707889,31.4730461064903));
#36819=CARTESIAN_POINT('Ctrl Pts',(23.4351406539558,26.4543320991532,31.3281434197422));
#36820=CARTESIAN_POINT('',(23.2833767218848,26.4543320991532,31.0433402183623));
#36821=CARTESIAN_POINT('Origin',(16.1460502915689,26.4543320991532,35.0294657090004));
#36822=CARTESIAN_POINT('',(22.9390679394266,26.7543320991532,31.0456815486958));
#36823=CARTESIAN_POINT('Ctrl Pts',(23.2833767218848,26.4543320991532,31.0433402183623));
#36824=CARTESIAN_POINT('Ctrl Pts',(23.1080044915673,26.6080253707889,31.044532765121));
#36825=CARTESIAN_POINT('Ctrl Pts',(22.9390679394266,26.7543320991532,31.0456815486958));
#36826=CARTESIAN_POINT('',(23.1091946791084,26.4543320991532,30.7463307311742));
#36827=CARTESIAN_POINT('Ctrl Pts',(22.9390679394266,26.7543320991532,31.0456815486958));
#36828=CARTESIAN_POINT('Ctrl Pts',(23.0225413397378,26.6080253707889,30.8988038111267));
#36829=CARTESIAN_POINT('Ctrl Pts',(23.1091946791084,26.4543320991532,30.7463307311742));
#36830=CARTESIAN_POINT('',(22.9347216241054,26.4543320991532,30.4748453583237));
#36831=CARTESIAN_POINT('Origin',(16.1460502915689,26.4543320991532,35.0294657090004));
#36832=CARTESIAN_POINT('',(22.5917493408753,26.7543320991532,30.5052432602507));
#36833=CARTESIAN_POINT('Ctrl Pts',(22.9347216241053,26.4543320991532,30.4748453583237));
#36834=CARTESIAN_POINT('Ctrl Pts',(22.7600301340489,26.6080253707889,30.4903284018285));
#36835=CARTESIAN_POINT('Ctrl Pts',(22.5917493408753,26.7543320991532,30.5052432602507));
#36836=CARTESIAN_POINT('',(22.7369101271998,26.4543320991532,30.193021599216));
#36837=CARTESIAN_POINT('Ctrl Pts',(22.5917493408753,26.7543320991532,30.5052432602507));
#36838=CARTESIAN_POINT('Ctrl Pts',(22.6629730911747,26.6080253707889,30.3520503891823));
#36839=CARTESIAN_POINT('Ctrl Pts',(22.7369101271998,26.4543320991532,30.193021599216));
#36840=CARTESIAN_POINT('',(22.5408890386598,26.4543320991532,29.9366607452593));
#36841=CARTESIAN_POINT('Origin',(16.1460502915689,26.4543320991532,35.0294657090004));
#36842=CARTESIAN_POINT('',(22.2015356786164,26.7543320991532,29.9949129257578));
#36843=CARTESIAN_POINT('Ctrl Pts',(22.5408890386598,26.4543320991532,29.9366607452593));
#36844=CARTESIAN_POINT('Ctrl Pts',(22.3680408319087,26.6080253707889,29.9663312484104));
#36845=CARTESIAN_POINT('Ctrl Pts',(22.2015356786164,26.7543320991532,29.9949129257578));
#36846=CARTESIAN_POINT('',(22.3207644905005,26.4543320991532,29.6718982048514));
#36847=CARTESIAN_POINT('Ctrl Pts',(22.2015356786164,26.7543320991532,29.9949129257579));
#36848=CARTESIAN_POINT('Ctrl Pts',(22.2600357965969,26.6080253707889,29.836424394472));
#36849=CARTESIAN_POINT('Ctrl Pts',(22.3207644905005,26.4543320991532,29.6718982048514));
#36850=CARTESIAN_POINT('',(22.1044998564264,26.4543320991532,29.4323679089749));
#36851=CARTESIAN_POINT('Origin',(16.1460502915689,26.4543320991532,35.0294657090004));
#36852=CARTESIAN_POINT('',(21.7710237601914,26.7543320991532,29.5180867093948));
#36853=CARTESIAN_POINT('Ctrl Pts',(22.1044998564264,26.4543320991532,29.4323679089749));
#36854=CARTESIAN_POINT('Ctrl Pts',(21.9346452092787,26.6080253707889,29.4760284194691));
#36855=CARTESIAN_POINT('Ctrl Pts',(21.7710237601914,26.7543320991532,29.5180867093948));
#36856=CARTESIAN_POINT('',(21.8635271495634,26.4543320991532,29.1864285382904));
#36857=CARTESIAN_POINT('Ctrl Pts',(21.7710237601914,26.7543320991532,29.5180867093948));
#36858=CARTESIAN_POINT('Ctrl Pts',(21.8164109372197,26.6080253707889,29.3553572329184));
#36859=CARTESIAN_POINT('Ctrl Pts',(21.8635271495634,26.4543320991532,29.1864285382904));
#36860=CARTESIAN_POINT('',(21.6284581754139,26.4543320991532,28.9653228350936));
#36861=CARTESIAN_POINT('Origin',(16.1460502915689,26.4543320991532,35.0294657090004));
#36862=CARTESIAN_POINT('',(21.303078571388,26.7543320991532,29.0779378109605));
#36863=CARTESIAN_POINT('Ctrl Pts',(21.6284581754139,26.4543320991532,28.9653228350936));
#36864=CARTESIAN_POINT('Ctrl Pts',(21.4627274425222,26.6080253707889,29.022682799437));
#36865=CARTESIAN_POINT('Ctrl Pts',(21.303078571388,26.7543320991532,29.0779378109605));
#36866=CARTESIAN_POINT('',(21.3682409434536,26.4543320991532,28.7398433200673));
#36867=CARTESIAN_POINT('Ctrl Pts',(21.303078571388,26.7543320991532,29.0779378109605));
#36868=CARTESIAN_POINT('Ctrl Pts',(21.3350507632894,26.6080253707889,28.912050327111));
#36869=CARTESIAN_POINT('Ctrl Pts',(21.3682409434536,26.4543320991532,28.7398433200673));
#36870=CARTESIAN_POINT('',(21.1159319744681,26.4543320991532,28.538633631525));
#36871=CARTESIAN_POINT('Origin',(16.1460502915689,26.4543320991532,35.0294657090004));
#36872=CARTESIAN_POINT('',(20.8008142102322,26.7543320991532,28.6773953487548));
#36873=CARTESIAN_POINT('Ctrl Pts',(21.1159319744681,26.4543320991532,28.538633631525));
#36874=CARTESIAN_POINT('Ctrl Pts',(20.9554280665162,26.6080253707889,28.6093113286187));
#36875=CARTESIAN_POINT('Ctrl Pts',(20.8008142102322,26.7543320991532,28.6773953487548));
#36876=CARTESIAN_POINT('',(20.8382019201564,26.4543320991532,28.3351145011278));
#36877=CARTESIAN_POINT('Ctrl Pts',(20.8008142102322,26.7543320991532,28.6773953487548));
#36878=CARTESIAN_POINT('Ctrl Pts',(20.8191586473445,26.6080253707889,28.5094538113677));
#36879=CARTESIAN_POINT('Ctrl Pts',(20.8382019201564,26.4543320991532,28.3351145011279));
#36880=CARTESIAN_POINT('',(20.5703320308953,26.4543320991532,28.15513984452));
#36881=CARTESIAN_POINT('Origin',(16.1460502915689,26.4543320991532,35.0294657090004));
#36882=CARTESIAN_POINT('',(20.2675731631797,26.7543320991532,28.3191248667786));
#36883=CARTESIAN_POINT('Ctrl Pts',(20.5703320308953,26.4543320991532,28.15513984452));
#36884=CARTESIAN_POINT('Ctrl Pts',(20.4161230749093,26.6080253707889,28.2386649259508));
#36885=CARTESIAN_POINT('Ctrl Pts',(20.2675731631797,26.7543320991532,28.3191248667786));
#36886=CARTESIAN_POINT('',(20.2769374019214,26.4543320991532,27.9749354849866));
#36887=CARTESIAN_POINT('Ctrl Pts',(20.2675731631797,26.7543320991532,28.3191248667786));
#36888=CARTESIAN_POINT('Ctrl Pts',(20.2721677663006,26.6080253707889,28.1502468990769));
#36889=CARTESIAN_POINT('Ctrl Pts',(20.2769374019214,26.4543320991532,27.9749354849866));
#36890=CARTESIAN_POINT('',(19.9952892223024,26.4543320991532,27.8173935619593));
#36891=CARTESIAN_POINT('Origin',(16.1460502915689,26.4543320991532,35.0294657090004));
#36892=CARTESIAN_POINT('',(19.70690406142,26.7543320991532,28.0055105959791));
#36893=CARTESIAN_POINT('Ctrl Pts',(19.9952892223024,26.4543320991532,27.8173935619593));
#36894=CARTESIAN_POINT('Ctrl Pts',(19.8484014534417,26.6080253707889,27.9132101820909));
#36895=CARTESIAN_POINT('Ctrl Pts',(19.70690406142,26.7543320991532,28.0055105959791));
#36896=CARTESIAN_POINT('',(19.6881825115154,26.4543320991532,27.6617032035706));
#36897=CARTESIAN_POINT('Ctrl Pts',(19.70690406142,26.7543320991532,28.0055105959791));
#36898=CARTESIAN_POINT('Ctrl Pts',(19.6977182542239,26.6080253707889,27.8368200529749));
#36899=CARTESIAN_POINT('Ctrl Pts',(19.6881825115154,26.4543320991532,27.6617032035706));
#36900=CARTESIAN_POINT('',(19.3946303637052,26.4543320991532,27.5276424296289));
#36901=CARTESIAN_POINT('Origin',(16.1460502915689,26.4543320991532,35.0294657090004));
#36902=CARTESIAN_POINT('',(19.1225380653215,26.7543320991532,27.7386395875858));
#36903=CARTESIAN_POINT('Ctrl Pts',(19.3946303637052,26.4543320991532,27.5276424296289));
#36904=CARTESIAN_POINT('Ctrl Pts',(19.2560412958369,26.6080253707889,27.635112944663));
#36905=CARTESIAN_POINT('Ctrl Pts',(19.1225380653215,26.7543320991532,27.7386395875858));
#36906=CARTESIAN_POINT('',(19.0758553155964,26.4543320991532,27.397502166033));
#36907=CARTESIAN_POINT('Ctrl Pts',(19.1225380653215,26.7543320991532,27.7386395875858));
#36908=CARTESIAN_POINT('Ctrl Pts',(19.0996329778396,26.6080253707889,27.5712590770108));
#36909=CARTESIAN_POINT('Ctrl Pts',(19.0758553155964,26.4543320991532,27.397502166033));
#36910=CARTESIAN_POINT('',(18.7723527407059,26.4543320991532,27.2878146935091));
#36911=CARTESIAN_POINT('Origin',(16.1460502915689,26.4543320991532,35.0294657090004));
#36912=CARTESIAN_POINT('',(18.5183640341746,26.7543320991532,27.5202878241288));
#36913=CARTESIAN_POINT('Ctrl Pts',(18.7723527407059,26.4543320991532,27.2878146935091));
#36914=CARTESIAN_POINT('Ctrl Pts',(18.642984661211,26.6080253707889,27.4062239048995));
#36915=CARTESIAN_POINT('Ctrl Pts',(18.5183640341746,26.7543320991532,27.5202878241288));
#36916=CARTESIAN_POINT('',(18.4440307506263,26.4543320991532,27.1840905866885));
#36917=CARTESIAN_POINT('Ctrl Pts',(18.5183640341746,26.7543320991532,27.5202878241288));
#36918=CARTESIAN_POINT('Ctrl Pts',(18.481892095985,26.6080253707889,27.3553312356651));
#36919=CARTESIAN_POINT('Ctrl Pts',(18.4440307506263,26.4543320991532,27.1840905866885));
#36920=CARTESIAN_POINT('',(18.132597508217,26.4543320991532,27.0995063676148));
#36921=CARTESIAN_POINT('Origin',(16.1460502915689,26.4543320991532,35.0294657090004));
#36922=CARTESIAN_POINT('',(17.8984026464748,26.7543320991532,27.3519084005685));
#36923=CARTESIAN_POINT('Ctrl Pts',(18.132597508217,26.4543320991532,27.0995063676148));
#36924=CARTESIAN_POINT('Ctrl Pts',(18.0133113403203,26.6080253707889,27.2280662815959));
#36925=CARTESIAN_POINT('Ctrl Pts',(17.8984026464748,26.7543320991532,27.3519084005685));
#36926=CARTESIAN_POINT('',(17.7969135048412,26.4543320991532,27.0228886843871));
#36927=CARTESIAN_POINT('Ctrl Pts',(17.8984026464748,26.7543320991532,27.3519084005685));
#36928=CARTESIAN_POINT('Ctrl Pts',(17.8486065723088,26.6080253707889,27.1904734930963));
#36929=CARTESIAN_POINT('Ctrl Pts',(17.7969135048412,26.4543320991532,27.0228886843871));
#36930=CARTESIAN_POINT('',(17.4796221317586,26.4543320991532,26.9639706127863));
#36931=CARTESIAN_POINT('Origin',(16.1460502915689,26.4543320991532,35.0294657090004));
#36932=CARTESIAN_POINT('',(17.266779642971,26.7543320991532,27.234621854188));
#36933=CARTESIAN_POINT('Ctrl Pts',(17.4796221317586,26.4543320991532,26.9639706127863));
#36934=CARTESIAN_POINT('Ctrl Pts',(17.3712117052266,26.6080253707889,27.1018256843414));
#36935=CARTESIAN_POINT('Ctrl Pts',(17.266779642971,26.7543320991532,27.234621854188));
#36936=CARTESIAN_POINT('',(17.1388100367451,26.4543320991532,26.9149692311924));
#36937=CARTESIAN_POINT('Ctrl Pts',(17.266779642971,26.7543320991532,27.234621854188));
#36938=CARTESIAN_POINT('Ctrl Pts',(17.2039908174863,26.6080253707889,27.0777829503817));
#36939=CARTESIAN_POINT('Ctrl Pts',(17.1388100367451,26.4543320991532,26.9149692311924));
#36940=CARTESIAN_POINT('',(16.8177720547275,26.4543320991532,26.88210939711));
#36941=CARTESIAN_POINT('Origin',(16.1460502915689,26.4543320991532,35.0294657090004));
#36942=CARTESIAN_POINT('',(16.6276983705409,26.7543320991532,27.1692087076026));
#36943=CARTESIAN_POINT('Ctrl Pts',(16.8177720547275,26.4543320991532,26.88210939711));
#36944=CARTESIAN_POINT('Ctrl Pts',(16.7209588230623,26.6080253707889,27.0283422234824));
#36945=CARTESIAN_POINT('Ctrl Pts',(16.6276983705409,26.7543320991532,27.1692087076026));
#36946=CARTESIAN_POINT('',(16.4740999163386,26.4543320991532,26.8610504132598));
#36947=CARTESIAN_POINT('Ctrl Pts',(16.6276983705409,26.7543320991532,27.1692087076026));
#36948=CARTESIAN_POINT('Ctrl Pts',(16.5523346430117,26.6080253707889,27.0180095444905));
#36949=CARTESIAN_POINT('Ctrl Pts',(16.4740999163386,26.4543320991532,26.8610504132598));
#36950=CARTESIAN_POINT('',(16.1514517801889,26.4543320991532,26.8544674934702));
#36951=CARTESIAN_POINT('Origin',(16.1460502915689,26.4543320991532,35.0294657090004));
#36952=CARTESIAN_POINT('',(16.1460502915689,26.4641465066589,26.8642801165061));
#36953=CARTESIAN_POINT('Ctrl Pts',(16.1514517801889,26.4543320991532,26.8544674934702));
#36954=CARTESIAN_POINT('Ctrl Pts',(16.1487494137305,26.4592431420195,26.8593767518666));
#36955=CARTESIAN_POINT('Ctrl Pts',(16.1460502915689,26.4641465066589,26.8642801165061));
#36956=CARTESIAN_POINT('',(16.1460502915689,26.8543320991532,27.2544657090004));
#36957=CARTESIAN_POINT('',(16.1460502915689,26.4543320991532,26.8544657090004));
#36958=CARTESIAN_POINT('Origin',(16.1460502915689,26.8543320991532,35.0294657090004));
#36959=CARTESIAN_POINT('',(15.9854118096115,26.7543320991532,27.1561042745104));
#36960=CARTESIAN_POINT('Ctrl Pts',(16.1460502915689,26.4641465066589,26.8642801165061));
#36961=CARTESIAN_POINT('Ctrl Pts',(16.0642779822078,26.6126983046876,27.0128319145347));
#36962=CARTESIAN_POINT('Ctrl Pts',(15.9854118096115,26.7543320991532,27.1561042745104));
#36963=CARTESIAN_POINT('',(15.8072066798037,26.4543320991532,26.8614910514267));
#36964=CARTESIAN_POINT('Ctrl Pts',(15.9854118096115,26.7543320991532,27.1561042745104));
#36965=CARTESIAN_POINT('Ctrl Pts',(15.8979747132105,26.6080253707889,27.0115510575768));
#36966=CARTESIAN_POINT('Ctrl Pts',(15.8072066798037,26.4543320991532,26.8614910514267));
#36967=CARTESIAN_POINT('',(15.4850955596347,26.4543320991532,26.881228854175));
#36968=CARTESIAN_POINT('Origin',(16.1460502915689,26.4543320991532,35.0294657090004));
#36969=CARTESIAN_POINT('',(15.3441942712762,26.7543320991532,27.1953957627515));
#36970=CARTESIAN_POINT('Ctrl Pts',(15.4850955596347,26.4543320991532,26.881228854175));
#36971=CARTESIAN_POINT('Ctrl Pts',(15.4133280809848,26.6080253707889,27.0412484477957));
#36972=CARTESIAN_POINT('Ctrl Pts',(15.3441942712762,26.7543320991532,27.1953957627515));
#36973=CARTESIAN_POINT('',(15.1425683915998,26.4543320991532,26.9162882133188));
#36974=CARTESIAN_POINT('Ctrl Pts',(15.3441942712762,26.7543320991532,27.1953957627515));
#36975=CARTESIAN_POINT('Ctrl Pts',(15.2452656854537,26.6080253707889,27.0584504698055));
#36976=CARTESIAN_POINT('Ctrl Pts',(15.1425683915998,26.4543320991532,26.9162882133188));
#36977=CARTESIAN_POINT('',(14.8231378837717,26.4543320991532,26.9622153867842));
#36978=CARTESIAN_POINT('Origin',(16.1460502915689,26.4543320991532,35.0294657090004));
#36979=CARTESIAN_POINT('',(14.7083129524589,26.7543320991532,27.2868216939543));
#36980=CARTESIAN_POINT('Ctrl Pts',(14.8231378837717,26.4543320991532,26.9622153867842));
#36981=CARTESIAN_POINT('Ctrl Pts',(14.7646522879161,26.6080253707889,27.1275522441746));
#36982=CARTESIAN_POINT('Ctrl Pts',(14.7083129524589,26.7543320991532,27.2868216939543));
#36983=CARTESIAN_POINT('',(14.4846081098774,26.4543320991532,27.0250772328645));
#36984=CARTESIAN_POINT('Ctrl Pts',(14.7083129524589,26.7543320991532,27.2868216939543));
#36985=CARTESIAN_POINT('Ctrl Pts',(14.5985512306315,26.6080253707889,27.1583956733261));
#36986=CARTESIAN_POINT('Ctrl Pts',(14.4846081098774,26.4543320991532,27.0250772328645));
#36987=CARTESIAN_POINT('',(14.1699839717174,26.4543320991532,27.0968881392852));
#36988=CARTESIAN_POINT('Origin',(16.1460502915689,26.4543320991532,35.0294657090004));
#36989=CARTESIAN_POINT('',(14.0819995384234,26.7543320991532,27.4297736436309));
#36990=CARTESIAN_POINT('Ctrl Pts',(14.1699839717174,26.4543320991532,27.0968881392852));
#36991=CARTESIAN_POINT('Ctrl Pts',(14.1251694706471,26.6080253707889,27.2664419709379));
#36992=CARTESIAN_POINT('Ctrl Pts',(14.0819995384234,26.7543320991532,27.4297736436309));
#36993=CARTESIAN_POINT('',(13.8377044517554,26.4543320991532,27.1871341370879));
#36994=CARTESIAN_POINT('Ctrl Pts',(14.0819995384234,26.7543320991532,27.4297736436309));
#36995=CARTESIAN_POINT('Ctrl Pts',(13.9621351267405,26.6080253707889,27.310721549299));
#36996=CARTESIAN_POINT('Ctrl Pts',(13.8377044517554,26.4543320991532,27.1871341370879));
#36997=CARTESIAN_POINT('',(13.5299804549937,26.4543320991532,27.2843508867294));
#36998=CARTESIAN_POINT('Origin',(16.1460502915689,26.4543320991532,35.0294657090004));
#36999=CARTESIAN_POINT('',(13.4694220416057,26.7543320991532,27.6233002901416));
#37000=CARTESIAN_POINT('Ctrl Pts',(13.5299804549937,26.4543320991532,27.2843508867294));
#37001=CARTESIAN_POINT('Ctrl Pts',(13.4991352818195,26.6080253707889,27.4569933398693));
#37002=CARTESIAN_POINT('Ctrl Pts',(13.4694220416057,26.7543320991532,27.6233002901416));
#37003=CARTESIAN_POINT('',(13.2061624543472,26.4543320991532,27.4013804640286));
#37004=CARTESIAN_POINT('Ctrl Pts',(13.4694220416057,26.7543320991532,27.6233002901416));
#37005=CARTESIAN_POINT('Ctrl Pts',(13.3402526179508,26.6080253707889,27.5144143941516));
#37006=CARTESIAN_POINT('Ctrl Pts',(13.2061624543472,26.4543320991532,27.4013804640286));
#37007=CARTESIAN_POINT('',(12.9073864514113,26.4543320991532,27.5233560954618));
#37008=CARTESIAN_POINT('Origin',(16.1460502915689,26.4543320991532,35.0294657090004));
#37009=CARTESIAN_POINT('',(12.874657064179,26.7543320991532,27.8661137455836));
#37010=CARTESIAN_POINT('Ctrl Pts',(12.9073864514113,26.4543320991532,27.5233560954618));
#37011=CARTESIAN_POINT('Ctrl Pts',(12.8907158756715,26.6080253707889,27.6979382630472));
#37012=CARTESIAN_POINT('Ctrl Pts',(12.874657064179,26.7543320991532,27.8661137455836));
#37013=CARTESIAN_POINT('',(12.5941849254483,26.4543320991532,27.6663904397292));
#37014=CARTESIAN_POINT('Ctrl Pts',(12.874657064179,26.7543320991532,27.8661137455836));
#37015=CARTESIAN_POINT('Ctrl Pts',(12.7370422297551,26.6080253707889,27.7681186656083));
#37016=CARTESIAN_POINT('Ctrl Pts',(12.5941849254483,26.4543320991532,27.6663904397292));
#37017=CARTESIAN_POINT('',(12.3063452213432,26.4543320991532,27.8123132252514));
#37018=CARTESIAN_POINT('Origin',(16.1460502915689,26.4543320991532,35.0294657090004));
#37019=CARTESIAN_POINT('',(12.3016626689386,26.7543320991532,28.1565981264722));
#37020=CARTESIAN_POINT('Ctrl Pts',(12.3063452213432,26.4543320991532,27.8123132252514));
#37021=CARTESIAN_POINT('Ctrl Pts',(12.3039601829689,26.6080253707889,27.9876732917611));
#37022=CARTESIAN_POINT('Ctrl Pts',(12.3016626689386,26.7543320991532,28.1565981264722));
#37023=CARTESIAN_POINT('',(12.0058444745444,26.4543320991532,27.9804004665249));
#37024=CARTESIAN_POINT('Ctrl Pts',(12.3016626689386,26.7543320991532,28.1565981264722));
#37025=CARTESIAN_POINT('Ctrl Pts',(12.1565182277639,26.6080253707889,28.0701460036008));
#37026=CARTESIAN_POINT('Ctrl Pts',(12.0058444745444,26.4543320991532,27.9804004665249));
#37027=CARTESIAN_POINT('',(11.7308565950108,26.4543320991532,28.1492993140741));
#37028=CARTESIAN_POINT('Origin',(16.1460502915689,26.4543320991532,35.0294657090004));
#37029=CARTESIAN_POINT('',(11.7542520390476,26.7543320991532,28.4928203071792));
#37030=CARTESIAN_POINT('Ctrl Pts',(11.7308565950108,26.4543320991532,28.1492993140741));
#37031=CARTESIAN_POINT('Ctrl Pts',(11.7427729660389,26.6080253707889,28.3242702871977));
#37032=CARTESIAN_POINT('Ctrl Pts',(11.7542520390476,26.7543320991532,28.4928203071792));
#37033=CARTESIAN_POINT('',(11.4450564102669,26.4543320991532,28.3413208594953));
#37034=CARTESIAN_POINT('Ctrl Pts',(11.7542520390476,26.7543320991532,28.4928203071792));
#37035=CARTESIAN_POINT('Ctrl Pts',(11.6025439034309,26.6080253707889,28.4184864660259));
#37036=CARTESIAN_POINT('Ctrl Pts',(11.4450564102669,26.4543320991532,28.3413208594953));
#37037=CARTESIAN_POINT('',(11.1847503542732,26.4543320991532,28.5320717751074));
#37038=CARTESIAN_POINT('Origin',(16.1460502915689,26.4543320991532,35.0294657090004));
#37039=CARTESIAN_POINT('',(11.2360681019313,26.7543320991532,28.8725427845647));
#37040=CARTESIAN_POINT('Ctrl Pts',(11.1847503542732,26.4543320991532,28.5320717751074));
#37041=CARTESIAN_POINT('Ctrl Pts',(11.2108888332206,26.6080253707889,28.705489251887));
#37042=CARTESIAN_POINT('Ctrl Pts',(11.2360681019313,26.7543320991532,28.8725427845647));
#37043=CARTESIAN_POINT('',(10.9155526846601,26.4543320991532,28.746749752973));
#37044=CARTESIAN_POINT('Ctrl Pts',(11.2360681019313,26.7543320991532,28.8725427845647));
#37045=CARTESIAN_POINT('Ctrl Pts',(11.0788058644852,26.6080253707889,28.8108219045781));
#37046=CARTESIAN_POINT('Ctrl Pts',(10.9155526846601,26.4543320991532,28.746749752973));
#37047=CARTESIAN_POINT('',(10.6716607460615,26.4543320991532,28.9580833207762));
#37048=CARTESIAN_POINT('Origin',(16.1460502915689,26.4543320991532,35.0294657090004));
#37049=CARTESIAN_POINT('',(10.7505592861971,26.7543320991532,29.2932385681916));
#37050=CARTESIAN_POINT('Ctrl Pts',(10.6716607460615,26.4543320991532,28.9580833207762));
#37051=CARTESIAN_POINT('Ctrl Pts',(10.7118473856633,26.6080253707889,29.1287932365158));
#37052=CARTESIAN_POINT('Ctrl Pts',(10.7505592861971,26.7543320991532,29.2932385681916));
#37053=CARTESIAN_POINT('',(10.4208570576559,26.4543320991532,29.1939890845628));
#37054=CARTESIAN_POINT('Ctrl Pts',(10.7505592861971,26.7543320991532,29.2932385681916));
#37055=CARTESIAN_POINT('Ctrl Pts',(10.5887895011652,26.6080253707889,29.2445413916448));
#37056=CARTESIAN_POINT('Ctrl Pts',(10.4208570576559,26.4543320991532,29.1939890845628));
#37057=CARTESIAN_POINT('',(10.1950022970644,26.4543320991532,29.4244989145311));
#37058=CARTESIAN_POINT('Origin',(16.1460502915689,26.4543320991532,35.0294657090004));
#37059=CARTESIAN_POINT('',(10.3009565729102,26.7543320991532,29.7521079970296));
#37060=CARTESIAN_POINT('Ctrl Pts',(10.1950022970644,26.4543320991532,29.4244989145311));
#37061=CARTESIAN_POINT('Ctrl Pts',(10.2489696618644,26.6080253707889,29.5913652229065));
#37062=CARTESIAN_POINT('Ctrl Pts',(10.3009565729103,26.7543320991532,29.7521079970296));
#37063=CARTESIAN_POINT('',(9.96426164703304,26.4543320991532,29.6800625503025));
#37064=CARTESIAN_POINT('Ctrl Pts',(10.3009565729102,26.7543320991532,29.7521079970296));
#37065=CARTESIAN_POINT('Ctrl Pts',(10.1357557915219,26.6080253707889,29.7167585955981));
#37066=CARTESIAN_POINT('Ctrl Pts',(9.96426164703304,26.4543320991532,29.6800625503025));
#37067=CARTESIAN_POINT('',(9.75794709061692,26.4543320991532,29.9282146375487));
#37068=CARTESIAN_POINT('Origin',(16.1460502915689,26.4543320991532,35.0294657090004));
#37069=CARTESIAN_POINT('',(9.89025199394849,26.7543320991532,30.2460973707382));
#37070=CARTESIAN_POINT('Ctrl Pts',(9.75794709061692,26.4543320991532,29.9282146375487));
#37071=CARTESIAN_POINT('Ctrl Pts',(9.82533603670637,26.6080253707889,30.0901268708088));
#37072=CARTESIAN_POINT('Ctrl Pts',(9.89025199394849,26.7543320991532,30.2460973707382));
#37073=CARTESIAN_POINT('',(9.5488050199162,26.4543320991532,30.2017354114738));
#37074=CARTESIAN_POINT('Ctrl Pts',(9.89025199394848,26.7543320991532,30.2460973707382));
#37075=CARTESIAN_POINT('Ctrl Pts',(9.7227196001476,26.6080253707889,30.2243309888561));
#37076=CARTESIAN_POINT('Ctrl Pts',(9.5488050199162,26.4543320991532,30.2017354114738));
#37077=CARTESIAN_POINT('',(9.36340365700895,26.4543320991532,30.4658783447997));
#37078=CARTESIAN_POINT('Origin',(16.1460502915689,26.4543320991532,35.0294657090004));
#37079=CARTESIAN_POINT('',(9.52117872052333,26.7543320991532,30.7719192715376));
#37080=CARTESIAN_POINT('Ctrl Pts',(9.36340365700896,26.4543320991532,30.4658783447997));
#37081=CARTESIAN_POINT('Ctrl Pts',(9.44376572207002,26.6080253707889,30.6217590037456));
#37082=CARTESIAN_POINT('Ctrl Pts',(9.52117872052333,26.7543320991532,30.7719192715376));
#37083=CARTESIAN_POINT('',(9.17725197161336,26.4543320991532,30.7555360212558));
#37084=CARTESIAN_POINT('Ctrl Pts',(9.52117872052333,26.7543320991532,30.7719192715376));
#37085=CARTESIAN_POINT('Ctrl Pts',(9.35242961474975,26.6080253707889,30.7638807608853));
#37086=CARTESIAN_POINT('Ctrl Pts',(9.17725197161336,26.4543320991532,30.7555360212558));
#37087=CARTESIAN_POINT('',(9.01399761769606,26.4543320991532,31.0339119730205));
#37088=CARTESIAN_POINT('Origin',(16.1460502915689,26.4543320991532,35.0294657090004));
#37089=CARTESIAN_POINT('',(9.19619287437661,26.7543320991532,31.3260744414326));
#37090=CARTESIAN_POINT('Ctrl Pts',(9.01399761769606,26.4543320991532,31.0339119730205));
#37091=CARTESIAN_POINT('Ctrl Pts',(9.10679800544456,26.6080253707889,31.1827236975856));
#37092=CARTESIAN_POINT('Ctrl Pts',(9.19619287437661,26.7543320991532,31.3260744414327));
#37093=CARTESIAN_POINT('',(8.85207512635903,26.4543320991532,31.3377789279609));
#37094=CARTESIAN_POINT('Ctrl Pts',(9.19619287437661,26.7543320991532,31.3260744414326));
#37095=CARTESIAN_POINT('Ctrl Pts',(9.02735005408761,26.6080253707889,31.3318172969722));
#37096=CARTESIAN_POINT('Ctrl Pts',(8.85207512635903,26.4543320991532,31.3377789279609));
#37097=CARTESIAN_POINT('',(8.71205421222193,26.4543320991532,31.6285353521343));
#37098=CARTESIAN_POINT('Origin',(16.1460502915689,26.4543320991532,35.0294657090004));
#37099=CARTESIAN_POINT('',(8.91745718269554,26.7543320991532,31.9048750691968));
#37100=CARTESIAN_POINT('Ctrl Pts',(8.71205421222193,26.4543320991532,31.6285353521343));
#37101=CARTESIAN_POINT('Ctrl Pts',(8.81667535138839,26.6080253707889,31.7692878248437));
#37102=CARTESIAN_POINT('Ctrl Pts',(8.91745718269554,26.7543320991532,31.9048750691968));
#37103=CARTESIAN_POINT('',(8.57543848240798,26.4543320991532,31.9445894011085));
#37104=CARTESIAN_POINT('Ctrl Pts',(8.91745718269554,26.7543320991532,31.9048750691968));
#37105=CARTESIAN_POINT('Ctrl Pts',(8.74964426900305,26.6080253707889,31.9243610731722));
#37106=CARTESIAN_POINT('Ctrl Pts',(8.57543848240799,26.4543320991532,31.9445894011085));
#37107=CARTESIAN_POINT('',(8.45958282413283,26.4543320991532,32.245791361659));
#37108=CARTESIAN_POINT('Origin',(16.1460502915689,26.4543320991532,35.0294657090004));
#37109=CARTESIAN_POINT('',(8.68682658552011,26.7543320991532,32.5044693321477));
#37110=CARTESIAN_POINT('Ctrl Pts',(8.45958282413283,26.4543320991532,32.245791361659));
#37111=CARTESIAN_POINT('Ctrl Pts',(8.57532847829738,26.6080253707889,32.3775478980294));
#37112=CARTESIAN_POINT('Ctrl Pts',(8.68682658552011,26.7543320991532,32.5044693321477));
#37113=CARTESIAN_POINT('',(8.34918301098387,26.4543320991532,32.5719292171162));
#37114=CARTESIAN_POINT('Ctrl Pts',(8.68682658552011,26.7543320991532,32.5044693321477));
#37115=CARTESIAN_POINT('Ctrl Pts',(8.52116034567757,26.6080253707889,32.5375688084173));
#37116=CARTESIAN_POINT('Ctrl Pts',(8.34918301098388,26.4543320991532,32.5719292171162));
#37117=CARTESIAN_POINT('',(8.25826360886166,26.4543320991532,32.8815722646913));
#37118=CARTESIAN_POINT('Origin',(16.1460502915689,26.4543320991532,35.0294657090004));
#37119=CARTESIAN_POINT('',(8.50583589142315,26.7543320991532,33.1208670293914));
#37120=CARTESIAN_POINT('Ctrl Pts',(8.25826360886166,26.4543320991532,32.8815722646913));
#37121=CARTESIAN_POINT('Ctrl Pts',(8.38436350979251,26.6080253707889,33.0034560467115));
#37122=CARTESIAN_POINT('Ctrl Pts',(8.50583589142315,26.7543320991532,33.1208670293914));
#37123=CARTESIAN_POINT('',(8.17481440491951,26.4543320991532,33.2156235330125));
#37124=CARTESIAN_POINT('Ctrl Pts',(8.50583589142315,26.7543320991532,33.1208670293914));
#37125=CARTESIAN_POINT('Ctrl Pts',(8.3434188069237,26.6080253707889,33.1673597064018));
#37126=CARTESIAN_POINT('Ctrl Pts',(8.17481440491951,26.4543320991532,33.2156235330125));
#37127=CARTESIAN_POINT('',(8.1094363125707,26.4543320991532,33.5316470442181));
#37128=CARTESIAN_POINT('Origin',(16.1460502915689,26.4543320991532,35.0294657090004));
#37129=CARTESIAN_POINT('',(8.37568956361252,26.7543320991532,33.7499661359513));
#37130=CARTESIAN_POINT('Ctrl Pts',(8.10943631257071,26.4543320991532,33.5316470442181));
#37131=CARTESIAN_POINT('Ctrl Pts',(8.24505128623219,26.6080253707889,33.642846955428));
#37132=CARTESIAN_POINT('Ctrl Pts',(8.37568956361252,26.7543320991532,33.7499661359513));
#37133=CARTESIAN_POINT('',(8.05349305851944,26.4543320991532,33.8713886693271));
#37134=CARTESIAN_POINT('Ctrl Pts',(8.37568956361252,26.7543320991532,33.7499661359513));
#37135=CARTESIAN_POINT('Ctrl Pts',(8.21760249335657,26.6080253707889,33.8095426126077));
#37136=CARTESIAN_POINT('Ctrl Pts',(8.05349305851944,26.4543320991532,33.8713886693271));
#37137=CARTESIAN_POINT('',(8.01409135636201,26.4543320991532,34.1916895598362));
#37138=CARTESIAN_POINT('Origin',(16.1460502915689,26.4543320991532,35.0294657090004));
#37139=CARTESIAN_POINT('',(8.29725370442715,26.7543320991532,34.3875801010673));
#37140=CARTESIAN_POINT('Ctrl Pts',(8.01409135636201,26.4543320991532,34.1916895598362));
#37141=CARTESIAN_POINT('Ctrl Pts',(8.1583189074793,26.6080253707889,34.2914655831736));
#37142=CARTESIAN_POINT('Ctrl Pts',(8.29725370442715,26.7543320991532,34.3875801010673));
#37143=CARTESIAN_POINT('',(7.98602634532736,26.4543320991532,34.5348606172715));
#37144=CARTESIAN_POINT('Ctrl Pts',(8.29725370442715,26.7543320991532,34.3875801010674));
#37145=CARTESIAN_POINT('Ctrl Pts',(8.14454869178473,26.6080253707889,34.4598439057469));
#37146=CARTESIAN_POINT('Ctrl Pts',(7.98602634532737,26.4543320991532,34.5348606172715));
#37147=CARTESIAN_POINT('',(7.97286324518834,26.4543320991532,34.8573073375037));
#37148=CARTESIAN_POINT('Origin',(16.1460502915689,26.4543320991532,35.0294657090004));
#37149=CARTESIAN_POINT('',(8.27105029156894,26.7543320991532,35.0294657090004));
#37150=CARTESIAN_POINT('Ctrl Pts',(7.97286324518834,26.4543320991532,34.8573073375037));
#37151=CARTESIAN_POINT('Ctrl Pts',(8.12474356320462,26.6080253707889,34.944995479995));
#37152=CARTESIAN_POINT('Ctrl Pts',(8.27105029156894,26.7543320991532,35.0294657090004));
#37153=CARTESIAN_POINT('',(7.97286324518834,26.4543320991532,35.2016240804971));
#37154=CARTESIAN_POINT('Ctrl Pts',(8.27105029156894,26.7543320991532,35.0294657090004));
#37155=CARTESIAN_POINT('Ctrl Pts',(8.12474356320462,26.6080253707889,35.1139359380058));
#37156=CARTESIAN_POINT('Ctrl Pts',(7.97286324518834,26.4543320991532,35.2016240804971));
#37157=CARTESIAN_POINT('',(7.98602634532737,26.4543320991532,35.5240708007294));
#37158=CARTESIAN_POINT('Origin',(16.1460502915689,26.4543320991532,35.0294657090004));
#37159=CARTESIAN_POINT('',(8.29725370442716,26.7543320991532,35.6713513169335));
#37160=CARTESIAN_POINT('Ctrl Pts',(7.98602634532737,26.4543320991532,35.5240708007294));
#37161=CARTESIAN_POINT('Ctrl Pts',(8.14454869178474,26.6080253707889,35.5990875122539));
#37162=CARTESIAN_POINT('Ctrl Pts',(8.29725370442716,26.7543320991532,35.6713513169335));
#37163=CARTESIAN_POINT('',(8.01409135636202,26.4543320991532,35.8672418581646));
#37164=CARTESIAN_POINT('Ctrl Pts',(8.29725370442716,26.7543320991532,35.6713513169335));
#37165=CARTESIAN_POINT('Ctrl Pts',(8.15831890747931,26.6080253707889,35.7674658348273));
#37166=CARTESIAN_POINT('Ctrl Pts',(8.01409135636202,26.4543320991532,35.8672418581646));
#37167=CARTESIAN_POINT('',(8.05349305851946,26.4543320991532,36.1875427486737));
#37168=CARTESIAN_POINT('Origin',(16.1460502915689,26.4543320991532,35.0294657090004));
#37169=CARTESIAN_POINT('',(8.37568956361253,26.7543320991532,36.3089652820495));
#37170=CARTESIAN_POINT('Ctrl Pts',(8.05349305851946,26.4543320991532,36.1875427486737));
#37171=CARTESIAN_POINT('Ctrl Pts',(8.21760249335659,26.6080253707889,36.2493888053931));
#37172=CARTESIAN_POINT('Ctrl Pts',(8.37568956361253,26.7543320991532,36.3089652820495));
#37173=CARTESIAN_POINT('',(8.10943631257072,26.4543320991532,36.5272843737828));
#37174=CARTESIAN_POINT('Ctrl Pts',(8.37568956361254,26.7543320991532,36.3089652820495));
#37175=CARTESIAN_POINT('Ctrl Pts',(8.24505128623221,26.6080253707889,36.4160844625728));
#37176=CARTESIAN_POINT('Ctrl Pts',(8.10943631257073,26.4543320991532,36.5272843737828));
#37177=CARTESIAN_POINT('',(8.17481440491953,26.4543320991532,36.8433078849883));
#37178=CARTESIAN_POINT('Origin',(16.1460502915689,26.4543320991532,35.0294657090004));
#37179=CARTESIAN_POINT('',(8.50583589142318,26.7543320991532,36.9380643886094));
#37180=CARTESIAN_POINT('Ctrl Pts',(8.17481440491953,26.4543320991532,36.8433078849883));
#37181=CARTESIAN_POINT('Ctrl Pts',(8.34341880692373,26.6080253707889,36.8915717115991));
#37182=CARTESIAN_POINT('Ctrl Pts',(8.50583589142318,26.7543320991532,36.9380643886094));
#37183=CARTESIAN_POINT('',(8.25826360886169,26.4543320991532,37.1773591533095));
#37184=CARTESIAN_POINT('Ctrl Pts',(8.50583589142317,26.7543320991532,36.9380643886094));
#37185=CARTESIAN_POINT('Ctrl Pts',(8.38436350979254,26.6080253707889,37.0554753712894));
#37186=CARTESIAN_POINT('Ctrl Pts',(8.25826360886169,26.4543320991532,37.1773591533095));
#37187=CARTESIAN_POINT('',(8.34918301098391,26.4543320991532,37.4870022008846));
#37188=CARTESIAN_POINT('Origin',(16.1460502915689,26.4543320991532,35.0294657090004));
#37189=CARTESIAN_POINT('',(8.68682658552014,26.7543320991532,37.5544620858532));
#37190=CARTESIAN_POINT('Ctrl Pts',(8.34918301098391,26.4543320991532,37.4870022008846));
#37191=CARTESIAN_POINT('Ctrl Pts',(8.5211603456776,26.6080253707889,37.5213626095835));
#37192=CARTESIAN_POINT('Ctrl Pts',(8.68682658552014,26.7543320991532,37.5544620858532));
#37193=CARTESIAN_POINT('',(8.45958282413287,26.4543320991532,37.8131400563419));
#37194=CARTESIAN_POINT('Ctrl Pts',(8.68682658552014,26.7543320991532,37.5544620858532));
#37195=CARTESIAN_POINT('Ctrl Pts',(8.57532847829741,26.6080253707889,37.6813835199714));
#37196=CARTESIAN_POINT('Ctrl Pts',(8.45958282413287,26.4543320991532,37.8131400563418));
#37197=CARTESIAN_POINT('',(8.57543848240802,26.4543320991532,38.1143420168924));
#37198=CARTESIAN_POINT('Origin',(16.1460502915689,26.4543320991532,35.0294657090004));
#37199=CARTESIAN_POINT('',(8.91745718269558,26.7543320991532,38.154056348804));
#37200=CARTESIAN_POINT('Ctrl Pts',(8.57543848240803,26.4543320991532,38.1143420168924));
#37201=CARTESIAN_POINT('Ctrl Pts',(8.74964426900309,26.6080253707889,38.1345703448287));
#37202=CARTESIAN_POINT('Ctrl Pts',(8.91745718269558,26.7543320991532,38.154056348804));
#37203=CARTESIAN_POINT('',(8.71205421222197,26.4543320991532,38.4303960658666));
#37204=CARTESIAN_POINT('Ctrl Pts',(8.91745718269558,26.7543320991532,38.154056348804));
#37205=CARTESIAN_POINT('Ctrl Pts',(8.81667535138844,26.6080253707889,38.2896435931571));
#37206=CARTESIAN_POINT('Ctrl Pts',(8.71205421222198,26.4543320991532,38.4303960658666));
#37207=CARTESIAN_POINT('',(8.85207512635908,26.4543320991532,38.7211524900399));
#37208=CARTESIAN_POINT('Origin',(16.1460502915689,26.4543320991532,35.0294657090004));
#37209=CARTESIAN_POINT('',(9.19619287437666,26.7543320991532,38.7328569765682));
#37210=CARTESIAN_POINT('Ctrl Pts',(8.85207512635908,26.4543320991532,38.7211524900399));
#37211=CARTESIAN_POINT('Ctrl Pts',(9.02735005408766,26.6080253707889,38.7271141210286));
#37212=CARTESIAN_POINT('Ctrl Pts',(9.19619287437666,26.7543320991532,38.7328569765682));
#37213=CARTESIAN_POINT('',(9.01399761769611,26.4543320991532,39.0250194449803));
#37214=CARTESIAN_POINT('Ctrl Pts',(9.19619287437666,26.7543320991532,38.7328569765682));
#37215=CARTESIAN_POINT('Ctrl Pts',(9.10679800544461,26.6080253707889,38.8762077204153));
#37216=CARTESIAN_POINT('Ctrl Pts',(9.01399761769611,26.4543320991532,39.0250194449803));
#37217=CARTESIAN_POINT('',(9.17725197161342,26.4543320991532,39.303395396745));
#37218=CARTESIAN_POINT('Origin',(16.1460502915689,26.4543320991532,35.0294657090004));
#37219=CARTESIAN_POINT('',(9.52117872052339,26.7543320991532,39.2870121464632));
#37220=CARTESIAN_POINT('Ctrl Pts',(9.17725197161342,26.4543320991532,39.303395396745));
#37221=CARTESIAN_POINT('Ctrl Pts',(9.3524296147498,26.6080253707889,39.2950506571155));
#37222=CARTESIAN_POINT('Ctrl Pts',(9.52117872052339,26.7543320991532,39.2870121464632));
#37223=CARTESIAN_POINT('',(9.36340365700901,26.4543320991532,39.5930530732011));
#37224=CARTESIAN_POINT('Ctrl Pts',(9.52117872052339,26.7543320991532,39.2870121464632));
#37225=CARTESIAN_POINT('Ctrl Pts',(9.44376572207008,26.6080253707889,39.4371724142552));
#37226=CARTESIAN_POINT('Ctrl Pts',(9.36340365700902,26.4543320991532,39.5930530732011));
#37227=CARTESIAN_POINT('',(9.54880501991626,26.4543320991532,39.857196006527));
#37228=CARTESIAN_POINT('Origin',(16.1460502915689,26.4543320991532,35.0294657090004));
#37229=CARTESIAN_POINT('',(9.89025199394856,26.7543320991532,39.8128340472626));
#37230=CARTESIAN_POINT('Ctrl Pts',(9.54880501991627,26.4543320991532,39.857196006527));
#37231=CARTESIAN_POINT('Ctrl Pts',(9.72271960014766,26.6080253707889,39.8346004291447));
#37232=CARTESIAN_POINT('Ctrl Pts',(9.89025199394855,26.7543320991532,39.8128340472626));
#37233=CARTESIAN_POINT('',(9.75794709061698,26.4543320991532,40.1307167804521));
#37234=CARTESIAN_POINT('Ctrl Pts',(9.89025199394855,26.7543320991532,39.8128340472626));
#37235=CARTESIAN_POINT('Ctrl Pts',(9.82533603670642,26.6080253707889,39.968804547192));
#37236=CARTESIAN_POINT('Ctrl Pts',(9.75794709061698,26.4543320991532,40.1307167804521));
#37237=CARTESIAN_POINT('',(9.96426164703311,26.4543320991532,40.3788688676983));
#37238=CARTESIAN_POINT('Origin',(16.1460502915689,26.4543320991532,35.0294657090004));
#37239=CARTESIAN_POINT('',(10.3009565729103,26.7543320991532,40.3068234209711));
#37240=CARTESIAN_POINT('Ctrl Pts',(9.96426164703311,26.4543320991532,40.3788688676983));
#37241=CARTESIAN_POINT('Ctrl Pts',(10.135755791522,26.6080253707889,40.3421728224027));
#37242=CARTESIAN_POINT('Ctrl Pts',(10.3009565729103,26.7543320991532,40.3068234209711));
#37243=CARTESIAN_POINT('',(10.1950022970645,26.4543320991532,40.6344325034697));
#37244=CARTESIAN_POINT('Ctrl Pts',(10.3009565729103,26.7543320991532,40.3068234209712));
#37245=CARTESIAN_POINT('Ctrl Pts',(10.2489696618645,26.6080253707889,40.4675661950943));
#37246=CARTESIAN_POINT('Ctrl Pts',(10.1950022970645,26.4543320991532,40.6344325034697));
#37247=CARTESIAN_POINT('',(10.420857057656,26.4543320991532,40.864942333438));
#37248=CARTESIAN_POINT('Origin',(16.1460502915689,26.4543320991532,35.0294657090004));
#37249=CARTESIAN_POINT('',(10.7505592861972,26.7543320991532,40.7656928498092));
#37250=CARTESIAN_POINT('Ctrl Pts',(10.420857057656,26.4543320991532,40.864942333438));
#37251=CARTESIAN_POINT('Ctrl Pts',(10.5887895011653,26.6080253707889,40.8143900263561));
#37252=CARTESIAN_POINT('Ctrl Pts',(10.7505592861972,26.7543320991532,40.7656928498092));
#37253=CARTESIAN_POINT('',(10.6716607460615,26.4543320991532,41.1008480972246));
#37254=CARTESIAN_POINT('Ctrl Pts',(10.7505592861972,26.7543320991532,40.7656928498093));
#37255=CARTESIAN_POINT('Ctrl Pts',(10.7118473856633,26.6080253707889,40.930138181485));
#37256=CARTESIAN_POINT('Ctrl Pts',(10.6716607460615,26.4543320991532,41.1008480972246));
#37257=CARTESIAN_POINT('',(10.9155526846602,26.4543320991532,41.3121816650278));
#37258=CARTESIAN_POINT('Origin',(16.1460502915689,26.4543320991532,35.0294657090004));
#37259=CARTESIAN_POINT('',(11.2360681019314,26.7543320991532,41.1863886334361));
#37260=CARTESIAN_POINT('Ctrl Pts',(10.9155526846602,26.4543320991532,41.3121816650278));
#37261=CARTESIAN_POINT('Ctrl Pts',(11.0788058644853,26.6080253707889,41.2481095134227));
#37262=CARTESIAN_POINT('Ctrl Pts',(11.2360681019314,26.7543320991532,41.1863886334361));
#37263=CARTESIAN_POINT('',(11.1847503542733,26.4543320991532,41.5268596428934));
#37264=CARTESIAN_POINT('Ctrl Pts',(11.2360681019314,26.7543320991532,41.1863886334361));
#37265=CARTESIAN_POINT('Ctrl Pts',(11.2108888332207,26.6080253707889,41.3534421661138));
#37266=CARTESIAN_POINT('Ctrl Pts',(11.1847503542733,26.4543320991532,41.5268596428934));
#37267=CARTESIAN_POINT('',(11.445056410267,26.4543320991532,41.7176105585055));
#37268=CARTESIAN_POINT('Origin',(16.1460502915689,26.4543320991532,35.0294657090004));
#37269=CARTESIAN_POINT('',(11.7542520390477,26.7543320991532,41.5661111108216));
#37270=CARTESIAN_POINT('Ctrl Pts',(11.445056410267,26.4543320991532,41.7176105585055));
#37271=CARTESIAN_POINT('Ctrl Pts',(11.602543903431,26.6080253707889,41.6404449519749));
#37272=CARTESIAN_POINT('Ctrl Pts',(11.7542520390477,26.7543320991532,41.5661111108216));
#37273=CARTESIAN_POINT('',(11.7308565950109,26.4543320991532,41.9096321039267));
#37274=CARTESIAN_POINT('Ctrl Pts',(11.7542520390477,26.7543320991532,41.5661111108216));
#37275=CARTESIAN_POINT('Ctrl Pts',(11.742772966039,26.6080253707889,41.7346611308031));
#37276=CARTESIAN_POINT('Ctrl Pts',(11.7308565950109,26.4543320991532,41.9096321039267));
#37277=CARTESIAN_POINT('',(12.0058444745445,26.4543320991532,42.0785309514759));
#37278=CARTESIAN_POINT('Origin',(16.1460502915689,26.4543320991532,35.0294657090004));
#37279=CARTESIAN_POINT('',(12.3016626689387,26.7543320991532,41.9023332915286));
#37280=CARTESIAN_POINT('Ctrl Pts',(12.0058444745445,26.4543320991532,42.0785309514759));
#37281=CARTESIAN_POINT('Ctrl Pts',(12.156518227764,26.6080253707889,41.9887854144));
#37282=CARTESIAN_POINT('Ctrl Pts',(12.3016626689387,26.7543320991532,41.9023332915286));
#37283=CARTESIAN_POINT('',(12.3063452213433,26.4543320991532,42.2466181927493));
#37284=CARTESIAN_POINT('Ctrl Pts',(12.3016626689387,26.7543320991532,41.9023332915286));
#37285=CARTESIAN_POINT('Ctrl Pts',(12.303960182969,26.6080253707889,42.0712581262397));
#37286=CARTESIAN_POINT('Ctrl Pts',(12.3063452213433,26.4543320991532,42.2466181927493));
#37287=CARTESIAN_POINT('',(12.5941849254484,26.4543320991532,42.3925409782716));
#37288=CARTESIAN_POINT('Origin',(16.1460502915689,26.4543320991532,35.0294657090004));
#37289=CARTESIAN_POINT('',(12.8746570641791,26.7543320991532,42.1928176724172));
#37290=CARTESIAN_POINT('Ctrl Pts',(12.5941849254484,26.4543320991532,42.3925409782716));
#37291=CARTESIAN_POINT('Ctrl Pts',(12.7370422297551,26.6080253707889,42.2908127523925));
#37292=CARTESIAN_POINT('Ctrl Pts',(12.8746570641791,26.7543320991532,42.1928176724172));
#37293=CARTESIAN_POINT('',(12.9073864514114,26.4543320991532,42.5355753225389));
#37294=CARTESIAN_POINT('Ctrl Pts',(12.8746570641791,26.7543320991532,42.1928176724172));
#37295=CARTESIAN_POINT('Ctrl Pts',(12.8907158756716,26.6080253707889,42.3609931549536));
#37296=CARTESIAN_POINT('Ctrl Pts',(12.9073864514114,26.4543320991532,42.5355753225389));
#37297=CARTESIAN_POINT('',(13.2061624543473,26.4543320991532,42.6575509539721));
#37298=CARTESIAN_POINT('Origin',(16.1460502915689,26.4543320991532,35.0294657090004));
#37299=CARTESIAN_POINT('',(13.4694220416058,26.7543320991532,42.4356311278591));
#37300=CARTESIAN_POINT('Ctrl Pts',(13.2061624543473,26.4543320991532,42.6575509539721));
#37301=CARTESIAN_POINT('Ctrl Pts',(13.3402526179509,26.6080253707889,42.5445170238492));
#37302=CARTESIAN_POINT('Ctrl Pts',(13.4694220416058,26.7543320991532,42.4356311278591));
#37303=CARTESIAN_POINT('',(13.5299804549939,26.4543320991532,42.7745805312714));
#37304=CARTESIAN_POINT('Ctrl Pts',(13.4694220416058,26.7543320991532,42.4356311278591));
#37305=CARTESIAN_POINT('Ctrl Pts',(13.4991352818196,26.6080253707889,42.6019380781315));
#37306=CARTESIAN_POINT('Ctrl Pts',(13.5299804549939,26.4543320991532,42.7745805312714));
#37307=CARTESIAN_POINT('',(13.8377044517555,26.4543320991532,42.8717972809129));
#37308=CARTESIAN_POINT('Origin',(16.1460502915689,26.4543320991532,35.0294657090004));
#37309=CARTESIAN_POINT('',(14.0819995384235,26.7543320991532,42.6291577743698));
#37310=CARTESIAN_POINT('Ctrl Pts',(13.8377044517555,26.4543320991532,42.8717972809129));
#37311=CARTESIAN_POINT('Ctrl Pts',(13.9621351267406,26.6080253707889,42.7482098687017));
#37312=CARTESIAN_POINT('Ctrl Pts',(14.0819995384235,26.7543320991532,42.6291577743698));
#37313=CARTESIAN_POINT('',(14.1699839717175,26.4543320991532,42.9620432787156));
#37314=CARTESIAN_POINT('Ctrl Pts',(14.0819995384235,26.7543320991532,42.6291577743698));
#37315=CARTESIAN_POINT('Ctrl Pts',(14.1251694706472,26.6080253707889,42.7924894470628));
#37316=CARTESIAN_POINT('Ctrl Pts',(14.1699839717175,26.4543320991532,42.9620432787156));
#37317=CARTESIAN_POINT('',(14.4846081098775,26.4543320991532,43.0338541851362));
#37318=CARTESIAN_POINT('Origin',(16.1460502915689,26.4543320991532,35.0294657090004));
#37319=CARTESIAN_POINT('',(14.708312952459,26.7543320991532,42.7721097240465));
#37320=CARTESIAN_POINT('Ctrl Pts',(14.4846081098775,26.4543320991532,43.0338541851362));
#37321=CARTESIAN_POINT('Ctrl Pts',(14.5985512306316,26.6080253707889,42.9005357446746));
#37322=CARTESIAN_POINT('Ctrl Pts',(14.708312952459,26.7543320991532,42.7721097240465));
#37323=CARTESIAN_POINT('',(14.8231378837718,26.4543320991532,43.0967160312165));
#37324=CARTESIAN_POINT('Ctrl Pts',(14.708312952459,26.7543320991532,42.7721097240464));
#37325=CARTESIAN_POINT('Ctrl Pts',(14.7646522879162,26.6080253707889,42.9313791738261));
#37326=CARTESIAN_POINT('Ctrl Pts',(14.8231378837718,26.4543320991532,43.0967160312165));
#37327=CARTESIAN_POINT('',(15.1425683915999,26.4543320991532,43.142643204682));
#37328=CARTESIAN_POINT('Origin',(16.1460502915689,26.4543320991532,35.0294657090004));
#37329=CARTESIAN_POINT('',(15.3441942712763,26.7543320991532,42.8635356552493));
#37330=CARTESIAN_POINT('Ctrl Pts',(15.1425683915999,26.4543320991532,43.142643204682));
#37331=CARTESIAN_POINT('Ctrl Pts',(15.2452656854538,26.6080253707889,43.0004809481952));
#37332=CARTESIAN_POINT('Ctrl Pts',(15.3441942712763,26.7543320991532,42.8635356552493));
#37333=CARTESIAN_POINT('',(15.4850955596348,26.4543320991532,43.1777025638257));
#37334=CARTESIAN_POINT('Ctrl Pts',(15.3441942712763,26.7543320991532,42.8635356552493));
#37335=CARTESIAN_POINT('Ctrl Pts',(15.4133280809849,26.6080253707889,43.017682970205));
#37336=CARTESIAN_POINT('Ctrl Pts',(15.4850955596348,26.4543320991532,43.1777025638257));
#37337=CARTESIAN_POINT('',(15.8072066798038,26.4543320991532,43.197440366574));
#37338=CARTESIAN_POINT('Origin',(16.1460502915689,26.4543320991532,35.0294657090004));
#37339=CARTESIAN_POINT('Ctrl Pts',(15.8072066798038,26.4543320991532,43.197440366574));
#37340=CARTESIAN_POINT('Ctrl Pts',(15.8979747132106,26.6080253707889,43.0473803604239));
#37341=CARTESIAN_POINT('Ctrl Pts',(15.9854118096116,26.7543320991532,42.9028271434904));
#37342=CARTESIAN_POINT('Origin',(16.1460502915689,23.7543320991532,35.0294657090004));
#37343=CARTESIAN_POINT('',(16.1514517801889,23.7543320991532,26.8544674934702));
#37344=CARTESIAN_POINT('',(15.9854118096115,23.4543320991532,27.1561042745104));
#37345=CARTESIAN_POINT('Ctrl Pts',(16.1514517801889,23.7543320991532,26.8544674934702));
#37346=CARTESIAN_POINT('Ctrl Pts',(16.0668800194743,23.6006388275175,27.0081049193271));
#37347=CARTESIAN_POINT('Ctrl Pts',(15.9854118096115,23.4543320991532,27.1561042745104));
#37348=CARTESIAN_POINT('',(16.4740999163386,23.7543320991532,26.8610504132598));
#37349=CARTESIAN_POINT('Origin',(16.1460502915689,23.7543320991532,35.0294657090004));
#37350=CARTESIAN_POINT('',(16.6276983705409,23.4543320991532,27.1692087076026));
#37351=CARTESIAN_POINT('Ctrl Pts',(16.6276983705409,23.4543320991532,27.1692087076026));
#37352=CARTESIAN_POINT('Ctrl Pts',(16.5523346430117,23.6006388275175,27.0180095444905));
#37353=CARTESIAN_POINT('Ctrl Pts',(16.4740999163386,23.7543320991532,26.8610504132598));
#37354=CARTESIAN_POINT('',(16.8177720547275,23.7543320991532,26.88210939711));
#37355=CARTESIAN_POINT('Ctrl Pts',(16.8177720547275,23.7543320991532,26.88210939711));
#37356=CARTESIAN_POINT('Ctrl Pts',(16.7209588230624,23.6006388275175,27.0283422234824));
#37357=CARTESIAN_POINT('Ctrl Pts',(16.6276983705409,23.4543320991532,27.1692087076026));
#37358=CARTESIAN_POINT('',(17.1388100367451,23.7543320991532,26.9149692311924));
#37359=CARTESIAN_POINT('Origin',(16.1460502915689,23.7543320991532,35.0294657090004));
#37360=CARTESIAN_POINT('',(17.266779642971,23.4543320991532,27.234621854188));
#37361=CARTESIAN_POINT('Ctrl Pts',(17.266779642971,23.4543320991532,27.234621854188));
#37362=CARTESIAN_POINT('Ctrl Pts',(17.2039908174863,23.6006388275175,27.0777829503818));
#37363=CARTESIAN_POINT('Ctrl Pts',(17.1388100367451,23.7543320991532,26.9149692311924));
#37364=CARTESIAN_POINT('',(17.4796221317586,23.7543320991532,26.9639706127863));
#37365=CARTESIAN_POINT('Ctrl Pts',(17.4796221317586,23.7543320991532,26.9639706127863));
#37366=CARTESIAN_POINT('Ctrl Pts',(17.3712117052266,23.6006388275175,27.1018256843414));
#37367=CARTESIAN_POINT('Ctrl Pts',(17.266779642971,23.4543320991532,27.234621854188));
#37368=CARTESIAN_POINT('',(17.7969135048412,23.7543320991532,27.0228886843871));
#37369=CARTESIAN_POINT('Origin',(16.1460502915689,23.7543320991532,35.0294657090004));
#37370=CARTESIAN_POINT('',(17.8984026464748,23.4543320991532,27.3519084005685));
#37371=CARTESIAN_POINT('Ctrl Pts',(17.8984026464748,23.4543320991532,27.3519084005685));
#37372=CARTESIAN_POINT('Ctrl Pts',(17.8486065723088,23.6006388275175,27.1904734930963));
#37373=CARTESIAN_POINT('Ctrl Pts',(17.7969135048412,23.7543320991532,27.0228886843871));
#37374=CARTESIAN_POINT('',(18.132597508217,23.7543320991532,27.0995063676148));
#37375=CARTESIAN_POINT('Ctrl Pts',(18.132597508217,23.7543320991532,27.0995063676148));
#37376=CARTESIAN_POINT('Ctrl Pts',(18.0133113403203,23.6006388275175,27.2280662815959));
#37377=CARTESIAN_POINT('Ctrl Pts',(17.8984026464748,23.4543320991532,27.3519084005685));
#37378=CARTESIAN_POINT('',(18.4440307506263,23.7543320991532,27.1840905866885));
#37379=CARTESIAN_POINT('Origin',(16.1460502915689,23.7543320991532,35.0294657090004));
#37380=CARTESIAN_POINT('',(18.5183640341746,23.4543320991532,27.5202878241288));
#37381=CARTESIAN_POINT('Ctrl Pts',(18.5183640341746,23.4543320991532,27.5202878241288));
#37382=CARTESIAN_POINT('Ctrl Pts',(18.481892095985,23.6006388275175,27.3553312356651));
#37383=CARTESIAN_POINT('Ctrl Pts',(18.4440307506263,23.7543320991532,27.1840905866885));
#37384=CARTESIAN_POINT('',(18.7723527407059,23.7543320991532,27.2878146935091));
#37385=CARTESIAN_POINT('Ctrl Pts',(18.7723527407059,23.7543320991532,27.2878146935091));
#37386=CARTESIAN_POINT('Ctrl Pts',(18.642984661211,23.6006388275175,27.4062239048995));
#37387=CARTESIAN_POINT('Ctrl Pts',(18.5183640341746,23.4543320991532,27.5202878241288));
#37388=CARTESIAN_POINT('',(19.0758553155964,23.7543320991532,27.397502166033));
#37389=CARTESIAN_POINT('Origin',(16.1460502915689,23.7543320991532,35.0294657090004));
#37390=CARTESIAN_POINT('',(19.1225380653215,23.4543320991532,27.7386395875858));
#37391=CARTESIAN_POINT('Ctrl Pts',(19.1225380653215,23.4543320991532,27.7386395875858));
#37392=CARTESIAN_POINT('Ctrl Pts',(19.0996329778396,23.6006388275175,27.5712590770108));
#37393=CARTESIAN_POINT('Ctrl Pts',(19.0758553155964,23.7543320991532,27.397502166033));
#37394=CARTESIAN_POINT('',(19.3946303637052,23.7543320991532,27.5276424296289));
#37395=CARTESIAN_POINT('Ctrl Pts',(19.3946303637052,23.7543320991532,27.5276424296289));
#37396=CARTESIAN_POINT('Ctrl Pts',(19.2560412958369,23.6006388275175,27.635112944663));
#37397=CARTESIAN_POINT('Ctrl Pts',(19.1225380653215,23.4543320991532,27.7386395875858));
#37398=CARTESIAN_POINT('',(19.6881825115154,23.7543320991532,27.6617032035706));
#37399=CARTESIAN_POINT('Origin',(16.1460502915689,23.7543320991532,35.0294657090004));
#37400=CARTESIAN_POINT('',(19.70690406142,23.4543320991532,28.0055105959791));
#37401=CARTESIAN_POINT('Ctrl Pts',(19.70690406142,23.4543320991532,28.0055105959791));
#37402=CARTESIAN_POINT('Ctrl Pts',(19.6977182542238,23.6006388275175,27.8368200529749));
#37403=CARTESIAN_POINT('Ctrl Pts',(19.6881825115154,23.7543320991532,27.6617032035706));
#37404=CARTESIAN_POINT('',(19.9952892223024,23.7543320991532,27.8173935619593));
#37405=CARTESIAN_POINT('Ctrl Pts',(19.9952892223024,23.7543320991532,27.8173935619593));
#37406=CARTESIAN_POINT('Ctrl Pts',(19.8484014534417,23.6006388275175,27.9132101820909));
#37407=CARTESIAN_POINT('Ctrl Pts',(19.70690406142,23.4543320991532,28.0055105959791));
#37408=CARTESIAN_POINT('',(20.2769374019214,23.7543320991532,27.9749354849866));
#37409=CARTESIAN_POINT('Origin',(16.1460502915689,23.7543320991532,35.0294657090004));
#37410=CARTESIAN_POINT('',(20.2675731631797,23.4543320991532,28.3191248667786));
#37411=CARTESIAN_POINT('Ctrl Pts',(20.2675731631797,23.4543320991532,28.3191248667786));
#37412=CARTESIAN_POINT('Ctrl Pts',(20.2721677663006,23.6006388275175,28.1502468990769));
#37413=CARTESIAN_POINT('Ctrl Pts',(20.2769374019214,23.7543320991532,27.9749354849866));
#37414=CARTESIAN_POINT('',(20.5703320308953,23.7543320991532,28.15513984452));
#37415=CARTESIAN_POINT('Ctrl Pts',(20.5703320308953,23.7543320991532,28.15513984452));
#37416=CARTESIAN_POINT('Ctrl Pts',(20.4161230749093,23.6006388275175,28.2386649259508));
#37417=CARTESIAN_POINT('Ctrl Pts',(20.2675731631797,23.4543320991532,28.3191248667786));
#37418=CARTESIAN_POINT('',(20.8382019201564,23.7543320991532,28.3351145011278));
#37419=CARTESIAN_POINT('Origin',(16.1460502915689,23.7543320991532,35.0294657090004));
#37420=CARTESIAN_POINT('',(20.8008142102322,23.4543320991532,28.6773953487548));
#37421=CARTESIAN_POINT('Ctrl Pts',(20.8008142102322,23.4543320991532,28.6773953487548));
#37422=CARTESIAN_POINT('Ctrl Pts',(20.8191586473445,23.6006388275175,28.5094538113677));
#37423=CARTESIAN_POINT('Ctrl Pts',(20.8382019201564,23.7543320991532,28.3351145011278));
#37424=CARTESIAN_POINT('',(21.1159319744681,23.7543320991532,28.538633631525));
#37425=CARTESIAN_POINT('Ctrl Pts',(21.1159319744681,23.7543320991532,28.538633631525));
#37426=CARTESIAN_POINT('Ctrl Pts',(20.9554280665162,23.6006388275175,28.6093113286187));
#37427=CARTESIAN_POINT('Ctrl Pts',(20.8008142102322,23.4543320991532,28.6773953487548));
#37428=CARTESIAN_POINT('',(21.3682409434536,23.7543320991532,28.7398433200673));
#37429=CARTESIAN_POINT('Origin',(16.1460502915689,23.7543320991532,35.0294657090004));
#37430=CARTESIAN_POINT('',(21.303078571388,23.4543320991532,29.0779378109605));
#37431=CARTESIAN_POINT('Ctrl Pts',(21.303078571388,23.4543320991532,29.0779378109605));
#37432=CARTESIAN_POINT('Ctrl Pts',(21.3350507632894,23.6006388275175,28.912050327111));
#37433=CARTESIAN_POINT('Ctrl Pts',(21.3682409434536,23.7543320991532,28.7398433200673));
#37434=CARTESIAN_POINT('',(21.6284581754139,23.7543320991532,28.9653228350936));
#37435=CARTESIAN_POINT('Ctrl Pts',(21.6284581754139,23.7543320991532,28.9653228350936));
#37436=CARTESIAN_POINT('Ctrl Pts',(21.4627274425222,23.6006388275175,29.022682799437));
#37437=CARTESIAN_POINT('Ctrl Pts',(21.303078571388,23.4543320991532,29.0779378109605));
#37438=CARTESIAN_POINT('',(21.8635271495634,23.7543320991532,29.1864285382904));
#37439=CARTESIAN_POINT('Origin',(16.1460502915689,23.7543320991532,35.0294657090004));
#37440=CARTESIAN_POINT('',(21.7710237601914,23.4543320991532,29.5180867093948));
#37441=CARTESIAN_POINT('Ctrl Pts',(21.7710237601914,23.4543320991532,29.5180867093948));
#37442=CARTESIAN_POINT('Ctrl Pts',(21.8164109372197,23.6006388275175,29.3553572329183));
#37443=CARTESIAN_POINT('Ctrl Pts',(21.8635271495634,23.7543320991532,29.1864285382904));
#37444=CARTESIAN_POINT('',(22.1044998564264,23.7543320991532,29.4323679089749));
#37445=CARTESIAN_POINT('Ctrl Pts',(22.1044998564264,23.7543320991532,29.4323679089749));
#37446=CARTESIAN_POINT('Ctrl Pts',(21.9346452092787,23.6006388275175,29.4760284194692));
#37447=CARTESIAN_POINT('Ctrl Pts',(21.7710237601914,23.4543320991532,29.5180867093948));
#37448=CARTESIAN_POINT('',(22.3207644905005,23.7543320991532,29.6718982048514));
#37449=CARTESIAN_POINT('Origin',(16.1460502915689,23.7543320991532,35.0294657090004));
#37450=CARTESIAN_POINT('',(22.2015356786164,23.4543320991532,29.9949129257578));
#37451=CARTESIAN_POINT('Ctrl Pts',(22.2015356786164,23.4543320991532,29.9949129257578));
#37452=CARTESIAN_POINT('Ctrl Pts',(22.2600357965969,23.6006388275175,29.836424394472));
#37453=CARTESIAN_POINT('Ctrl Pts',(22.3207644905005,23.7543320991532,29.6718982048514));
#37454=CARTESIAN_POINT('',(22.5408890386598,23.7543320991532,29.9366607452593));
#37455=CARTESIAN_POINT('Ctrl Pts',(22.5408890386598,23.7543320991532,29.9366607452593));
#37456=CARTESIAN_POINT('Ctrl Pts',(22.3680408319087,23.6006388275175,29.9663312484104));
#37457=CARTESIAN_POINT('Ctrl Pts',(22.2015356786164,23.4543320991532,29.9949129257578));
#37458=CARTESIAN_POINT('',(22.7369101271998,23.7543320991532,30.193021599216));
#37459=CARTESIAN_POINT('Origin',(16.1460502915689,23.7543320991532,35.0294657090004));
#37460=CARTESIAN_POINT('',(22.5917493408753,23.4543320991532,30.5052432602507));
#37461=CARTESIAN_POINT('Ctrl Pts',(22.5917493408753,23.4543320991532,30.5052432602507));
#37462=CARTESIAN_POINT('Ctrl Pts',(22.6629730911747,23.6006388275175,30.3520503891823));
#37463=CARTESIAN_POINT('Ctrl Pts',(22.7369101271998,23.7543320991532,30.193021599216));
#37464=CARTESIAN_POINT('',(22.9347216241054,23.7543320991532,30.4748453583237));
#37465=CARTESIAN_POINT('Ctrl Pts',(22.9347216241053,23.7543320991532,30.4748453583237));
#37466=CARTESIAN_POINT('Ctrl Pts',(22.7600301340489,23.6006388275175,30.4903284018285));
#37467=CARTESIAN_POINT('Ctrl Pts',(22.5917493408753,23.4543320991532,30.5052432602507));
#37468=CARTESIAN_POINT('',(23.1091946791084,23.7543320991532,30.7463307311742));
#37469=CARTESIAN_POINT('Origin',(16.1460502915689,23.7543320991532,35.0294657090004));
#37470=CARTESIAN_POINT('',(22.9390679394266,23.4543320991532,31.0456815486958));
#37471=CARTESIAN_POINT('Ctrl Pts',(22.9390679394266,23.4543320991532,31.0456815486957));
#37472=CARTESIAN_POINT('Ctrl Pts',(23.0225413397378,23.6006388275175,30.8988038111267));
#37473=CARTESIAN_POINT('Ctrl Pts',(23.1091946791084,23.7543320991532,30.7463307311742));
#37474=CARTESIAN_POINT('',(23.2833767218848,23.7543320991532,31.0433402183623));
#37475=CARTESIAN_POINT('Ctrl Pts',(23.2833767218848,23.7543320991532,31.0433402183623));
#37476=CARTESIAN_POINT('Ctrl Pts',(23.1080044915673,23.6006388275175,31.0445327651209));
#37477=CARTESIAN_POINT('Ctrl Pts',(22.9390679394266,23.4543320991532,31.0456815486958));
#37478=CARTESIAN_POINT('',(23.4351406539558,23.7543320991532,31.3281434197422));
#37479=CARTESIAN_POINT('Origin',(16.1460502915689,23.7543320991532,35.0294657090004));
#37480=CARTESIAN_POINT('',(23.2411801263005,23.4543320991532,31.6126312634495));
#37481=CARTESIAN_POINT('Ctrl Pts',(23.2411801263005,23.4543320991532,31.6126312634495));
#37482=CARTESIAN_POINT('Ctrl Pts',(23.3363476749164,23.6006388275175,31.4730461064903));
#37483=CARTESIAN_POINT('Ctrl Pts',(23.4351406539558,23.7543320991532,31.3281434197422));
#37484=CARTESIAN_POINT('',(23.5845340898465,23.7543320991532,31.6383620858768));
#37485=CARTESIAN_POINT('Ctrl Pts',(23.5845340898465,23.7543320991532,31.6383620858768));
#37486=CARTESIAN_POINT('Ctrl Pts',(23.4096481925263,23.6006388275175,31.6252561996872));
#37487=CARTESIAN_POINT('Ctrl Pts',(23.2411801263005,23.4543320991532,31.6126312634495));
#37488=CARTESIAN_POINT('',(23.7125789350568,23.7543320991532,31.9345877974701));
#37489=CARTESIAN_POINT('Origin',(16.1460502915689,23.7543320991532,35.0294657090004));
#37490=CARTESIAN_POINT('',(23.4960753947382,23.4543320991532,32.2023194477005));
#37491=CARTESIAN_POINT('Ctrl Pts',(23.4960753947382,23.4543320991532,32.2023194477005));
#37492=CARTESIAN_POINT('Ctrl Pts',(23.6023037673244,23.6006388275175,32.0709557875407));
#37493=CARTESIAN_POINT('Ctrl Pts',(23.7125789350568,23.7543320991532,31.9345877974701));
#37494=CARTESIAN_POINT('',(23.8361895753941,23.7543320991532,32.2559511885104));
#37495=CARTESIAN_POINT('Ctrl Pts',(23.8361895753941,23.7543320991532,32.2559511885104));
#37496=CARTESIAN_POINT('Ctrl Pts',(23.6629538478638,23.6006388275175,32.2286340868829));
#37497=CARTESIAN_POINT('Ctrl Pts',(23.4960753947382,23.4543320991532,32.2023194477005));
#37498=CARTESIAN_POINT('',(23.9396632164247,23.7543320991532,32.5616280770803));
#37499=CARTESIAN_POINT('Origin',(16.1460502915689,23.7543320991532,35.0294657090004));
#37500=CARTESIAN_POINT('',(23.7020574587831,23.4543320991532,32.8108218238741));
#37501=CARTESIAN_POINT('Ctrl Pts',(23.7020574587831,23.4543320991532,32.8108218238741));
#37502=CARTESIAN_POINT('Ctrl Pts',(23.8186397230465,23.6006388275175,32.6885538639986));
#37503=CARTESIAN_POINT('Ctrl Pts',(23.9396632164247,23.7543320991532,32.5616280770803));
#37504=CARTESIAN_POINT('',(24.0366684527916,23.7543320991532,32.8919975726802));
#37505=CARTESIAN_POINT('Ctrl Pts',(24.0366684527916,23.7543320991532,32.8919975726803));
#37506=CARTESIAN_POINT('Ctrl Pts',(23.8662357502358,23.6006388275175,32.8506510464192));
#37507=CARTESIAN_POINT('Ctrl Pts',(23.7020574587831,23.4543320991532,32.8108218238741));
#37508=CARTESIAN_POINT('',(24.1148822896334,23.7543320991532,33.2050914089663));
#37509=CARTESIAN_POINT('Origin',(16.1460502915689,23.7543320991532,35.0294657090004));
#37510=CARTESIAN_POINT('',(23.8577555417836,23.4543320991532,33.4340889090527));
#37511=CARTESIAN_POINT('Ctrl Pts',(23.8577555417836,23.4543320991532,33.4340889090527));
#37512=CARTESIAN_POINT('Ctrl Pts',(23.9839158619903,23.6006388275175,33.3217303225617));
#37513=CARTESIAN_POINT('Ctrl Pts',(24.1148822896334,23.7543320991532,33.2050914089663));
#37514=CARTESIAN_POINT('',(24.1846365681864,23.7543320991532,33.5422684546398));
#37515=CARTESIAN_POINT('Ctrl Pts',(24.1846365681864,23.7543320991532,33.5422684546398));
#37516=CARTESIAN_POINT('Ctrl Pts',(24.0181410921214,23.6006388275175,33.4871676580557));
#37517=CARTESIAN_POINT('Ctrl Pts',(23.8577555417836,23.4543320991532,33.4340889090527));
#37518=CARTESIAN_POINT('',(24.2370701006596,23.7543320991532,33.8606956508185));
#37519=CARTESIAN_POINT('Origin',(16.1460502915689,23.7543320991532,35.0294657090004));
#37520=CARTESIAN_POINT('',(23.9621334986858,23.4543320991532,34.0679729636163));
#37521=CARTESIAN_POINT('Ctrl Pts',(23.9621334986858,23.4543320991532,34.0679729636163));
#37522=CARTESIAN_POINT('Ctrl Pts',(24.0970322987197,23.6006388275175,33.9662714783651));
#37523=CARTESIAN_POINT('Ctrl Pts',(24.2370701006596,23.7543320991532,33.8606956508185));
#37524=CARTESIAN_POINT('',(24.2791092181837,23.7543320991532,34.2024363889569));
#37525=CARTESIAN_POINT('Ctrl Pts',(24.2791092181837,23.7543320991532,34.2024363889569));
#37526=CARTESIAN_POINT('Ctrl Pts',(24.1176589685329,23.6006388275175,34.1339480087601));
#37527=CARTESIAN_POINT('Ctrl Pts',(23.9621334986858,23.4543320991532,34.0679729636163));
#37528=CARTESIAN_POINT('',(24.3054135097807,23.7543320991532,34.5240778645745));
#37529=CARTESIAN_POINT('Origin',(16.1460502915689,23.7543320991532,35.0294657090004));
#37530=CARTESIAN_POINT('',(24.0144967114075,23.4543320991532,34.7082555937653));
#37531=CARTESIAN_POINT('Ctrl Pts',(24.0144967114075,23.4543320991532,34.7082555937653));
#37532=CARTESIAN_POINT('Ctrl Pts',(24.1572362620112,23.6006388275175,34.6178880163586));
#37533=CARTESIAN_POINT('Ctrl Pts',(24.3054135097807,23.7543320991532,34.5240778645745));
#37534=CARTESIAN_POINT('',(24.3194577028847,23.7543320991532,34.8681080669487));
#37535=CARTESIAN_POINT('Ctrl Pts',(24.3194577028847,23.7543320991532,34.8681080669487));
#37536=CARTESIAN_POINT('Ctrl Pts',(24.164127104422,23.6006388275175,34.7866878820095));
#37537=CARTESIAN_POINT('Ctrl Pts',(24.0144967114075,23.4543320991532,34.7082555937653));
#37538=CARTESIAN_POINT('',(24.3194577028847,23.7543320991532,35.1908233510519));
#37539=CARTESIAN_POINT('Origin',(16.1460502915689,23.7543320991532,35.0294657090004));
#37540=CARTESIAN_POINT('',(24.0144967114075,23.4543320991532,35.3506758242353));
#37541=CARTESIAN_POINT('Ctrl Pts',(24.0144967114075,23.4543320991532,35.3506758242353));
#37542=CARTESIAN_POINT('Ctrl Pts',(24.164127104422,23.6006388275175,35.2722435359911));
#37543=CARTESIAN_POINT('Ctrl Pts',(24.3194577028847,23.7543320991532,35.1908233510519));
#37544=CARTESIAN_POINT('',(24.3054135097807,23.7543320991532,35.5348535534261));
#37545=CARTESIAN_POINT('Ctrl Pts',(24.3054135097807,23.7543320991532,35.5348535534261));
#37546=CARTESIAN_POINT('Ctrl Pts',(24.1572362620112,23.6006388275175,35.441043401642));
#37547=CARTESIAN_POINT('Ctrl Pts',(24.0144967114075,23.4543320991532,35.3506758242353));
#37548=CARTESIAN_POINT('',(24.2791092181837,23.7543320991532,35.8564950290437));
#37549=CARTESIAN_POINT('Origin',(16.1460502915689,23.7543320991532,35.0294657090004));
#37550=CARTESIAN_POINT('',(23.9621334986858,23.4543320991532,35.9909584543843));
#37551=CARTESIAN_POINT('Ctrl Pts',(23.9621334986858,23.4543320991532,35.9909584543843));
#37552=CARTESIAN_POINT('Ctrl Pts',(24.1176589685329,23.6006388275175,35.9249834092406));
#37553=CARTESIAN_POINT('Ctrl Pts',(24.2791092181837,23.7543320991532,35.8564950290437));
#37554=CARTESIAN_POINT('',(24.2370701006596,23.7543320991532,36.1982357671821));
#37555=CARTESIAN_POINT('Ctrl Pts',(24.2370701006596,23.7543320991532,36.1982357671821));
#37556=CARTESIAN_POINT('Ctrl Pts',(24.0970322987197,23.6006388275175,36.0926599396356));
#37557=CARTESIAN_POINT('Ctrl Pts',(23.9621334986858,23.4543320991532,35.9909584543843));
#37558=CARTESIAN_POINT('',(24.1846365681864,23.7543320991532,36.5166629633608));
#37559=CARTESIAN_POINT('Origin',(16.1460502915689,23.7543320991532,35.0294657090004));
#37560=CARTESIAN_POINT('',(23.8577555417836,23.4543320991532,36.6248425089479));
#37561=CARTESIAN_POINT('Ctrl Pts',(23.8577555417836,23.4543320991532,36.6248425089479));
#37562=CARTESIAN_POINT('Ctrl Pts',(24.0181410921214,23.6006388275175,36.5717637599449));
#37563=CARTESIAN_POINT('Ctrl Pts',(24.1846365681864,23.7543320991532,36.5166629633608));
#37564=CARTESIAN_POINT('',(24.1148822896334,23.7543320991532,36.8538400090343));
#37565=CARTESIAN_POINT('Ctrl Pts',(24.1148822896334,23.7543320991532,36.8538400090343));
#37566=CARTESIAN_POINT('Ctrl Pts',(23.9839158619903,23.6006388275175,36.7372010954389));
#37567=CARTESIAN_POINT('Ctrl Pts',(23.8577555417836,23.4543320991532,36.624842508948));
#37568=CARTESIAN_POINT('',(24.0366684527916,23.7543320991532,37.1669338453204));
#37569=CARTESIAN_POINT('Origin',(16.1460502915689,23.7543320991532,35.0294657090004));
#37570=CARTESIAN_POINT('',(23.7020574587831,23.4543320991532,37.2481095941266));
#37571=CARTESIAN_POINT('Ctrl Pts',(23.7020574587831,23.4543320991532,37.2481095941266));
#37572=CARTESIAN_POINT('Ctrl Pts',(23.8662357502359,23.6006388275175,37.2082803715815));
#37573=CARTESIAN_POINT('Ctrl Pts',(24.0366684527916,23.7543320991532,37.1669338453204));
#37574=CARTESIAN_POINT('',(23.9396632164247,23.7543320991532,37.4973033409204));
#37575=CARTESIAN_POINT('Ctrl Pts',(23.9396632164247,23.7543320991532,37.4973033409204));
#37576=CARTESIAN_POINT('Ctrl Pts',(23.8186397230465,23.6006388275175,37.370377554002));
#37577=CARTESIAN_POINT('Ctrl Pts',(23.7020574587831,23.4543320991532,37.2481095941266));
#37578=CARTESIAN_POINT('',(23.8361895753942,23.7543320991532,37.8029802294902));
#37579=CARTESIAN_POINT('Origin',(16.1460502915689,23.7543320991532,35.0294657090004));
#37580=CARTESIAN_POINT('',(23.4960753947382,23.4543320991532,37.8566119703002));
#37581=CARTESIAN_POINT('Ctrl Pts',(23.4960753947382,23.4543320991532,37.8566119703002));
#37582=CARTESIAN_POINT('Ctrl Pts',(23.6629538478638,23.6006388275175,37.8302973311177));
#37583=CARTESIAN_POINT('Ctrl Pts',(23.8361895753942,23.7543320991532,37.8029802294902));
#37584=CARTESIAN_POINT('',(23.7125789350568,23.7543320991532,38.1243436205306));
#37585=CARTESIAN_POINT('Ctrl Pts',(23.7125789350568,23.7543320991532,38.1243436205306));
#37586=CARTESIAN_POINT('Ctrl Pts',(23.6023037673244,23.6006388275175,37.9879756304599));
#37587=CARTESIAN_POINT('Ctrl Pts',(23.4960753947382,23.4543320991532,37.8566119703002));
#37588=CARTESIAN_POINT('',(23.5845340898466,23.7543320991532,38.4205693321238));
#37589=CARTESIAN_POINT('Origin',(16.1460502915689,23.7543320991532,35.0294657090004));
#37590=CARTESIAN_POINT('',(23.2411801263005,23.4543320991532,38.4463001545511));
#37591=CARTESIAN_POINT('Ctrl Pts',(23.2411801263005,23.4543320991532,38.4463001545511));
#37592=CARTESIAN_POINT('Ctrl Pts',(23.4096481925264,23.6006388275175,38.4336752183134));
#37593=CARTESIAN_POINT('Ctrl Pts',(23.5845340898466,23.7543320991532,38.4205693321238));
#37594=CARTESIAN_POINT('',(23.4351406539558,23.7543320991532,38.7307879982584));
#37595=CARTESIAN_POINT('Ctrl Pts',(23.4351406539558,23.7543320991532,38.7307879982584));
#37596=CARTESIAN_POINT('Ctrl Pts',(23.3363476749164,23.6006388275175,38.5858853115103));
#37597=CARTESIAN_POINT('Ctrl Pts',(23.2411801263005,23.4543320991532,38.4463001545511));
#37598=CARTESIAN_POINT('',(23.2833767218849,23.7543320991532,39.0155911996383));
#37599=CARTESIAN_POINT('Origin',(16.1460502915689,23.7543320991532,35.0294657090004));
#37600=CARTESIAN_POINT('',(22.9390679394267,23.4543320991532,39.0132498693049));
#37601=CARTESIAN_POINT('Ctrl Pts',(22.9390679394267,23.4543320991532,39.0132498693049));
#37602=CARTESIAN_POINT('Ctrl Pts',(23.1080044915674,23.6006388275175,39.0143986528797));
#37603=CARTESIAN_POINT('Ctrl Pts',(23.2833767218849,23.7543320991532,39.0155911996383));
#37604=CARTESIAN_POINT('',(23.1091946791084,23.7543320991532,39.3126006868265));
#37605=CARTESIAN_POINT('Ctrl Pts',(23.1091946791084,23.7543320991532,39.3126006868265));
#37606=CARTESIAN_POINT('Ctrl Pts',(23.0225413397378,23.6006388275175,39.1601276068739));
#37607=CARTESIAN_POINT('Ctrl Pts',(22.9390679394267,23.4543320991532,39.0132498693049));
#37608=CARTESIAN_POINT('',(22.9347216241054,23.7543320991532,39.584086059677));
#37609=CARTESIAN_POINT('Origin',(16.1460502915689,23.7543320991532,35.0294657090004));
#37610=CARTESIAN_POINT('',(22.5917493408754,23.4543320991532,39.55368815775));
#37611=CARTESIAN_POINT('Ctrl Pts',(22.5917493408754,23.4543320991532,39.55368815775));
#37612=CARTESIAN_POINT('Ctrl Pts',(22.760030134049,23.6006388275175,39.5686030161721));
#37613=CARTESIAN_POINT('Ctrl Pts',(22.9347216241054,23.7543320991532,39.584086059677));
#37614=CARTESIAN_POINT('',(22.7369101271999,23.7543320991532,39.8659098187846));
#37615=CARTESIAN_POINT('Ctrl Pts',(22.7369101271999,23.7543320991532,39.8659098187846));
#37616=CARTESIAN_POINT('Ctrl Pts',(22.6629730911748,23.6006388275175,39.7068810288184));
#37617=CARTESIAN_POINT('Ctrl Pts',(22.5917493408754,23.4543320991532,39.55368815775));
#37618=CARTESIAN_POINT('',(22.5408890386598,23.7543320991532,40.1222706727414));
#37619=CARTESIAN_POINT('Origin',(16.1460502915689,23.7543320991532,35.0294657090004));
#37620=CARTESIAN_POINT('',(22.2015356786164,23.4543320991532,40.0640184922428));
#37621=CARTESIAN_POINT('Ctrl Pts',(22.2015356786164,23.4543320991532,40.0640184922428));
#37622=CARTESIAN_POINT('Ctrl Pts',(22.3680408319088,23.6006388275175,40.0926001695902));
#37623=CARTESIAN_POINT('Ctrl Pts',(22.5408890386598,23.7543320991532,40.1222706727414));
#37624=CARTESIAN_POINT('',(22.3207644905006,23.7543320991532,40.3870332131493));
#37625=CARTESIAN_POINT('Ctrl Pts',(22.3207644905006,23.7543320991532,40.3870332131493));
#37626=CARTESIAN_POINT('Ctrl Pts',(22.260035796597,23.6006388275175,40.2225070235287));
#37627=CARTESIAN_POINT('Ctrl Pts',(22.2015356786164,23.4543320991532,40.0640184922428));
#37628=CARTESIAN_POINT('',(22.1044998564265,23.7543320991532,40.6265635090257));
#37629=CARTESIAN_POINT('Origin',(16.1460502915689,23.7543320991532,35.0294657090004));
#37630=CARTESIAN_POINT('',(21.7710237601915,23.4543320991532,40.5408447086059));
#37631=CARTESIAN_POINT('Ctrl Pts',(21.7710237601915,23.4543320991532,40.5408447086059));
#37632=CARTESIAN_POINT('Ctrl Pts',(21.9346452092787,23.6006388275175,40.5829029985315));
#37633=CARTESIAN_POINT('Ctrl Pts',(22.1044998564265,23.7543320991532,40.6265635090257));
#37634=CARTESIAN_POINT('',(21.8635271495635,23.7543320991532,40.8725028797102));
#37635=CARTESIAN_POINT('Ctrl Pts',(21.8635271495635,23.7543320991532,40.8725028797102));
#37636=CARTESIAN_POINT('Ctrl Pts',(21.8164109372198,23.6006388275175,40.7035741850823));
#37637=CARTESIAN_POINT('Ctrl Pts',(21.7710237601915,23.4543320991532,40.5408447086059));
#37638=CARTESIAN_POINT('',(21.628458175414,23.7543320991532,41.0936085829071));
#37639=CARTESIAN_POINT('Origin',(16.1460502915689,23.7543320991532,35.0294657090004));
#37640=CARTESIAN_POINT('',(21.3030785713881,23.4543320991532,40.9809936070401));
#37641=CARTESIAN_POINT('Ctrl Pts',(21.3030785713881,23.4543320991532,40.9809936070401));
#37642=CARTESIAN_POINT('Ctrl Pts',(21.4627274425223,23.6006388275175,41.0362486185636));
#37643=CARTESIAN_POINT('Ctrl Pts',(21.628458175414,23.7543320991532,41.0936085829071));
#37644=CARTESIAN_POINT('',(21.3682409434537,23.7543320991532,41.3190880979334));
#37645=CARTESIAN_POINT('Ctrl Pts',(21.3682409434537,23.7543320991532,41.3190880979334));
#37646=CARTESIAN_POINT('Ctrl Pts',(21.3350507632894,23.6006388275175,41.1468810908896));
#37647=CARTESIAN_POINT('Ctrl Pts',(21.3030785713881,23.4543320991532,40.9809936070401));
#37648=CARTESIAN_POINT('',(21.1159319744682,23.7543320991532,41.5202977864757));
#37649=CARTESIAN_POINT('Origin',(16.1460502915689,23.7543320991532,35.0294657090004));
#37650=CARTESIAN_POINT('',(20.8008142102323,23.4543320991532,41.3815360692459));
#37651=CARTESIAN_POINT('Ctrl Pts',(20.8008142102323,23.4543320991532,41.3815360692459));
#37652=CARTESIAN_POINT('Ctrl Pts',(20.9554280665163,23.6006388275175,41.449620089382));
#37653=CARTESIAN_POINT('Ctrl Pts',(21.1159319744682,23.7543320991532,41.5202977864757));
#37654=CARTESIAN_POINT('',(20.8382019201565,23.7543320991532,41.7238169168728));
#37655=CARTESIAN_POINT('Ctrl Pts',(20.8382019201565,23.7543320991532,41.7238169168728));
#37656=CARTESIAN_POINT('Ctrl Pts',(20.8191586473446,23.6006388275175,41.5494776066329));
#37657=CARTESIAN_POINT('Ctrl Pts',(20.8008142102323,23.4543320991532,41.3815360692459));
#37658=CARTESIAN_POINT('',(20.5703320308954,23.7543320991532,41.9037915734806));
#37659=CARTESIAN_POINT('Origin',(16.1460502915689,23.7543320991532,35.0294657090004));
#37660=CARTESIAN_POINT('',(20.2675731631798,23.4543320991532,41.7398065512221));
#37661=CARTESIAN_POINT('Ctrl Pts',(20.2675731631798,23.4543320991532,41.7398065512221));
#37662=CARTESIAN_POINT('Ctrl Pts',(20.4161230749094,23.6006388275175,41.8202664920499));
#37663=CARTESIAN_POINT('Ctrl Pts',(20.5703320308954,23.7543320991532,41.9037915734806));
#37664=CARTESIAN_POINT('',(20.2769374019215,23.7543320991532,42.0839959330141));
#37665=CARTESIAN_POINT('Ctrl Pts',(20.2769374019215,23.7543320991532,42.0839959330141));
#37666=CARTESIAN_POINT('Ctrl Pts',(20.2721677663007,23.6006388275175,41.9086845189237));
#37667=CARTESIAN_POINT('Ctrl Pts',(20.2675731631798,23.4543320991532,41.7398065512221));
#37668=CARTESIAN_POINT('',(19.9952892223025,23.7543320991532,42.2415378560414));
#37669=CARTESIAN_POINT('Origin',(16.1460502915689,23.7543320991532,35.0294657090004));
#37670=CARTESIAN_POINT('',(19.7069040614201,23.4543320991532,42.0534208220216));
#37671=CARTESIAN_POINT('Ctrl Pts',(19.7069040614201,23.4543320991532,42.0534208220216));
#37672=CARTESIAN_POINT('Ctrl Pts',(19.8484014534418,23.6006388275175,42.1457212359098));
#37673=CARTESIAN_POINT('Ctrl Pts',(19.9952892223025,23.7543320991532,42.2415378560414));
#37674=CARTESIAN_POINT('',(19.6881825115155,23.7543320991532,42.3972282144301));
#37675=CARTESIAN_POINT('Ctrl Pts',(19.6881825115155,23.7543320991532,42.3972282144301));
#37676=CARTESIAN_POINT('Ctrl Pts',(19.6977182542239,23.6006388275175,42.2221113650258));
#37677=CARTESIAN_POINT('Ctrl Pts',(19.7069040614201,23.4543320991532,42.0534208220216));
#37678=CARTESIAN_POINT('',(19.3946303637053,23.7543320991532,42.5312889883718));
#37679=CARTESIAN_POINT('Origin',(16.1460502915689,23.7543320991532,35.0294657090004));
#37680=CARTESIAN_POINT('',(19.1225380653216,23.4543320991532,42.3202918304149));
#37681=CARTESIAN_POINT('Ctrl Pts',(19.1225380653216,23.4543320991532,42.3202918304149));
#37682=CARTESIAN_POINT('Ctrl Pts',(19.256041295837,23.6006388275175,42.4238184733377));
#37683=CARTESIAN_POINT('Ctrl Pts',(19.3946303637053,23.7543320991532,42.5312889883718));
#37684=CARTESIAN_POINT('',(19.0758553155965,23.7543320991532,42.6614292519677));
#37685=CARTESIAN_POINT('Ctrl Pts',(19.0758553155965,23.7543320991532,42.6614292519677));
#37686=CARTESIAN_POINT('Ctrl Pts',(19.0996329778397,23.6006388275175,42.4876723409899));
#37687=CARTESIAN_POINT('Ctrl Pts',(19.1225380653216,23.4543320991532,42.3202918304149));
#37688=CARTESIAN_POINT('',(18.772352740706,23.7543320991532,42.7711167244916));
#37689=CARTESIAN_POINT('Origin',(16.1460502915689,23.7543320991532,35.0294657090004));
#37690=CARTESIAN_POINT('',(18.5183640341747,23.4543320991532,42.5386435938719));
#37691=CARTESIAN_POINT('Ctrl Pts',(18.5183640341747,23.4543320991532,42.5386435938719));
#37692=CARTESIAN_POINT('Ctrl Pts',(18.6429846612111,23.6006388275175,42.6527075131012));
#37693=CARTESIAN_POINT('Ctrl Pts',(18.772352740706,23.7543320991532,42.7711167244916));
#37694=CARTESIAN_POINT('',(18.4440307506264,23.7543320991532,42.8748408313122));
#37695=CARTESIAN_POINT('Ctrl Pts',(18.4440307506264,23.7543320991532,42.8748408313122));
#37696=CARTESIAN_POINT('Ctrl Pts',(18.4818920959851,23.6006388275175,42.7036001823356));
#37697=CARTESIAN_POINT('Ctrl Pts',(18.5183640341747,23.4543320991532,42.5386435938719));
#37698=CARTESIAN_POINT('',(18.1325975082171,23.7543320991532,42.9594250503859));
#37699=CARTESIAN_POINT('Origin',(16.1460502915689,23.7543320991532,35.0294657090004));
#37700=CARTESIAN_POINT('',(17.8984026464749,23.4543320991532,42.7070230174322));
#37701=CARTESIAN_POINT('Ctrl Pts',(17.8984026464749,23.4543320991532,42.7070230174322));
#37702=CARTESIAN_POINT('Ctrl Pts',(18.0133113403204,23.6006388275175,42.8308651364048));
#37703=CARTESIAN_POINT('Ctrl Pts',(18.1325975082171,23.7543320991532,42.9594250503859));
#37704=CARTESIAN_POINT('',(17.7969135048413,23.7543320991532,43.0360427336136));
#37705=CARTESIAN_POINT('Ctrl Pts',(17.7969135048413,23.7543320991532,43.0360427336136));
#37706=CARTESIAN_POINT('Ctrl Pts',(17.8486065723089,23.6006388275175,42.8684579249044));
#37707=CARTESIAN_POINT('Ctrl Pts',(17.8984026464749,23.4543320991532,42.7070230174322));
#37708=CARTESIAN_POINT('',(17.4796221317587,23.7543320991532,43.0949608052144));
#37709=CARTESIAN_POINT('Origin',(16.1460502915689,23.7543320991532,35.0294657090004));
#37710=CARTESIAN_POINT('',(17.2667796429711,23.4543320991532,42.8243095638127));
#37711=CARTESIAN_POINT('Ctrl Pts',(17.2667796429711,23.4543320991532,42.8243095638127));
#37712=CARTESIAN_POINT('Ctrl Pts',(17.3712117052267,23.6006388275175,42.9571057336593));
#37713=CARTESIAN_POINT('Ctrl Pts',(17.4796221317587,23.7543320991532,43.0949608052144));
#37714=CARTESIAN_POINT('',(17.1388100367452,23.7543320991532,43.1439621868083));
#37715=CARTESIAN_POINT('Ctrl Pts',(17.1388100367452,23.7543320991532,43.1439621868083));
#37716=CARTESIAN_POINT('Ctrl Pts',(17.2039908174864,23.6006388275175,42.981148467619));
#37717=CARTESIAN_POINT('Ctrl Pts',(17.2667796429711,23.4543320991532,42.8243095638127));
#37718=CARTESIAN_POINT('',(16.8177720547276,23.7543320991532,43.1768220208907));
#37719=CARTESIAN_POINT('Origin',(16.1460502915689,23.7543320991532,35.0294657090004));
#37720=CARTESIAN_POINT('',(16.627698370541,23.4543320991532,42.8897227103981));
#37721=CARTESIAN_POINT('Ctrl Pts',(16.627698370541,23.4543320991532,42.8897227103981));
#37722=CARTESIAN_POINT('Ctrl Pts',(16.7209588230625,23.6006388275175,43.0305891945183));
#37723=CARTESIAN_POINT('Ctrl Pts',(16.8177720547276,23.7543320991532,43.1768220208907));
#37724=CARTESIAN_POINT('',(16.4740999163387,23.7543320991532,43.1978810047409));
#37725=CARTESIAN_POINT('Ctrl Pts',(16.4740999163387,23.7543320991532,43.1978810047409));
#37726=CARTESIAN_POINT('Ctrl Pts',(16.5523346430118,23.6006388275175,43.0409218735102));
#37727=CARTESIAN_POINT('Ctrl Pts',(16.627698370541,23.4543320991532,42.8897227103981));
#37728=CARTESIAN_POINT('',(16.151451780189,23.7543320991532,43.2044639245305));
#37729=CARTESIAN_POINT('Origin',(16.1460502915689,23.7543320991532,35.0294657090004));
#37730=CARTESIAN_POINT('',(16.1460502915689,23.7445176916473,43.1946513014945));
#37731=CARTESIAN_POINT('Ctrl Pts',(16.151451780189,23.7543320991532,43.2044639245305));
#37732=CARTESIAN_POINT('Ctrl Pts',(16.1487494137306,23.7494210562869,43.199554666134));
#37733=CARTESIAN_POINT('Ctrl Pts',(16.1460502915689,23.7445176916473,43.1946513014945));
#37734=CARTESIAN_POINT('',(16.1460502915689,23.3543320991532,42.8044657090004));
#37735=CARTESIAN_POINT('',(16.1460502915689,23.7543320991532,43.2044657090004));
#37736=CARTESIAN_POINT('Origin',(16.1460502915689,23.3543320991532,35.0294657090004));
#37737=CARTESIAN_POINT('',(15.9854118096116,23.4543320991532,42.9028271434904));
#37738=CARTESIAN_POINT('Ctrl Pts',(16.1460502915689,23.7445176916473,43.1946513014945));
#37739=CARTESIAN_POINT('Ctrl Pts',(16.0642779822079,23.5959658936188,43.0460995034659));
#37740=CARTESIAN_POINT('Ctrl Pts',(15.9854118096116,23.4543320991532,42.9028271434904));
#37741=CARTESIAN_POINT('',(15.8072066798038,23.7543320991532,43.197440366574));
#37742=CARTESIAN_POINT('Ctrl Pts',(15.8072066798038,23.7543320991532,43.1974403665741));
#37743=CARTESIAN_POINT('Ctrl Pts',(15.8979747132106,23.6006388275175,43.047380360424));
#37744=CARTESIAN_POINT('Ctrl Pts',(15.9854118096116,23.4543320991532,42.9028271434904));
#37745=CARTESIAN_POINT('',(15.4850955596348,23.7543320991532,43.1777025638257));
#37746=CARTESIAN_POINT('Origin',(16.1460502915689,23.7543320991532,35.0294657090004));
#37747=CARTESIAN_POINT('',(15.3441942712763,23.4543320991532,42.8635356552493));
#37748=CARTESIAN_POINT('Ctrl Pts',(15.3441942712763,23.4543320991532,42.8635356552493));
#37749=CARTESIAN_POINT('Ctrl Pts',(15.4133280809849,23.6006388275175,43.017682970205));
#37750=CARTESIAN_POINT('Ctrl Pts',(15.4850955596348,23.7543320991532,43.1777025638257));
#37751=CARTESIAN_POINT('',(15.1425683915999,23.7543320991532,43.142643204682));
#37752=CARTESIAN_POINT('Ctrl Pts',(15.1425683915999,23.7543320991532,43.142643204682));
#37753=CARTESIAN_POINT('Ctrl Pts',(15.2452656854538,23.6006388275175,43.0004809481952));
#37754=CARTESIAN_POINT('Ctrl Pts',(15.3441942712763,23.4543320991532,42.8635356552493));
#37755=CARTESIAN_POINT('',(14.8231378837718,23.7543320991532,43.0967160312165));
#37756=CARTESIAN_POINT('Origin',(16.1460502915689,23.7543320991532,35.0294657090004));
#37757=CARTESIAN_POINT('',(14.708312952459,23.4543320991532,42.7721097240465));
#37758=CARTESIAN_POINT('Ctrl Pts',(14.708312952459,23.4543320991532,42.7721097240465));
#37759=CARTESIAN_POINT('Ctrl Pts',(14.7646522879162,23.6006388275175,42.9313791738262));
#37760=CARTESIAN_POINT('Ctrl Pts',(14.8231378837718,23.7543320991532,43.0967160312165));
#37761=CARTESIAN_POINT('',(14.4846081098775,23.7543320991532,43.0338541851362));
#37762=CARTESIAN_POINT('Ctrl Pts',(14.4846081098775,23.7543320991532,43.0338541851362));
#37763=CARTESIAN_POINT('Ctrl Pts',(14.5985512306316,23.6006388275175,42.9005357446746));
#37764=CARTESIAN_POINT('Ctrl Pts',(14.708312952459,23.4543320991532,42.7721097240465));
#37765=CARTESIAN_POINT('',(14.1699839717175,23.7543320991532,42.9620432787156));
#37766=CARTESIAN_POINT('Origin',(16.1460502915689,23.7543320991532,35.0294657090004));
#37767=CARTESIAN_POINT('',(14.0819995384235,23.4543320991532,42.6291577743698));
#37768=CARTESIAN_POINT('Ctrl Pts',(14.0819995384235,23.4543320991532,42.6291577743698));
#37769=CARTESIAN_POINT('Ctrl Pts',(14.1251694706472,23.6006388275175,42.7924894470628));
#37770=CARTESIAN_POINT('Ctrl Pts',(14.1699839717175,23.7543320991532,42.9620432787156));
#37771=CARTESIAN_POINT('',(13.8377044517555,23.7543320991532,42.8717972809129));
#37772=CARTESIAN_POINT('Ctrl Pts',(13.8377044517555,23.7543320991532,42.8717972809129));
#37773=CARTESIAN_POINT('Ctrl Pts',(13.9621351267406,23.6006388275175,42.7482098687017));
#37774=CARTESIAN_POINT('Ctrl Pts',(14.0819995384235,23.4543320991532,42.6291577743699));
#37775=CARTESIAN_POINT('',(13.5299804549939,23.7543320991532,42.7745805312714));
#37776=CARTESIAN_POINT('Origin',(16.1460502915689,23.7543320991532,35.0294657090004));
#37777=CARTESIAN_POINT('',(13.4694220416058,23.4543320991532,42.4356311278591));
#37778=CARTESIAN_POINT('Ctrl Pts',(13.4694220416058,23.4543320991532,42.4356311278591));
#37779=CARTESIAN_POINT('Ctrl Pts',(13.4991352818196,23.6006388275175,42.6019380781315));
#37780=CARTESIAN_POINT('Ctrl Pts',(13.5299804549938,23.7543320991532,42.7745805312714));
#37781=CARTESIAN_POINT('',(13.2061624543473,23.7543320991532,42.6575509539721));
#37782=CARTESIAN_POINT('Ctrl Pts',(13.2061624543473,23.7543320991532,42.6575509539721));
#37783=CARTESIAN_POINT('Ctrl Pts',(13.3402526179509,23.6006388275175,42.5445170238492));
#37784=CARTESIAN_POINT('Ctrl Pts',(13.4694220416058,23.4543320991532,42.4356311278591));
#37785=CARTESIAN_POINT('',(12.9073864514114,23.7543320991532,42.5355753225389));
#37786=CARTESIAN_POINT('Origin',(16.1460502915689,23.7543320991532,35.0294657090004));
#37787=CARTESIAN_POINT('',(12.8746570641791,23.4543320991532,42.1928176724172));
#37788=CARTESIAN_POINT('Ctrl Pts',(12.8746570641791,23.4543320991532,42.1928176724172));
#37789=CARTESIAN_POINT('Ctrl Pts',(12.8907158756716,23.6006388275175,42.3609931549536));
#37790=CARTESIAN_POINT('Ctrl Pts',(12.9073864514114,23.7543320991532,42.5355753225389));
#37791=CARTESIAN_POINT('',(12.5941849254484,23.7543320991532,42.3925409782716));
#37792=CARTESIAN_POINT('Ctrl Pts',(12.5941849254484,23.7543320991532,42.3925409782716));
#37793=CARTESIAN_POINT('Ctrl Pts',(12.7370422297551,23.6006388275175,42.2908127523925));
#37794=CARTESIAN_POINT('Ctrl Pts',(12.8746570641791,23.4543320991532,42.1928176724172));
#37795=CARTESIAN_POINT('',(12.3063452213433,23.7543320991532,42.2466181927493));
#37796=CARTESIAN_POINT('Origin',(16.1460502915689,23.7543320991532,35.0294657090004));
#37797=CARTESIAN_POINT('',(12.3016626689387,23.4543320991532,41.9023332915286));
#37798=CARTESIAN_POINT('Ctrl Pts',(12.3016626689387,23.4543320991532,41.9023332915286));
#37799=CARTESIAN_POINT('Ctrl Pts',(12.303960182969,23.6006388275175,42.0712581262397));
#37800=CARTESIAN_POINT('Ctrl Pts',(12.3063452213433,23.7543320991532,42.2466181927493));
#37801=CARTESIAN_POINT('',(12.0058444745445,23.7543320991532,42.0785309514759));
#37802=CARTESIAN_POINT('Ctrl Pts',(12.0058444745445,23.7543320991532,42.0785309514759));
#37803=CARTESIAN_POINT('Ctrl Pts',(12.156518227764,23.6006388275175,41.9887854144));
#37804=CARTESIAN_POINT('Ctrl Pts',(12.3016626689387,23.4543320991532,41.9023332915286));
#37805=CARTESIAN_POINT('',(11.7308565950109,23.7543320991532,41.9096321039267));
#37806=CARTESIAN_POINT('Origin',(16.1460502915689,23.7543320991532,35.0294657090004));
#37807=CARTESIAN_POINT('',(11.7542520390477,23.4543320991532,41.5661111108216));
#37808=CARTESIAN_POINT('Ctrl Pts',(11.7542520390477,23.4543320991532,41.5661111108216));
#37809=CARTESIAN_POINT('Ctrl Pts',(11.7427729660389,23.6006388275175,41.7346611308031));
#37810=CARTESIAN_POINT('Ctrl Pts',(11.7308565950109,23.7543320991532,41.9096321039267));
#37811=CARTESIAN_POINT('',(11.445056410267,23.7543320991532,41.7176105585055));
#37812=CARTESIAN_POINT('Ctrl Pts',(11.445056410267,23.7543320991532,41.7176105585055));
#37813=CARTESIAN_POINT('Ctrl Pts',(11.602543903431,23.6006388275175,41.6404449519749));
#37814=CARTESIAN_POINT('Ctrl Pts',(11.7542520390477,23.4543320991532,41.5661111108216));
#37815=CARTESIAN_POINT('',(11.1847503542733,23.7543320991532,41.5268596428934));
#37816=CARTESIAN_POINT('Origin',(16.1460502915689,23.7543320991532,35.0294657090004));
#37817=CARTESIAN_POINT('',(11.2360681019314,23.4543320991532,41.1863886334361));
#37818=CARTESIAN_POINT('Ctrl Pts',(11.2360681019314,23.4543320991532,41.1863886334361));
#37819=CARTESIAN_POINT('Ctrl Pts',(11.2108888332207,23.6006388275175,41.3534421661138));
#37820=CARTESIAN_POINT('Ctrl Pts',(11.1847503542733,23.7543320991532,41.5268596428934));
#37821=CARTESIAN_POINT('',(10.9155526846602,23.7543320991532,41.3121816650278));
#37822=CARTESIAN_POINT('Ctrl Pts',(10.9155526846602,23.7543320991532,41.3121816650278));
#37823=CARTESIAN_POINT('Ctrl Pts',(11.0788058644853,23.6006388275175,41.2481095134227));
#37824=CARTESIAN_POINT('Ctrl Pts',(11.2360681019314,23.4543320991532,41.1863886334361));
#37825=CARTESIAN_POINT('',(10.6716607460615,23.7543320991532,41.1008480972246));
#37826=CARTESIAN_POINT('Origin',(16.1460502915689,23.7543320991532,35.0294657090004));
#37827=CARTESIAN_POINT('',(10.7505592861972,23.4543320991532,40.7656928498092));
#37828=CARTESIAN_POINT('Ctrl Pts',(10.7505592861972,23.4543320991532,40.7656928498092));
#37829=CARTESIAN_POINT('Ctrl Pts',(10.7118473856633,23.6006388275175,40.930138181485));
#37830=CARTESIAN_POINT('Ctrl Pts',(10.6716607460615,23.7543320991532,41.1008480972246));
#37831=CARTESIAN_POINT('',(10.420857057656,23.7543320991532,40.864942333438));
#37832=CARTESIAN_POINT('Ctrl Pts',(10.420857057656,23.7543320991532,40.864942333438));
#37833=CARTESIAN_POINT('Ctrl Pts',(10.5887895011653,23.6006388275175,40.8143900263561));
#37834=CARTESIAN_POINT('Ctrl Pts',(10.7505592861972,23.4543320991532,40.7656928498093));
#37835=CARTESIAN_POINT('',(10.1950022970645,23.7543320991532,40.6344325034697));
#37836=CARTESIAN_POINT('Origin',(16.1460502915689,23.7543320991532,35.0294657090004));
#37837=CARTESIAN_POINT('',(10.3009565729103,23.4543320991532,40.3068234209711));
#37838=CARTESIAN_POINT('Ctrl Pts',(10.3009565729103,23.4543320991532,40.3068234209712));
#37839=CARTESIAN_POINT('Ctrl Pts',(10.2489696618645,23.6006388275175,40.4675661950943));
#37840=CARTESIAN_POINT('Ctrl Pts',(10.1950022970645,23.7543320991532,40.6344325034697));
#37841=CARTESIAN_POINT('',(9.96426164703311,23.7543320991532,40.3788688676983));
#37842=CARTESIAN_POINT('Ctrl Pts',(9.9642616470331,23.7543320991532,40.3788688676983));
#37843=CARTESIAN_POINT('Ctrl Pts',(10.135755791522,23.6006388275175,40.3421728224027));
#37844=CARTESIAN_POINT('Ctrl Pts',(10.3009565729103,23.4543320991532,40.3068234209712));
#37845=CARTESIAN_POINT('',(9.75794709061699,23.7543320991532,40.1307167804521));
#37846=CARTESIAN_POINT('Origin',(16.1460502915689,23.7543320991532,35.0294657090004));
#37847=CARTESIAN_POINT('',(9.89025199394856,23.4543320991532,39.8128340472626));
#37848=CARTESIAN_POINT('Ctrl Pts',(9.89025199394855,23.4543320991532,39.8128340472626));
#37849=CARTESIAN_POINT('Ctrl Pts',(9.82533603670643,23.6006388275175,39.968804547192));
#37850=CARTESIAN_POINT('Ctrl Pts',(9.75794709061698,23.7543320991532,40.1307167804521));
#37851=CARTESIAN_POINT('',(9.54880501991626,23.7543320991532,39.857196006527));
#37852=CARTESIAN_POINT('Ctrl Pts',(9.54880501991626,23.7543320991532,39.857196006527));
#37853=CARTESIAN_POINT('Ctrl Pts',(9.72271960014766,23.6006388275175,39.8346004291447));
#37854=CARTESIAN_POINT('Ctrl Pts',(9.89025199394855,23.4543320991532,39.8128340472626));
#37855=CARTESIAN_POINT('',(9.36340365700901,23.7543320991532,39.5930530732011));
#37856=CARTESIAN_POINT('Origin',(16.1460502915689,23.7543320991532,35.0294657090004));
#37857=CARTESIAN_POINT('',(9.52117872052339,23.4543320991532,39.2870121464632));
#37858=CARTESIAN_POINT('Ctrl Pts',(9.52117872052339,23.4543320991532,39.2870121464632));
#37859=CARTESIAN_POINT('Ctrl Pts',(9.44376572207008,23.6006388275175,39.4371724142552));
#37860=CARTESIAN_POINT('Ctrl Pts',(9.36340365700902,23.7543320991532,39.5930530732011));
#37861=CARTESIAN_POINT('',(9.17725197161341,23.7543320991532,39.303395396745));
#37862=CARTESIAN_POINT('Ctrl Pts',(9.17725197161342,23.7543320991532,39.303395396745));
#37863=CARTESIAN_POINT('Ctrl Pts',(9.3524296147498,23.6006388275175,39.2950506571155));
#37864=CARTESIAN_POINT('Ctrl Pts',(9.52117872052339,23.4543320991532,39.2870121464632));
#37865=CARTESIAN_POINT('',(9.01399761769611,23.7543320991532,39.0250194449803));
#37866=CARTESIAN_POINT('Origin',(16.1460502915689,23.7543320991532,35.0294657090004));
#37867=CARTESIAN_POINT('',(9.19619287437666,23.4543320991532,38.7328569765682));
#37868=CARTESIAN_POINT('Ctrl Pts',(9.19619287437665,23.4543320991532,38.7328569765682));
#37869=CARTESIAN_POINT('Ctrl Pts',(9.10679800544461,23.6006388275175,38.8762077204153));
#37870=CARTESIAN_POINT('Ctrl Pts',(9.01399761769611,23.7543320991532,39.0250194449803));
#37871=CARTESIAN_POINT('',(8.85207512635908,23.7543320991532,38.7211524900399));
#37872=CARTESIAN_POINT('Ctrl Pts',(8.85207512635908,23.7543320991532,38.7211524900399));
#37873=CARTESIAN_POINT('Ctrl Pts',(9.02735005408766,23.6006388275175,38.7271141210286));
#37874=CARTESIAN_POINT('Ctrl Pts',(9.19619287437665,23.4543320991532,38.7328569765682));
#37875=CARTESIAN_POINT('',(8.71205421222197,23.7543320991532,38.4303960658666));
#37876=CARTESIAN_POINT('Origin',(16.1460502915689,23.7543320991532,35.0294657090004));
#37877=CARTESIAN_POINT('',(8.91745718269558,23.4543320991532,38.154056348804));
#37878=CARTESIAN_POINT('Ctrl Pts',(8.91745718269558,23.4543320991532,38.154056348804));
#37879=CARTESIAN_POINT('Ctrl Pts',(8.81667535138843,23.6006388275175,38.2896435931571));
#37880=CARTESIAN_POINT('Ctrl Pts',(8.71205421222197,23.7543320991532,38.4303960658666));
#37881=CARTESIAN_POINT('',(8.57543848240802,23.7543320991532,38.1143420168924));
#37882=CARTESIAN_POINT('Ctrl Pts',(8.57543848240802,23.7543320991532,38.1143420168924));
#37883=CARTESIAN_POINT('Ctrl Pts',(8.74964426900309,23.6006388275175,38.1345703448287));
#37884=CARTESIAN_POINT('Ctrl Pts',(8.91745718269558,23.4543320991532,38.154056348804));
#37885=CARTESIAN_POINT('',(8.45958282413287,23.7543320991532,37.8131400563419));
#37886=CARTESIAN_POINT('Origin',(16.1460502915689,23.7543320991532,35.0294657090004));
#37887=CARTESIAN_POINT('',(8.68682658552014,23.4543320991532,37.5544620858532));
#37888=CARTESIAN_POINT('Ctrl Pts',(8.68682658552015,23.4543320991532,37.5544620858532));
#37889=CARTESIAN_POINT('Ctrl Pts',(8.57532847829742,23.6006388275175,37.6813835199714));
#37890=CARTESIAN_POINT('Ctrl Pts',(8.45958282413287,23.7543320991532,37.8131400563418));
#37891=CARTESIAN_POINT('',(8.3491830109839,23.7543320991532,37.4870022008846));
#37892=CARTESIAN_POINT('Ctrl Pts',(8.3491830109839,23.7543320991532,37.4870022008846));
#37893=CARTESIAN_POINT('Ctrl Pts',(8.5211603456776,23.6006388275175,37.5213626095835));
#37894=CARTESIAN_POINT('Ctrl Pts',(8.68682658552015,23.4543320991532,37.5544620858532));
#37895=CARTESIAN_POINT('',(8.25826360886169,23.7543320991532,37.1773591533095));
#37896=CARTESIAN_POINT('Origin',(16.1460502915689,23.7543320991532,35.0294657090004));
#37897=CARTESIAN_POINT('',(8.50583589142318,23.4543320991532,36.9380643886094));
#37898=CARTESIAN_POINT('Ctrl Pts',(8.50583589142318,23.4543320991532,36.9380643886094));
#37899=CARTESIAN_POINT('Ctrl Pts',(8.38436350979254,23.6006388275175,37.0554753712894));
#37900=CARTESIAN_POINT('Ctrl Pts',(8.25826360886169,23.7543320991532,37.1773591533095));
#37901=CARTESIAN_POINT('',(8.17481440491953,23.7543320991532,36.8433078849883));
#37902=CARTESIAN_POINT('Ctrl Pts',(8.17481440491953,23.7543320991532,36.8433078849883));
#37903=CARTESIAN_POINT('Ctrl Pts',(8.34341880692372,23.6006388275175,36.8915717115991));
#37904=CARTESIAN_POINT('Ctrl Pts',(8.50583589142317,23.4543320991532,36.9380643886094));
#37905=CARTESIAN_POINT('',(8.10943631257072,23.7543320991532,36.5272843737828));
#37906=CARTESIAN_POINT('Origin',(16.1460502915689,23.7543320991532,35.0294657090004));
#37907=CARTESIAN_POINT('',(8.37568956361253,23.4543320991532,36.3089652820495));
#37908=CARTESIAN_POINT('Ctrl Pts',(8.37568956361253,23.4543320991532,36.3089652820495));
#37909=CARTESIAN_POINT('Ctrl Pts',(8.24505128623221,23.6006388275175,36.4160844625728));
#37910=CARTESIAN_POINT('Ctrl Pts',(8.10943631257073,23.7543320991532,36.5272843737828));
#37911=CARTESIAN_POINT('',(8.05349305851946,23.7543320991532,36.1875427486737));
#37912=CARTESIAN_POINT('Ctrl Pts',(8.05349305851946,23.7543320991532,36.1875427486737));
#37913=CARTESIAN_POINT('Ctrl Pts',(8.21760249335658,23.6006388275175,36.2493888053932));
#37914=CARTESIAN_POINT('Ctrl Pts',(8.37568956361253,23.4543320991532,36.3089652820495));
#37915=CARTESIAN_POINT('',(8.01409135636202,23.7543320991532,35.8672418581646));
#37916=CARTESIAN_POINT('Origin',(16.1460502915689,23.7543320991532,35.0294657090004));
#37917=CARTESIAN_POINT('',(8.29725370442716,23.4543320991532,35.6713513169335));
#37918=CARTESIAN_POINT('Ctrl Pts',(8.29725370442717,23.4543320991532,35.6713513169335));
#37919=CARTESIAN_POINT('Ctrl Pts',(8.15831890747932,23.6006388275175,35.7674658348272));
#37920=CARTESIAN_POINT('Ctrl Pts',(8.01409135636202,23.7543320991532,35.8672418581646));
#37921=CARTESIAN_POINT('',(7.98602634532737,23.7543320991532,35.5240708007294));
#37922=CARTESIAN_POINT('Ctrl Pts',(7.98602634532737,23.7543320991532,35.5240708007294));
#37923=CARTESIAN_POINT('Ctrl Pts',(8.14454869178474,23.6006388275175,35.5990875122539));
#37924=CARTESIAN_POINT('Ctrl Pts',(8.29725370442716,23.4543320991532,35.6713513169335));
#37925=CARTESIAN_POINT('',(7.97286324518834,23.7543320991532,35.2016240804971));
#37926=CARTESIAN_POINT('Origin',(16.1460502915689,23.7543320991532,35.0294657090004));
#37927=CARTESIAN_POINT('',(8.27105029156894,23.4543320991532,35.0294657090004));
#37928=CARTESIAN_POINT('Ctrl Pts',(8.27105029156893,23.4543320991532,35.0294657090004));
#37929=CARTESIAN_POINT('Ctrl Pts',(8.12474356320462,23.6006388275175,35.1139359380058));
#37930=CARTESIAN_POINT('Ctrl Pts',(7.97286324518834,23.7543320991532,35.2016240804971));
#37931=CARTESIAN_POINT('',(7.97286324518834,23.7543320991532,34.8573073375037));
#37932=CARTESIAN_POINT('Ctrl Pts',(7.97286324518833,23.7543320991532,34.8573073375037));
#37933=CARTESIAN_POINT('Ctrl Pts',(8.12474356320462,23.6006388275175,34.944995479995));
#37934=CARTESIAN_POINT('Ctrl Pts',(8.27105029156893,23.4543320991532,35.0294657090004));
#37935=CARTESIAN_POINT('',(7.98602634532736,23.7543320991532,34.5348606172715));
#37936=CARTESIAN_POINT('Origin',(16.1460502915689,23.7543320991532,35.0294657090004));
#37937=CARTESIAN_POINT('',(8.29725370442715,23.4543320991532,34.3875801010673));
#37938=CARTESIAN_POINT('Ctrl Pts',(8.29725370442715,23.4543320991532,34.3875801010673));
#37939=CARTESIAN_POINT('Ctrl Pts',(8.14454869178473,23.6006388275175,34.4598439057469));
#37940=CARTESIAN_POINT('Ctrl Pts',(7.98602634532737,23.7543320991532,34.5348606172715));
#37941=CARTESIAN_POINT('',(8.01409135636201,23.7543320991532,34.1916895598362));
#37942=CARTESIAN_POINT('Ctrl Pts',(8.01409135636201,23.7543320991532,34.1916895598362));
#37943=CARTESIAN_POINT('Ctrl Pts',(8.1583189074793,23.6006388275175,34.2914655831736));
#37944=CARTESIAN_POINT('Ctrl Pts',(8.29725370442715,23.4543320991532,34.3875801010673));
#37945=CARTESIAN_POINT('',(8.05349305851944,23.7543320991532,33.8713886693271));
#37946=CARTESIAN_POINT('Origin',(16.1460502915689,23.7543320991532,35.0294657090004));
#37947=CARTESIAN_POINT('',(8.37568956361252,23.4543320991532,33.7499661359513));
#37948=CARTESIAN_POINT('Ctrl Pts',(8.37568956361251,23.4543320991532,33.7499661359513));
#37949=CARTESIAN_POINT('Ctrl Pts',(8.21760249335657,23.6006388275175,33.8095426126077));
#37950=CARTESIAN_POINT('Ctrl Pts',(8.05349305851945,23.7543320991532,33.8713886693271));
#37951=CARTESIAN_POINT('',(8.1094363125707,23.7543320991532,33.5316470442181));
#37952=CARTESIAN_POINT('Ctrl Pts',(8.1094363125707,23.7543320991532,33.5316470442181));
#37953=CARTESIAN_POINT('Ctrl Pts',(8.24505128623219,23.6006388275175,33.642846955428));
#37954=CARTESIAN_POINT('Ctrl Pts',(8.37568956361251,23.4543320991532,33.7499661359513));
#37955=CARTESIAN_POINT('',(8.17481440491951,23.7543320991532,33.2156235330125));
#37956=CARTESIAN_POINT('Origin',(16.1460502915689,23.7543320991532,35.0294657090004));
#37957=CARTESIAN_POINT('',(8.50583589142315,23.4543320991532,33.1208670293914));
#37958=CARTESIAN_POINT('Ctrl Pts',(8.50583589142315,23.4543320991532,33.1208670293914));
#37959=CARTESIAN_POINT('Ctrl Pts',(8.3434188069237,23.6006388275175,33.1673597064018));
#37960=CARTESIAN_POINT('Ctrl Pts',(8.17481440491951,23.7543320991532,33.2156235330125));
#37961=CARTESIAN_POINT('',(8.25826360886166,23.7543320991532,32.8815722646913));
#37962=CARTESIAN_POINT('Ctrl Pts',(8.25826360886166,23.7543320991532,32.8815722646913));
#37963=CARTESIAN_POINT('Ctrl Pts',(8.38436350979251,23.6006388275175,33.0034560467115));
#37964=CARTESIAN_POINT('Ctrl Pts',(8.50583589142315,23.4543320991532,33.1208670293914));
#37965=CARTESIAN_POINT('',(8.34918301098388,23.7543320991532,32.5719292171162));
#37966=CARTESIAN_POINT('Origin',(16.1460502915689,23.7543320991532,35.0294657090004));
#37967=CARTESIAN_POINT('',(8.68682658552011,23.4543320991532,32.5044693321477));
#37968=CARTESIAN_POINT('Ctrl Pts',(8.68682658552011,23.4543320991532,32.5044693321477));
#37969=CARTESIAN_POINT('Ctrl Pts',(8.52116034567756,23.6006388275175,32.5375688084173));
#37970=CARTESIAN_POINT('Ctrl Pts',(8.34918301098388,23.7543320991532,32.5719292171162));
#37971=CARTESIAN_POINT('',(8.45958282413283,23.7543320991532,32.245791361659));
#37972=CARTESIAN_POINT('Ctrl Pts',(8.45958282413283,23.7543320991532,32.245791361659));
#37973=CARTESIAN_POINT('Ctrl Pts',(8.57532847829738,23.6006388275175,32.3775478980294));
#37974=CARTESIAN_POINT('Ctrl Pts',(8.68682658552011,23.4543320991532,32.5044693321477));
#37975=CARTESIAN_POINT('',(8.57543848240798,23.7543320991532,31.9445894011085));
#37976=CARTESIAN_POINT('Origin',(16.1460502915689,23.7543320991532,35.0294657090004));
#37977=CARTESIAN_POINT('',(8.91745718269554,23.4543320991532,31.9048750691968));
#37978=CARTESIAN_POINT('Ctrl Pts',(8.91745718269554,23.4543320991532,31.9048750691968));
#37979=CARTESIAN_POINT('Ctrl Pts',(8.74964426900305,23.6006388275175,31.9243610731722));
#37980=CARTESIAN_POINT('Ctrl Pts',(8.57543848240798,23.7543320991532,31.9445894011085));
#37981=CARTESIAN_POINT('',(8.71205421222193,23.7543320991532,31.6285353521343));
#37982=CARTESIAN_POINT('Ctrl Pts',(8.71205421222193,23.7543320991532,31.6285353521343));
#37983=CARTESIAN_POINT('Ctrl Pts',(8.81667535138839,23.6006388275175,31.7692878248437));
#37984=CARTESIAN_POINT('Ctrl Pts',(8.91745718269554,23.4543320991532,31.9048750691968));
#37985=CARTESIAN_POINT('',(8.85207512635903,23.7543320991532,31.337778927961));
#37986=CARTESIAN_POINT('Origin',(16.1460502915689,23.7543320991532,35.0294657090004));
#37987=CARTESIAN_POINT('',(9.19619287437661,23.4543320991532,31.3260744414326));
#37988=CARTESIAN_POINT('Ctrl Pts',(9.19619287437661,23.4543320991532,31.3260744414326));
#37989=CARTESIAN_POINT('Ctrl Pts',(9.02735005408761,23.6006388275175,31.3318172969722));
#37990=CARTESIAN_POINT('Ctrl Pts',(8.85207512635904,23.7543320991532,31.3377789279609));
#37991=CARTESIAN_POINT('',(9.01399761769606,23.7543320991532,31.0339119730205));
#37992=CARTESIAN_POINT('Ctrl Pts',(9.01399761769606,23.7543320991532,31.0339119730205));
#37993=CARTESIAN_POINT('Ctrl Pts',(9.10679800544456,23.6006388275175,31.1827236975856));
#37994=CARTESIAN_POINT('Ctrl Pts',(9.1961928743766,23.4543320991532,31.3260744414326));
#37995=CARTESIAN_POINT('',(9.17725197161336,23.7543320991532,30.7555360212558));
#37996=CARTESIAN_POINT('Origin',(16.1460502915689,23.7543320991532,35.0294657090004));
#37997=CARTESIAN_POINT('',(9.52117872052333,23.4543320991532,30.7719192715376));
#37998=CARTESIAN_POINT('Ctrl Pts',(9.52117872052333,23.4543320991532,30.7719192715376));
#37999=CARTESIAN_POINT('Ctrl Pts',(9.35242961474975,23.6006388275175,30.7638807608853));
#38000=CARTESIAN_POINT('Ctrl Pts',(9.17725197161336,23.7543320991532,30.7555360212558));
#38001=CARTESIAN_POINT('',(9.36340365700895,23.7543320991532,30.4658783447997));
#38002=CARTESIAN_POINT('Ctrl Pts',(9.36340365700895,23.7543320991532,30.4658783447997));
#38003=CARTESIAN_POINT('Ctrl Pts',(9.44376572207002,23.6006388275175,30.6217590037456));
#38004=CARTESIAN_POINT('Ctrl Pts',(9.52117872052333,23.4543320991532,30.7719192715376));
#38005=CARTESIAN_POINT('',(9.54880501991619,23.7543320991532,30.2017354114738));
#38006=CARTESIAN_POINT('Origin',(16.1460502915689,23.7543320991532,35.0294657090004));
#38007=CARTESIAN_POINT('',(9.89025199394849,23.4543320991532,30.2460973707382));
#38008=CARTESIAN_POINT('Ctrl Pts',(9.89025199394849,23.4543320991532,30.2460973707382));
#38009=CARTESIAN_POINT('Ctrl Pts',(9.7227196001476,23.6006388275175,30.2243309888561));
#38010=CARTESIAN_POINT('Ctrl Pts',(9.5488050199162,23.7543320991532,30.2017354114738));
#38011=CARTESIAN_POINT('',(9.75794709061692,23.7543320991532,29.9282146375487));
#38012=CARTESIAN_POINT('Ctrl Pts',(9.75794709061692,23.7543320991532,29.9282146375487));
#38013=CARTESIAN_POINT('Ctrl Pts',(9.82533603670636,23.6006388275175,30.0901268708088));
#38014=CARTESIAN_POINT('Ctrl Pts',(9.89025199394849,23.4543320991532,30.2460973707382));
#38015=CARTESIAN_POINT('',(9.96426164703304,23.7543320991532,29.6800625503025));
#38016=CARTESIAN_POINT('Origin',(16.1460502915689,23.7543320991532,35.0294657090004));
#38017=CARTESIAN_POINT('',(10.3009565729102,23.4543320991532,29.7521079970296));
#38018=CARTESIAN_POINT('Ctrl Pts',(10.3009565729102,23.4543320991532,29.7521079970297));
#38019=CARTESIAN_POINT('Ctrl Pts',(10.1357557915219,23.6006388275175,29.7167585955981));
#38020=CARTESIAN_POINT('Ctrl Pts',(9.96426164703304,23.7543320991532,29.6800625503025));
#38021=CARTESIAN_POINT('',(10.1950022970644,23.7543320991532,29.4244989145311));
#38022=CARTESIAN_POINT('Ctrl Pts',(10.1950022970644,23.7543320991532,29.4244989145311));
#38023=CARTESIAN_POINT('Ctrl Pts',(10.2489696618644,23.6006388275175,29.5913652229065));
#38024=CARTESIAN_POINT('Ctrl Pts',(10.3009565729102,23.4543320991532,29.7521079970296));
#38025=CARTESIAN_POINT('',(10.4208570576559,23.7543320991532,29.1939890845628));
#38026=CARTESIAN_POINT('Origin',(16.1460502915689,23.7543320991532,35.0294657090004));
#38027=CARTESIAN_POINT('',(10.7505592861971,23.4543320991532,29.2932385681916));
#38028=CARTESIAN_POINT('Ctrl Pts',(10.7505592861971,23.4543320991532,29.2932385681915));
#38029=CARTESIAN_POINT('Ctrl Pts',(10.5887895011652,23.6006388275175,29.2445413916448));
#38030=CARTESIAN_POINT('Ctrl Pts',(10.4208570576559,23.7543320991532,29.1939890845628));
#38031=CARTESIAN_POINT('',(10.6716607460615,23.7543320991532,28.9580833207762));
#38032=CARTESIAN_POINT('Ctrl Pts',(10.6716607460615,23.7543320991532,28.9580833207762));
#38033=CARTESIAN_POINT('Ctrl Pts',(10.7118473856633,23.6006388275175,29.1287932365158));
#38034=CARTESIAN_POINT('Ctrl Pts',(10.7505592861971,23.4543320991532,29.2932385681916));
#38035=CARTESIAN_POINT('',(10.9155526846601,23.7543320991532,28.746749752973));
#38036=CARTESIAN_POINT('Origin',(16.1460502915689,23.7543320991532,35.0294657090004));
#38037=CARTESIAN_POINT('',(11.2360681019313,23.4543320991532,28.8725427845647));
#38038=CARTESIAN_POINT('Ctrl Pts',(11.2360681019313,23.4543320991532,28.8725427845647));
#38039=CARTESIAN_POINT('Ctrl Pts',(11.0788058644852,23.6006388275175,28.8108219045781));
#38040=CARTESIAN_POINT('Ctrl Pts',(10.9155526846601,23.7543320991532,28.746749752973));
#38041=CARTESIAN_POINT('',(11.1847503542732,23.7543320991532,28.5320717751074));
#38042=CARTESIAN_POINT('Ctrl Pts',(11.1847503542732,23.7543320991532,28.5320717751074));
#38043=CARTESIAN_POINT('Ctrl Pts',(11.2108888332206,23.6006388275175,28.705489251887));
#38044=CARTESIAN_POINT('Ctrl Pts',(11.2360681019313,23.4543320991532,28.8725427845647));
#38045=CARTESIAN_POINT('',(11.4450564102669,23.7543320991532,28.3413208594953));
#38046=CARTESIAN_POINT('Origin',(16.1460502915689,23.7543320991532,35.0294657090004));
#38047=CARTESIAN_POINT('',(11.7542520390476,23.4543320991532,28.4928203071792));
#38048=CARTESIAN_POINT('Ctrl Pts',(11.7542520390476,23.4543320991532,28.4928203071792));
#38049=CARTESIAN_POINT('Ctrl Pts',(11.6025439034309,23.6006388275175,28.4184864660259));
#38050=CARTESIAN_POINT('Ctrl Pts',(11.4450564102669,23.7543320991532,28.3413208594953));
#38051=CARTESIAN_POINT('',(11.7308565950108,23.7543320991532,28.1492993140741));
#38052=CARTESIAN_POINT('Ctrl Pts',(11.7308565950108,23.7543320991532,28.1492993140741));
#38053=CARTESIAN_POINT('Ctrl Pts',(11.7427729660389,23.6006388275175,28.3242702871977));
#38054=CARTESIAN_POINT('Ctrl Pts',(11.7542520390476,23.4543320991532,28.4928203071792));
#38055=CARTESIAN_POINT('',(12.0058444745444,23.7543320991532,27.9804004665249));
#38056=CARTESIAN_POINT('Origin',(16.1460502915689,23.7543320991532,35.0294657090004));
#38057=CARTESIAN_POINT('',(12.3016626689386,23.4543320991532,28.1565981264722));
#38058=CARTESIAN_POINT('Ctrl Pts',(12.3016626689386,23.4543320991532,28.1565981264722));
#38059=CARTESIAN_POINT('Ctrl Pts',(12.1565182277639,23.6006388275175,28.0701460036008));
#38060=CARTESIAN_POINT('Ctrl Pts',(12.0058444745444,23.7543320991532,27.9804004665249));
#38061=CARTESIAN_POINT('',(12.3063452213432,23.7543320991532,27.8123132252514));
#38062=CARTESIAN_POINT('Ctrl Pts',(12.3063452213432,23.7543320991532,27.8123132252514));
#38063=CARTESIAN_POINT('Ctrl Pts',(12.3039601829689,23.6006388275175,27.9876732917611));
#38064=CARTESIAN_POINT('Ctrl Pts',(12.3016626689386,23.4543320991532,28.1565981264722));
#38065=CARTESIAN_POINT('',(12.5941849254483,23.7543320991532,27.6663904397292));
#38066=CARTESIAN_POINT('Origin',(16.1460502915689,23.7543320991532,35.0294657090004));
#38067=CARTESIAN_POINT('',(12.874657064179,23.4543320991532,27.8661137455836));
#38068=CARTESIAN_POINT('Ctrl Pts',(12.874657064179,23.4543320991532,27.8661137455836));
#38069=CARTESIAN_POINT('Ctrl Pts',(12.7370422297551,23.6006388275175,27.7681186656083));
#38070=CARTESIAN_POINT('Ctrl Pts',(12.5941849254483,23.7543320991532,27.6663904397292));
#38071=CARTESIAN_POINT('',(12.9073864514113,23.7543320991532,27.5233560954618));
#38072=CARTESIAN_POINT('Ctrl Pts',(12.9073864514113,23.7543320991532,27.5233560954618));
#38073=CARTESIAN_POINT('Ctrl Pts',(12.8907158756715,23.6006388275175,27.6979382630472));
#38074=CARTESIAN_POINT('Ctrl Pts',(12.874657064179,23.4543320991532,27.8661137455836));
#38075=CARTESIAN_POINT('',(13.2061624543472,23.7543320991532,27.4013804640286));
#38076=CARTESIAN_POINT('Origin',(16.1460502915689,23.7543320991532,35.0294657090004));
#38077=CARTESIAN_POINT('',(13.4694220416057,23.4543320991532,27.6233002901416));
#38078=CARTESIAN_POINT('Ctrl Pts',(13.4694220416057,23.4543320991532,27.6233002901416));
#38079=CARTESIAN_POINT('Ctrl Pts',(13.3402526179508,23.6006388275175,27.5144143941516));
#38080=CARTESIAN_POINT('Ctrl Pts',(13.2061624543472,23.7543320991532,27.4013804640286));
#38081=CARTESIAN_POINT('',(13.5299804549937,23.7543320991532,27.2843508867294));
#38082=CARTESIAN_POINT('Ctrl Pts',(13.5299804549937,23.7543320991532,27.2843508867294));
#38083=CARTESIAN_POINT('Ctrl Pts',(13.4991352818195,23.6006388275175,27.4569933398693));
#38084=CARTESIAN_POINT('Ctrl Pts',(13.4694220416057,23.4543320991532,27.6233002901416));
#38085=CARTESIAN_POINT('',(13.8377044517554,23.7543320991532,27.1871341370879));
#38086=CARTESIAN_POINT('Origin',(16.1460502915689,23.7543320991532,35.0294657090004));
#38087=CARTESIAN_POINT('',(14.0819995384234,23.4543320991532,27.4297736436309));
#38088=CARTESIAN_POINT('Ctrl Pts',(14.0819995384234,23.4543320991532,27.4297736436309));
#38089=CARTESIAN_POINT('Ctrl Pts',(13.9621351267405,23.6006388275175,27.310721549299));
#38090=CARTESIAN_POINT('Ctrl Pts',(13.8377044517554,23.7543320991532,27.1871341370879));
#38091=CARTESIAN_POINT('',(14.1699839717174,23.7543320991532,27.0968881392852));
#38092=CARTESIAN_POINT('Ctrl Pts',(14.1699839717174,23.7543320991532,27.0968881392852));
#38093=CARTESIAN_POINT('Ctrl Pts',(14.1251694706471,23.6006388275175,27.2664419709379));
#38094=CARTESIAN_POINT('Ctrl Pts',(14.0819995384234,23.4543320991532,27.4297736436309));
#38095=CARTESIAN_POINT('',(14.4846081098774,23.7543320991532,27.0250772328645));
#38096=CARTESIAN_POINT('Origin',(16.1460502915689,23.7543320991532,35.0294657090004));
#38097=CARTESIAN_POINT('',(14.7083129524589,23.4543320991532,27.2868216939543));
#38098=CARTESIAN_POINT('Ctrl Pts',(14.7083129524589,23.4543320991532,27.2868216939543));
#38099=CARTESIAN_POINT('Ctrl Pts',(14.5985512306315,23.6006388275175,27.1583956733261));
#38100=CARTESIAN_POINT('Ctrl Pts',(14.4846081098774,23.7543320991532,27.0250772328645));
#38101=CARTESIAN_POINT('',(14.8231378837717,23.7543320991532,26.9622153867842));
#38102=CARTESIAN_POINT('Ctrl Pts',(14.8231378837717,23.7543320991532,26.9622153867842));
#38103=CARTESIAN_POINT('Ctrl Pts',(14.7646522879161,23.6006388275175,27.1275522441746));
#38104=CARTESIAN_POINT('Ctrl Pts',(14.7083129524589,23.4543320991532,27.2868216939543));
#38105=CARTESIAN_POINT('',(15.1425683915998,23.7543320991532,26.9162882133188));
#38106=CARTESIAN_POINT('Origin',(16.1460502915689,23.7543320991532,35.0294657090004));
#38107=CARTESIAN_POINT('',(15.3441942712762,23.4543320991532,27.1953957627515));
#38108=CARTESIAN_POINT('Ctrl Pts',(15.3441942712762,23.4543320991532,27.1953957627515));
#38109=CARTESIAN_POINT('Ctrl Pts',(15.2452656854537,23.6006388275175,27.0584504698055));
#38110=CARTESIAN_POINT('Ctrl Pts',(15.1425683915998,23.7543320991532,26.9162882133188));
#38111=CARTESIAN_POINT('',(15.4850955596347,23.7543320991532,26.881228854175));
#38112=CARTESIAN_POINT('Ctrl Pts',(15.4850955596347,23.7543320991532,26.881228854175));
#38113=CARTESIAN_POINT('Ctrl Pts',(15.4133280809848,23.6006388275175,27.0412484477957));
#38114=CARTESIAN_POINT('Ctrl Pts',(15.3441942712762,23.4543320991532,27.1953957627515));
#38115=CARTESIAN_POINT('',(15.8072066798037,23.7543320991532,26.8614910514267));
#38116=CARTESIAN_POINT('Origin',(16.1460502915689,23.7543320991532,35.0294657090004));
#38117=CARTESIAN_POINT('Ctrl Pts',(15.9854118096115,23.4543320991532,27.1561042745104));
#38118=CARTESIAN_POINT('Ctrl Pts',(15.8979747132105,23.6006388275175,27.0115510575768));
#38119=CARTESIAN_POINT('Ctrl Pts',(15.8072066798037,23.7543320991532,26.8614910514267));
#38120=CARTESIAN_POINT('Origin',(16.1460502915689,-2.04566790084674,35.0294657090004));
#38121=CARTESIAN_POINT('',(16.1460502915689,32.8543320991532,33.0294657090004));
#38122=CARTESIAN_POINT('Origin',(16.1460502915689,32.8543320991532,35.0294657090004));
#38123=CARTESIAN_POINT('',(16.1460502915689,-2.04566790084674,33.0294657090004));
#38124=CARTESIAN_POINT('Origin',(16.1460502915689,-2.04566790084674,35.0294657090004));
#38125=CARTESIAN_POINT('',(8.05349305851946,42.8553320991532,36.1875427486737));
#38126=CARTESIAN_POINT('',(8.01409135636202,42.8553320991532,35.8672418581646));
#38127=CARTESIAN_POINT('Origin',(16.1460502915689,-2.04566790084674,35.0294657090004));
#38128=CARTESIAN_POINT('',(8.10943631257073,42.8553320991532,36.5272843737828));
#38129=CARTESIAN_POINT('',(8.17481440491953,42.8553320991532,36.8433078849883));
#38130=CARTESIAN_POINT('Origin',(16.1460502915689,-2.04566790084674,35.0294657090004));
#38131=CARTESIAN_POINT('',(8.25826360886169,42.8553320991532,37.1773591533095));
#38132=CARTESIAN_POINT('',(8.34918301098391,42.8553320991532,37.4870022008846));
#38133=CARTESIAN_POINT('Origin',(16.1460502915689,-2.04566790084674,35.0294657090004));
#38134=CARTESIAN_POINT('',(8.45958282413287,42.8553320991532,37.8131400563419));
#38135=CARTESIAN_POINT('',(8.57543848240802,42.8553320991532,38.1143420168924));
#38136=CARTESIAN_POINT('Origin',(16.1460502915689,-2.04566790084674,35.0294657090004));
#38137=CARTESIAN_POINT('',(8.71205421222198,42.8553320991532,38.4303960658666));
#38138=CARTESIAN_POINT('',(8.85207512635908,42.8553320991532,38.7211524900399));
#38139=CARTESIAN_POINT('Origin',(16.1460502915689,-2.04566790084674,35.0294657090004));
#38140=CARTESIAN_POINT('',(9.01399761769612,42.8553320991532,39.0250194449803));
#38141=CARTESIAN_POINT('',(9.17725197161342,42.8553320991532,39.303395396745));
#38142=CARTESIAN_POINT('Origin',(16.1460502915689,-2.04566790084674,35.0294657090004));
#38143=CARTESIAN_POINT('',(9.36340365700902,42.8553320991532,39.5930530732011));
#38144=CARTESIAN_POINT('',(9.54880501991626,42.8553320991532,39.857196006527));
#38145=CARTESIAN_POINT('Origin',(16.1460502915689,-2.04566790084674,35.0294657090004));
#38146=CARTESIAN_POINT('',(9.75794709061699,42.8553320991532,40.1307167804521));
#38147=CARTESIAN_POINT('',(9.96426164703311,42.8553320991532,40.3788688676983));
#38148=CARTESIAN_POINT('Origin',(16.1460502915689,-2.04566790084674,35.0294657090004));
#38149=CARTESIAN_POINT('',(10.1950022970645,42.8553320991532,40.6344325034697));
#38150=CARTESIAN_POINT('',(10.420857057656,42.8553320991532,40.864942333438));
#38151=CARTESIAN_POINT('Origin',(16.1460502915689,-2.04566790084674,35.0294657090004));
#38152=CARTESIAN_POINT('',(10.6716607460615,42.8553320991532,41.1008480972246));
#38153=CARTESIAN_POINT('',(10.9155526846602,42.8553320991532,41.3121816650278));
#38154=CARTESIAN_POINT('Origin',(16.1460502915689,-2.04566790084674,35.0294657090004));
#38155=CARTESIAN_POINT('',(11.1847503542733,42.8553320991532,41.5268596428934));
#38156=CARTESIAN_POINT('',(11.445056410267,42.8553320991532,41.7176105585055));
#38157=CARTESIAN_POINT('Origin',(16.1460502915689,-2.04566790084674,35.0294657090004));
#38158=CARTESIAN_POINT('',(11.7308565950109,42.8553320991532,41.9096321039267));
#38159=CARTESIAN_POINT('',(12.0058444745445,42.8553320991532,42.0785309514759));
#38160=CARTESIAN_POINT('Origin',(16.1460502915689,-2.04566790084674,35.0294657090004));
#38161=CARTESIAN_POINT('',(12.3063452213433,42.8553320991532,42.2466181927493));
#38162=CARTESIAN_POINT('',(12.5941849254484,42.8553320991532,42.3925409782716));
#38163=CARTESIAN_POINT('Origin',(16.1460502915689,-2.04566790084674,35.0294657090004));
#38164=CARTESIAN_POINT('',(12.9073864514114,42.8553320991532,42.5355753225389));
#38165=CARTESIAN_POINT('',(13.2061624543473,42.8553320991532,42.6575509539721));
#38166=CARTESIAN_POINT('Origin',(16.1460502915689,-2.04566790084674,35.0294657090004));
#38167=CARTESIAN_POINT('',(13.5299804549939,42.8553320991532,42.7745805312714));
#38168=CARTESIAN_POINT('',(13.8377044517555,42.8553320991532,42.8717972809129));
#38169=CARTESIAN_POINT('Origin',(16.1460502915689,-2.04566790084674,35.0294657090004));
#38170=CARTESIAN_POINT('',(14.1699839717175,42.8553320991532,42.9620432787156));
#38171=CARTESIAN_POINT('',(14.4846081098775,42.8553320991532,43.0338541851362));
#38172=CARTESIAN_POINT('Origin',(16.1460502915689,-2.04566790084674,35.0294657090004));
#38173=CARTESIAN_POINT('',(14.8231378837718,42.8553320991532,43.0967160312165));
#38174=CARTESIAN_POINT('',(15.1425683915999,42.8553320991532,43.142643204682));
#38175=CARTESIAN_POINT('Origin',(16.1460502915689,-2.04566790084674,35.0294657090004));
#38176=CARTESIAN_POINT('',(15.4850955596348,42.8553320991532,43.1777025638257));
#38177=CARTESIAN_POINT('',(15.8072066798038,42.8553320991532,43.197440366574));
#38178=CARTESIAN_POINT('Origin',(16.1460502915689,-2.04566790084674,35.0294657090004));
#38179=CARTESIAN_POINT('',(16.151451780189,42.8553320991532,43.2044639245305));
#38180=CARTESIAN_POINT('',(16.4740999163387,42.8553320991532,43.1978810047409));
#38181=CARTESIAN_POINT('Origin',(16.1460502915689,-2.04566790084674,35.0294657090004));
#38182=CARTESIAN_POINT('',(16.8177720547276,42.8553320991532,43.1768220208907));
#38183=CARTESIAN_POINT('',(17.1388100367452,42.8553320991532,43.1439621868083));
#38184=CARTESIAN_POINT('Origin',(16.1460502915689,-2.04566790084674,35.0294657090004));
#38185=CARTESIAN_POINT('',(17.4796221317587,42.8553320991532,43.0949608052144));
#38186=CARTESIAN_POINT('',(17.7969135048413,42.8553320991532,43.0360427336136));
#38187=CARTESIAN_POINT('Origin',(16.1460502915689,-2.04566790084674,35.0294657090004));
#38188=CARTESIAN_POINT('',(18.1325975082171,42.8553320991532,42.9594250503859));
#38189=CARTESIAN_POINT('',(18.4440307506264,42.8553320991532,42.8748408313122));
#38190=CARTESIAN_POINT('Origin',(16.1460502915689,-2.04566790084674,35.0294657090004));
#38191=CARTESIAN_POINT('',(18.772352740706,42.8553320991532,42.7711167244916));
#38192=CARTESIAN_POINT('',(19.0758553155965,42.8553320991532,42.6614292519677));
#38193=CARTESIAN_POINT('Origin',(16.1460502915689,-2.04566790084674,35.0294657090004));
#38194=CARTESIAN_POINT('',(19.3946303637053,42.8553320991532,42.5312889883718));
#38195=CARTESIAN_POINT('',(19.6881825115155,42.8553320991532,42.3972282144301));
#38196=CARTESIAN_POINT('Origin',(16.1460502915689,-2.04566790084674,35.0294657090004));
#38197=CARTESIAN_POINT('',(19.9952892223025,42.8553320991532,42.2415378560414));
#38198=CARTESIAN_POINT('',(20.2769374019215,42.8553320991532,42.0839959330141));
#38199=CARTESIAN_POINT('Origin',(16.1460502915689,-2.04566790084674,35.0294657090004));
#38200=CARTESIAN_POINT('',(20.5703320308954,42.8553320991532,41.9037915734806));
#38201=CARTESIAN_POINT('',(20.8382019201565,42.8553320991532,41.7238169168728));
#38202=CARTESIAN_POINT('Origin',(16.1460502915689,-2.04566790084674,35.0294657090004));
#38203=CARTESIAN_POINT('',(21.1159319744682,42.8553320991532,41.5202977864757));
#38204=CARTESIAN_POINT('',(21.3682409434537,42.8553320991532,41.3190880979334));
#38205=CARTESIAN_POINT('Origin',(16.1460502915689,-2.04566790084674,35.0294657090004));
#38206=CARTESIAN_POINT('',(21.628458175414,42.8553320991532,41.0936085829071));
#38207=CARTESIAN_POINT('',(21.8635271495635,42.8553320991532,40.8725028797102));
#38208=CARTESIAN_POINT('Origin',(16.1460502915689,-2.04566790084674,35.0294657090004));
#38209=CARTESIAN_POINT('',(22.1044998564265,42.8553320991532,40.6265635090257));
#38210=CARTESIAN_POINT('',(22.3207644905006,42.8553320991532,40.3870332131493));
#38211=CARTESIAN_POINT('Origin',(16.1460502915689,-2.04566790084674,35.0294657090004));
#38212=CARTESIAN_POINT('',(22.5408890386598,42.8553320991532,40.1222706727414));
#38213=CARTESIAN_POINT('',(22.7369101271999,42.8553320991532,39.8659098187846));
#38214=CARTESIAN_POINT('Origin',(16.1460502915689,-2.04566790084674,35.0294657090004));
#38215=CARTESIAN_POINT('',(22.9347216241054,42.8553320991532,39.584086059677));
#38216=CARTESIAN_POINT('',(23.1091946791084,42.8553320991532,39.3126006868265));
#38217=CARTESIAN_POINT('Origin',(16.1460502915689,-2.04566790084674,35.0294657090004));
#38218=CARTESIAN_POINT('',(23.2833767218849,42.8553320991532,39.0155911996383));
#38219=CARTESIAN_POINT('',(23.4351406539558,42.8553320991532,38.7307879982584));
#38220=CARTESIAN_POINT('Origin',(16.1460502915689,-2.04566790084674,35.0294657090004));
#38221=CARTESIAN_POINT('',(23.5845340898466,42.8553320991532,38.4205693321238));
#38222=CARTESIAN_POINT('',(23.7125789350568,42.8553320991532,38.1243436205306));
#38223=CARTESIAN_POINT('Origin',(16.1460502915689,-2.04566790084674,35.0294657090004));
#38224=CARTESIAN_POINT('',(23.8361895753942,42.8553320991532,37.8029802294902));
#38225=CARTESIAN_POINT('',(23.9396632164247,42.8553320991532,37.4973033409204));
#38226=CARTESIAN_POINT('Origin',(16.1460502915689,-2.04566790084674,35.0294657090004));
#38227=CARTESIAN_POINT('',(24.0366684527916,42.8553320991532,37.1669338453204));
#38228=CARTESIAN_POINT('',(24.1148822896334,42.8553320991532,36.8538400090343));
#38229=CARTESIAN_POINT('Origin',(16.1460502915689,-2.04566790084674,35.0294657090004));
#38230=CARTESIAN_POINT('',(24.1846365681864,42.8553320991532,36.5166629633608));
#38231=CARTESIAN_POINT('',(24.2370701006596,42.8553320991532,36.1982357671821));
#38232=CARTESIAN_POINT('Origin',(16.1460502915689,-2.04566790084674,35.0294657090004));
#38233=CARTESIAN_POINT('',(24.2791092181837,42.8553320991532,35.8564950290437));
#38234=CARTESIAN_POINT('',(24.3054135097807,42.8553320991532,35.5348535534261));
#38235=CARTESIAN_POINT('Origin',(16.1460502915689,-2.04566790084674,35.0294657090004));
#38236=CARTESIAN_POINT('',(24.3194577028847,42.8553320991532,35.1908233510519));
#38237=CARTESIAN_POINT('',(24.3194577028847,42.8553320991532,34.8681080669487));
#38238=CARTESIAN_POINT('Origin',(16.1460502915689,-2.04566790084674,35.0294657090004));
#38239=CARTESIAN_POINT('',(24.3054135097807,42.8553320991532,34.5240778645745));
#38240=CARTESIAN_POINT('',(24.2791092181837,42.8553320991532,34.2024363889569));
#38241=CARTESIAN_POINT('Origin',(16.1460502915689,-2.04566790084674,35.0294657090004));
#38242=CARTESIAN_POINT('',(24.2370701006596,42.8553320991532,33.8606956508185));
#38243=CARTESIAN_POINT('',(24.1846365681864,42.8553320991532,33.5422684546398));
#38244=CARTESIAN_POINT('Origin',(16.1460502915689,-2.04566790084674,35.0294657090004));
#38245=CARTESIAN_POINT('',(24.1148822896334,42.8553320991532,33.2050914089663));
#38246=CARTESIAN_POINT('',(24.0366684527916,42.8553320991532,32.8919975726802));
#38247=CARTESIAN_POINT('Origin',(16.1460502915689,-2.04566790084674,35.0294657090004));
#38248=CARTESIAN_POINT('',(23.9396632164247,42.8553320991532,32.5616280770803));
#38249=CARTESIAN_POINT('',(23.8361895753941,42.8553320991532,32.2559511885104));
#38250=CARTESIAN_POINT('Origin',(16.1460502915689,-2.04566790084674,35.0294657090004));
#38251=CARTESIAN_POINT('',(23.7125789350568,42.8553320991532,31.9345877974701));
#38252=CARTESIAN_POINT('',(23.5845340898465,42.8553320991532,31.6383620858768));
#38253=CARTESIAN_POINT('Origin',(16.1460502915689,-2.04566790084674,35.0294657090004));
#38254=CARTESIAN_POINT('',(23.4351406539558,42.8553320991532,31.3281434197422));
#38255=CARTESIAN_POINT('',(23.2833767218848,42.8553320991532,31.0433402183623));
#38256=CARTESIAN_POINT('Origin',(16.1460502915689,-2.04566790084674,35.0294657090004));
#38257=CARTESIAN_POINT('',(23.1091946791084,42.8553320991532,30.7463307311742));
#38258=CARTESIAN_POINT('',(22.9347216241054,42.8553320991532,30.4748453583237));
#38259=CARTESIAN_POINT('Origin',(16.1460502915689,-2.04566790084674,35.0294657090004));
#38260=CARTESIAN_POINT('',(22.7369101271998,42.8553320991532,30.193021599216));
#38261=CARTESIAN_POINT('',(22.5408890386598,42.8553320991532,29.9366607452593));
#38262=CARTESIAN_POINT('Origin',(16.1460502915689,-2.04566790084674,35.0294657090004));
#38263=CARTESIAN_POINT('',(22.3207644905005,42.8553320991532,29.6718982048514));
#38264=CARTESIAN_POINT('',(22.1044998564264,42.8553320991532,29.4323679089749));
#38265=CARTESIAN_POINT('Origin',(16.1460502915689,-2.04566790084674,35.0294657090004));
#38266=CARTESIAN_POINT('',(21.8635271495634,42.8553320991532,29.1864285382904));
#38267=CARTESIAN_POINT('',(21.6284581754139,42.8553320991532,28.9653228350936));
#38268=CARTESIAN_POINT('Origin',(16.1460502915689,-2.04566790084674,35.0294657090004));
#38269=CARTESIAN_POINT('',(21.3682409434536,42.8553320991532,28.7398433200673));
#38270=CARTESIAN_POINT('',(21.1159319744681,42.8553320991532,28.538633631525));
#38271=CARTESIAN_POINT('Origin',(16.1460502915689,-2.04566790084674,35.0294657090004));
#38272=CARTESIAN_POINT('',(20.8382019201564,42.8553320991532,28.3351145011278));
#38273=CARTESIAN_POINT('',(20.5703320308953,42.8553320991532,28.15513984452));
#38274=CARTESIAN_POINT('Origin',(16.1460502915689,-2.04566790084674,35.0294657090004));
#38275=CARTESIAN_POINT('',(20.2769374019214,42.8553320991532,27.9749354849866));
#38276=CARTESIAN_POINT('',(19.9952892223024,42.8553320991532,27.8173935619593));
#38277=CARTESIAN_POINT('Origin',(16.1460502915689,-2.04566790084674,35.0294657090004));
#38278=CARTESIAN_POINT('',(19.6881825115154,42.8553320991532,27.6617032035706));
#38279=CARTESIAN_POINT('',(19.3946303637052,42.8553320991532,27.5276424296289));
#38280=CARTESIAN_POINT('Origin',(16.1460502915689,-2.04566790084674,35.0294657090004));
#38281=CARTESIAN_POINT('',(19.0758553155964,42.8553320991532,27.397502166033));
#38282=CARTESIAN_POINT('',(18.7723527407059,42.8553320991532,27.2878146935091));
#38283=CARTESIAN_POINT('Origin',(16.1460502915689,-2.04566790084674,35.0294657090004));
#38284=CARTESIAN_POINT('',(18.4440307506263,42.8553320991532,27.1840905866885));
#38285=CARTESIAN_POINT('',(18.132597508217,42.8553320991532,27.0995063676148));
#38286=CARTESIAN_POINT('Origin',(16.1460502915689,-2.04566790084674,35.0294657090004));
#38287=CARTESIAN_POINT('',(17.7969135048412,42.8553320991532,27.0228886843871));
#38288=CARTESIAN_POINT('',(17.4796221317586,42.8553320991532,26.9639706127863));
#38289=CARTESIAN_POINT('Origin',(16.1460502915689,-2.04566790084674,35.0294657090004));
#38290=CARTESIAN_POINT('',(17.1388100367451,42.8553320991532,26.9149692311924));
#38291=CARTESIAN_POINT('',(16.8177720547275,42.8553320991532,26.88210939711));
#38292=CARTESIAN_POINT('Origin',(16.1460502915689,-2.04566790084674,35.0294657090004));
#38293=CARTESIAN_POINT('',(16.4740999163386,42.8553320991532,26.8610504132598));
#38294=CARTESIAN_POINT('',(16.1514517801889,42.8553320991532,26.8544674934702));
#38295=CARTESIAN_POINT('Origin',(16.1460502915689,-2.04566790084674,35.0294657090004));
#38296=CARTESIAN_POINT('',(15.8072066798037,42.8553320991532,26.8614910514267));
#38297=CARTESIAN_POINT('',(15.4850955596347,42.8553320991532,26.881228854175));
#38298=CARTESIAN_POINT('Origin',(16.1460502915689,-2.04566790084674,35.0294657090004));
#38299=CARTESIAN_POINT('',(15.1425683915998,42.8553320991532,26.9162882133188));
#38300=CARTESIAN_POINT('',(14.8231378837717,42.8553320991532,26.9622153867842));
#38301=CARTESIAN_POINT('Origin',(16.1460502915689,-2.04566790084674,35.0294657090004));
#38302=CARTESIAN_POINT('',(14.4846081098774,42.8553320991532,27.0250772328645));
#38303=CARTESIAN_POINT('',(14.1699839717174,42.8553320991532,27.0968881392852));
#38304=CARTESIAN_POINT('Origin',(16.1460502915689,-2.04566790084674,35.0294657090004));
#38305=CARTESIAN_POINT('',(13.8377044517554,42.8553320991532,27.1871341370879));
#38306=CARTESIAN_POINT('',(13.5299804549937,42.8553320991532,27.2843508867294));
#38307=CARTESIAN_POINT('Origin',(16.1460502915689,-2.04566790084674,35.0294657090004));
#38308=CARTESIAN_POINT('',(13.2061624543472,42.8553320991532,27.4013804640286));
#38309=CARTESIAN_POINT('',(12.9073864514113,42.8553320991532,27.5233560954618));
#38310=CARTESIAN_POINT('Origin',(16.1460502915689,-2.04566790084674,35.0294657090004));
#38311=CARTESIAN_POINT('',(12.5941849254483,42.8553320991532,27.6663904397292));
#38312=CARTESIAN_POINT('',(12.3063452213433,42.8553320991532,27.8123132252514));
#38313=CARTESIAN_POINT('Origin',(16.1460502915689,-2.04566790084674,35.0294657090004));
#38314=CARTESIAN_POINT('',(12.0058444745444,42.8553320991532,27.9804004665249));
#38315=CARTESIAN_POINT('',(11.7308565950108,42.8553320991532,28.1492993140741));
#38316=CARTESIAN_POINT('Origin',(16.1460502915689,-2.04566790084674,35.0294657090004));
#38317=CARTESIAN_POINT('',(11.4450564102669,42.8553320991532,28.3413208594953));
#38318=CARTESIAN_POINT('',(11.1847503542732,42.8553320991532,28.5320717751074));
#38319=CARTESIAN_POINT('Origin',(16.1460502915689,-2.04566790084674,35.0294657090004));
#38320=CARTESIAN_POINT('',(10.9155526846601,42.8553320991532,28.746749752973));
#38321=CARTESIAN_POINT('',(10.6716607460615,42.8553320991532,28.9580833207762));
#38322=CARTESIAN_POINT('Origin',(16.1460502915689,-2.04566790084674,35.0294657090004));
#38323=CARTESIAN_POINT('',(10.4208570576559,42.8553320991532,29.1939890845628));
#38324=CARTESIAN_POINT('',(10.1950022970644,42.8553320991532,29.4244989145311));
#38325=CARTESIAN_POINT('Origin',(16.1460502915689,-2.04566790084674,35.0294657090004));
#38326=CARTESIAN_POINT('',(9.96426164703304,42.8553320991532,29.6800625503025));
#38327=CARTESIAN_POINT('',(9.75794709061692,42.8553320991532,29.9282146375487));
#38328=CARTESIAN_POINT('Origin',(16.1460502915689,-2.04566790084674,35.0294657090004));
#38329=CARTESIAN_POINT('',(9.5488050199162,42.8553320991532,30.2017354114738));
#38330=CARTESIAN_POINT('',(9.36340365700895,42.8553320991532,30.4658783447997));
#38331=CARTESIAN_POINT('Origin',(16.1460502915689,-2.04566790084674,35.0294657090004));
#38332=CARTESIAN_POINT('',(9.17725197161336,42.8553320991532,30.7555360212558));
#38333=CARTESIAN_POINT('',(9.01399761769606,42.8553320991532,31.0339119730205));
#38334=CARTESIAN_POINT('Origin',(16.1460502915689,-2.04566790084674,35.0294657090004));
#38335=CARTESIAN_POINT('',(8.85207512635903,42.8553320991532,31.337778927961));
#38336=CARTESIAN_POINT('',(8.71205421222193,42.8553320991532,31.6285353521343));
#38337=CARTESIAN_POINT('Origin',(16.1460502915689,-2.04566790084674,35.0294657090004));
#38338=CARTESIAN_POINT('',(8.57543848240798,42.8553320991532,31.9445894011085));
#38339=CARTESIAN_POINT('',(8.45958282413283,42.8553320991532,32.245791361659));
#38340=CARTESIAN_POINT('Origin',(16.1460502915689,-2.04566790084674,35.0294657090004));
#38341=CARTESIAN_POINT('',(8.34918301098387,42.8553320991532,32.5719292171162));
#38342=CARTESIAN_POINT('',(8.25826360886166,42.8553320991532,32.8815722646913));
#38343=CARTESIAN_POINT('Origin',(16.1460502915689,-2.04566790084674,35.0294657090004));
#38344=CARTESIAN_POINT('',(8.17481440491951,42.8553320991532,33.2156235330125));
#38345=CARTESIAN_POINT('',(8.1094363125707,42.8553320991532,33.5316470442181));
#38346=CARTESIAN_POINT('Origin',(16.1460502915689,-2.04566790084674,35.0294657090004));
#38347=CARTESIAN_POINT('',(8.05349305851944,42.8553320991532,33.8713886693271));
#38348=CARTESIAN_POINT('',(8.01409135636201,42.8553320991532,34.1916895598362));
#38349=CARTESIAN_POINT('Origin',(16.1460502915689,-2.04566790084674,35.0294657090004));
#38350=CARTESIAN_POINT('',(7.98602634532737,42.8553320991532,35.5240708007294));
#38351=CARTESIAN_POINT('',(7.97286324518834,42.8553320991532,35.2016240804971));
#38352=CARTESIAN_POINT('Origin',(16.1460502915689,23.3543320991532,35.0294657090004));
#38353=CARTESIAN_POINT('Origin',(16.1460502915689,-2.04566790084674,35.0294657090004));
#38354=CARTESIAN_POINT('',(7.98602634532736,42.8553320991532,34.5348606172715));
#38355=CARTESIAN_POINT('',(7.97286324518834,42.8553320991532,34.8573073375037));
#38356=CARTESIAN_POINT('Origin',(12.1460502915689,26.8543320991532,35.0294657090004));
#38357=CARTESIAN_POINT('Origin',(12.1460502915689,32.8543320991532,35.0294657090004));
#38358=CARTESIAN_POINT('Origin',(14.5360502915689,42.8543320991532,35.0294657090004));
#38359=CARTESIAN_POINT('Origin',(8.27105029156894,42.8553320991532,35.0294657090004));
#38360=CARTESIAN_POINT('',(8.27105029156894,42.8553320991532,35.0294657090004));
#38361=CARTESIAN_POINT('Origin',(8.27105029156894,42.8553320991532,35.0294657090004));
#38362=CARTESIAN_POINT('Origin',(8.29725370442717,42.8553320991532,35.6713513169335));
#38363=CARTESIAN_POINT('',(8.29725370442717,42.8553320991532,35.6713513169335));
#38364=CARTESIAN_POINT('Origin',(8.29725370442717,42.8553320991532,35.6713513169335));
#38365=CARTESIAN_POINT('Origin',(8.29725370442716,42.8553320991532,34.3875801010673));
#38366=CARTESIAN_POINT('',(8.29725370442716,42.8553320991532,34.3875801010673));
#38367=CARTESIAN_POINT('Origin',(8.29725370442716,42.8553320991532,34.3875801010673));
#38368=CARTESIAN_POINT('Origin',(8.37568956361252,42.8553320991532,33.7499661359513));
#38369=CARTESIAN_POINT('',(8.37568956361252,42.8553320991532,33.7499661359513));
#38370=CARTESIAN_POINT('Origin',(8.37568956361252,42.8553320991532,33.7499661359513));
#38371=CARTESIAN_POINT('Origin',(8.50583589142315,42.8553320991532,33.1208670293914));
#38372=CARTESIAN_POINT('',(8.50583589142315,42.8553320991532,33.1208670293914));
#38373=CARTESIAN_POINT('Origin',(8.50583589142315,42.8553320991532,33.1208670293914));
#38374=CARTESIAN_POINT('Origin',(8.68682658552011,42.8553320991532,32.5044693321477));
#38375=CARTESIAN_POINT('',(8.68682658552011,42.8553320991532,32.5044693321477));
#38376=CARTESIAN_POINT('Origin',(8.68682658552011,42.8553320991532,32.5044693321477));
#38377=CARTESIAN_POINT('Origin',(8.91745718269554,42.8553320991532,31.9048750691968));
#38378=CARTESIAN_POINT('',(8.91745718269554,42.8553320991532,31.9048750691968));
#38379=CARTESIAN_POINT('Origin',(8.91745718269554,42.8553320991532,31.9048750691968));
#38380=CARTESIAN_POINT('Origin',(9.19619287437661,42.8553320991532,31.3260744414326));
#38381=CARTESIAN_POINT('',(9.19619287437661,42.8553320991532,31.3260744414326));
#38382=CARTESIAN_POINT('Origin',(9.19619287437661,42.8553320991532,31.3260744414326));
#38383=CARTESIAN_POINT('Origin',(9.52117872052333,42.8553320991532,30.7719192715376));
#38384=CARTESIAN_POINT('',(9.52117872052333,42.8553320991532,30.7719192715376));
#38385=CARTESIAN_POINT('Origin',(9.52117872052333,42.8553320991532,30.7719192715376));
#38386=CARTESIAN_POINT('Origin',(9.89025199394849,42.8553320991532,30.2460973707382));
#38387=CARTESIAN_POINT('',(9.89025199394849,42.8553320991532,30.2460973707382));
#38388=CARTESIAN_POINT('Origin',(9.89025199394849,42.8553320991532,30.2460973707382));
#38389=CARTESIAN_POINT('Origin',(10.3009565729103,42.8553320991532,29.7521079970296));
#38390=CARTESIAN_POINT('',(10.3009565729103,42.8553320991532,29.7521079970296));
#38391=CARTESIAN_POINT('Origin',(10.3009565729103,42.8553320991532,29.7521079970296));
#38392=CARTESIAN_POINT('Origin',(10.7505592861971,42.8553320991532,29.2932385681916));
#38393=CARTESIAN_POINT('',(10.7505592861971,42.8553320991532,29.2932385681916));
#38394=CARTESIAN_POINT('Origin',(10.7505592861971,42.8553320991532,29.2932385681916));
#38395=CARTESIAN_POINT('Origin',(11.2360681019313,42.8553320991532,28.8725427845647));
#38396=CARTESIAN_POINT('',(11.2360681019313,42.8553320991532,28.8725427845647));
#38397=CARTESIAN_POINT('Origin',(11.2360681019313,42.8553320991532,28.8725427845647));
#38398=CARTESIAN_POINT('Origin',(11.7542520390476,42.8553320991532,28.4928203071792));
#38399=CARTESIAN_POINT('',(11.7542520390476,42.8553320991532,28.4928203071792));
#38400=CARTESIAN_POINT('Origin',(11.7542520390476,42.8553320991532,28.4928203071792));
#38401=CARTESIAN_POINT('Origin',(12.3016626689386,42.8553320991532,28.1565981264722));
#38402=CARTESIAN_POINT('',(12.3016626689386,42.8553320991532,28.1565981264722));
#38403=CARTESIAN_POINT('Origin',(12.3016626689386,42.8553320991532,28.1565981264722));
#38404=CARTESIAN_POINT('Origin',(12.874657064179,42.8553320991532,27.8661137455836));
#38405=CARTESIAN_POINT('',(12.874657064179,42.8553320991532,27.8661137455836));
#38406=CARTESIAN_POINT('Origin',(12.874657064179,42.8553320991532,27.8661137455836));
#38407=CARTESIAN_POINT('Origin',(13.4694220416057,42.8553320991532,27.6233002901416));
#38408=CARTESIAN_POINT('',(13.4694220416057,42.8553320991532,27.6233002901416));
#38409=CARTESIAN_POINT('Origin',(13.4694220416057,42.8553320991532,27.6233002901416));
#38410=CARTESIAN_POINT('Origin',(14.0819995384234,42.8553320991532,27.4297736436309));
#38411=CARTESIAN_POINT('',(14.0819995384234,42.8553320991532,27.4297736436309));
#38412=CARTESIAN_POINT('Origin',(14.0819995384234,42.8553320991532,27.4297736436309));
#38413=CARTESIAN_POINT('Origin',(14.7083129524589,42.8553320991532,27.2868216939543));
#38414=CARTESIAN_POINT('',(14.7083129524589,42.8553320991532,27.2868216939543));
#38415=CARTESIAN_POINT('Origin',(14.7083129524589,42.8553320991532,27.2868216939543));
#38416=CARTESIAN_POINT('Origin',(15.3441942712762,42.8553320991532,27.1953957627515));
#38417=CARTESIAN_POINT('',(15.3441942712762,42.8553320991532,27.1953957627515));
#38418=CARTESIAN_POINT('Origin',(15.3441942712762,42.8553320991532,27.1953957627515));
#38419=CARTESIAN_POINT('Origin',(15.9854118096115,42.8553320991532,27.1561042745104));
#38420=CARTESIAN_POINT('',(15.9854118096115,42.8553320991532,27.1561042745104));
#38421=CARTESIAN_POINT('Origin',(15.9854118096115,42.8553320991532,27.1561042745104));
#38422=CARTESIAN_POINT('Origin',(16.6276983705409,42.8553320991532,27.1692087076026));
#38423=CARTESIAN_POINT('',(16.6276983705409,42.8553320991532,27.1692087076026));
#38424=CARTESIAN_POINT('Origin',(16.6276983705409,42.8553320991532,27.1692087076026));
#38425=CARTESIAN_POINT('Origin',(17.266779642971,42.8553320991532,27.234621854188));
#38426=CARTESIAN_POINT('',(17.266779642971,42.8553320991532,27.234621854188));
#38427=CARTESIAN_POINT('Origin',(17.266779642971,42.8553320991532,27.234621854188));
#38428=CARTESIAN_POINT('Origin',(17.8984026464748,42.8553320991532,27.3519084005685));
#38429=CARTESIAN_POINT('',(17.8984026464748,42.8553320991532,27.3519084005685));
#38430=CARTESIAN_POINT('Origin',(17.8984026464748,42.8553320991532,27.3519084005685));
#38431=CARTESIAN_POINT('Origin',(18.5183640341746,42.8553320991532,27.5202878241288));
#38432=CARTESIAN_POINT('',(18.5183640341746,42.8553320991532,27.5202878241288));
#38433=CARTESIAN_POINT('Origin',(18.5183640341746,42.8553320991532,27.5202878241288));
#38434=CARTESIAN_POINT('Origin',(19.1225380653215,42.8553320991532,27.7386395875858));
#38435=CARTESIAN_POINT('',(19.1225380653215,42.8553320991532,27.7386395875858));
#38436=CARTESIAN_POINT('Origin',(19.1225380653215,42.8553320991532,27.7386395875858));
#38437=CARTESIAN_POINT('Origin',(19.70690406142,42.8553320991532,28.0055105959791));
#38438=CARTESIAN_POINT('',(19.70690406142,42.8553320991532,28.0055105959791));
#38439=CARTESIAN_POINT('Origin',(19.70690406142,42.8553320991532,28.0055105959791));
#38440=CARTESIAN_POINT('Origin',(20.2675731631797,42.8553320991532,28.3191248667786));
#38441=CARTESIAN_POINT('',(20.2675731631797,42.8553320991532,28.3191248667786));
#38442=CARTESIAN_POINT('Origin',(20.2675731631797,42.8553320991532,28.3191248667786));
#38443=CARTESIAN_POINT('Origin',(20.8008142102322,42.8553320991532,28.6773953487548));
#38444=CARTESIAN_POINT('',(20.8008142102322,42.8553320991532,28.6773953487548));
#38445=CARTESIAN_POINT('Origin',(20.8008142102322,42.8553320991532,28.6773953487548));
#38446=CARTESIAN_POINT('Origin',(21.303078571388,42.8553320991532,29.0779378109605));
#38447=CARTESIAN_POINT('',(21.303078571388,42.8553320991532,29.0779378109605));
#38448=CARTESIAN_POINT('Origin',(21.303078571388,42.8553320991532,29.0779378109605));
#38449=CARTESIAN_POINT('Origin',(21.7710237601914,42.8553320991532,29.5180867093948));
#38450=CARTESIAN_POINT('',(21.7710237601914,42.8553320991532,29.5180867093948));
#38451=CARTESIAN_POINT('Origin',(21.7710237601914,42.8553320991532,29.5180867093948));
#38452=CARTESIAN_POINT('Origin',(22.2015356786164,42.8553320991532,29.9949129257578));
#38453=CARTESIAN_POINT('',(22.2015356786164,42.8553320991532,29.9949129257578));
#38454=CARTESIAN_POINT('Origin',(22.2015356786164,42.8553320991532,29.9949129257578));
#38455=CARTESIAN_POINT('Origin',(22.5917493408753,42.8553320991532,30.5052432602507));
#38456=CARTESIAN_POINT('',(22.5917493408753,42.8553320991532,30.5052432602507));
#38457=CARTESIAN_POINT('Origin',(22.5917493408753,42.8553320991532,30.5052432602507));
#38458=CARTESIAN_POINT('Origin',(22.9390679394266,42.8553320991532,31.0456815486958));
#38459=CARTESIAN_POINT('',(22.9390679394266,42.8553320991532,31.0456815486958));
#38460=CARTESIAN_POINT('Origin',(22.9390679394266,42.8553320991532,31.0456815486958));
#38461=CARTESIAN_POINT('Origin',(23.2411801263005,42.8553320991532,31.6126312634495));
#38462=CARTESIAN_POINT('',(23.2411801263005,42.8553320991532,31.6126312634495));
#38463=CARTESIAN_POINT('Origin',(23.2411801263005,42.8553320991532,31.6126312634495));
#38464=CARTESIAN_POINT('Origin',(23.4960753947382,42.8553320991532,32.2023194477005));
#38465=CARTESIAN_POINT('',(23.4960753947382,42.8553320991532,32.2023194477005));
#38466=CARTESIAN_POINT('Origin',(23.4960753947382,42.8553320991532,32.2023194477005));
#38467=CARTESIAN_POINT('Origin',(23.7020574587831,42.8553320991532,32.8108218238741));
#38468=CARTESIAN_POINT('',(23.7020574587831,42.8553320991532,32.8108218238741));
#38469=CARTESIAN_POINT('Origin',(23.7020574587831,42.8553320991532,32.8108218238741));
#38470=CARTESIAN_POINT('Origin',(23.8577555417836,42.8553320991532,33.4340889090527));
#38471=CARTESIAN_POINT('',(23.8577555417836,42.8553320991532,33.4340889090527));
#38472=CARTESIAN_POINT('Origin',(23.8577555417836,42.8553320991532,33.4340889090527));
#38473=CARTESIAN_POINT('Origin',(23.9621334986858,42.8553320991532,34.0679729636163));
#38474=CARTESIAN_POINT('',(23.9621334986858,42.8553320991532,34.0679729636163));
#38475=CARTESIAN_POINT('Origin',(23.9621334986858,42.8553320991532,34.0679729636163));
#38476=CARTESIAN_POINT('Origin',(24.0144967114075,42.8553320991532,34.7082555937653));
#38477=CARTESIAN_POINT('',(24.0144967114075,42.8553320991532,34.7082555937653));
#38478=CARTESIAN_POINT('Origin',(24.0144967114075,42.8553320991532,34.7082555937653));
#38479=CARTESIAN_POINT('Origin',(24.0144967114075,42.8553320991532,35.3506758242353));
#38480=CARTESIAN_POINT('',(24.0144967114075,42.8553320991532,35.3506758242353));
#38481=CARTESIAN_POINT('Origin',(24.0144967114075,42.8553320991532,35.3506758242353));
#38482=CARTESIAN_POINT('Origin',(23.9621334986858,42.8553320991532,35.9909584543843));
#38483=CARTESIAN_POINT('',(23.9621334986858,42.8553320991532,35.9909584543843));
#38484=CARTESIAN_POINT('Origin',(23.9621334986858,42.8553320991532,35.9909584543843));
#38485=CARTESIAN_POINT('Origin',(23.8577555417836,42.8553320991532,36.6248425089479));
#38486=CARTESIAN_POINT('',(23.8577555417836,42.8553320991532,36.6248425089479));
#38487=CARTESIAN_POINT('Origin',(23.8577555417836,42.8553320991532,36.6248425089479));
#38488=CARTESIAN_POINT('Origin',(23.7020574587831,42.8553320991532,37.2481095941266));
#38489=CARTESIAN_POINT('',(23.7020574587831,42.8553320991532,37.2481095941266));
#38490=CARTESIAN_POINT('Origin',(23.7020574587831,42.8553320991532,37.2481095941266));
#38491=CARTESIAN_POINT('Origin',(23.4960753947382,42.8553320991532,37.8566119703002));
#38492=CARTESIAN_POINT('',(23.4960753947382,42.8553320991532,37.8566119703002));
#38493=CARTESIAN_POINT('Origin',(23.4960753947382,42.8553320991532,37.8566119703002));
#38494=CARTESIAN_POINT('Origin',(23.2411801263005,42.8553320991532,38.4463001545511));
#38495=CARTESIAN_POINT('',(23.2411801263005,42.8553320991532,38.4463001545511));
#38496=CARTESIAN_POINT('Origin',(23.2411801263005,42.8553320991532,38.4463001545511));
#38497=CARTESIAN_POINT('Origin',(22.9390679394267,42.8553320991532,39.0132498693049));
#38498=CARTESIAN_POINT('',(22.9390679394267,42.8553320991532,39.0132498693049));
#38499=CARTESIAN_POINT('Origin',(22.9390679394267,42.8553320991532,39.0132498693049));
#38500=CARTESIAN_POINT('Origin',(22.5917493408754,42.8553320991532,39.55368815775));
#38501=CARTESIAN_POINT('',(22.5917493408754,42.8553320991532,39.55368815775));
#38502=CARTESIAN_POINT('Origin',(22.5917493408754,42.8553320991532,39.55368815775));
#38503=CARTESIAN_POINT('Origin',(22.2015356786164,42.8553320991532,40.0640184922428));
#38504=CARTESIAN_POINT('',(22.2015356786164,42.8553320991532,40.0640184922428));
#38505=CARTESIAN_POINT('Origin',(22.2015356786164,42.8553320991532,40.0640184922428));
#38506=CARTESIAN_POINT('Origin',(21.7710237601915,42.8553320991532,40.5408447086059));
#38507=CARTESIAN_POINT('',(21.7710237601915,42.8553320991532,40.5408447086059));
#38508=CARTESIAN_POINT('Origin',(21.7710237601915,42.8553320991532,40.5408447086059));
#38509=CARTESIAN_POINT('Origin',(21.3030785713881,42.8553320991532,40.9809936070401));
#38510=CARTESIAN_POINT('',(21.3030785713881,42.8553320991532,40.9809936070401));
#38511=CARTESIAN_POINT('Origin',(21.3030785713881,42.8553320991532,40.9809936070401));
#38512=CARTESIAN_POINT('Origin',(20.8008142102323,42.8553320991532,41.3815360692459));
#38513=CARTESIAN_POINT('',(20.8008142102323,42.8553320991532,41.3815360692459));
#38514=CARTESIAN_POINT('Origin',(20.8008142102323,42.8553320991532,41.3815360692459));
#38515=CARTESIAN_POINT('Origin',(20.2675731631798,42.8553320991532,41.7398065512221));
#38516=CARTESIAN_POINT('',(20.2675731631798,42.8553320991532,41.7398065512221));
#38517=CARTESIAN_POINT('Origin',(20.2675731631798,42.8553320991532,41.7398065512221));
#38518=CARTESIAN_POINT('Origin',(19.7069040614201,42.8553320991532,42.0534208220216));
#38519=CARTESIAN_POINT('',(19.7069040614201,42.8553320991532,42.0534208220216));
#38520=CARTESIAN_POINT('Origin',(19.7069040614201,42.8553320991532,42.0534208220216));
#38521=CARTESIAN_POINT('Origin',(19.1225380653216,42.8553320991532,42.3202918304149));
#38522=CARTESIAN_POINT('',(19.1225380653216,42.8553320991532,42.3202918304149));
#38523=CARTESIAN_POINT('Origin',(19.1225380653216,42.8553320991532,42.3202918304149));
#38524=CARTESIAN_POINT('Origin',(18.5183640341747,42.8553320991532,42.5386435938719));
#38525=CARTESIAN_POINT('',(18.5183640341747,42.8553320991532,42.5386435938719));
#38526=CARTESIAN_POINT('Origin',(18.5183640341747,42.8553320991532,42.5386435938719));
#38527=CARTESIAN_POINT('Origin',(17.8984026464749,42.8553320991532,42.7070230174322));
#38528=CARTESIAN_POINT('',(17.8984026464749,42.8553320991532,42.7070230174322));
#38529=CARTESIAN_POINT('Origin',(17.8984026464749,42.8553320991532,42.7070230174322));
#38530=CARTESIAN_POINT('Origin',(17.2667796429711,42.8553320991532,42.8243095638127));
#38531=CARTESIAN_POINT('',(17.2667796429711,42.8553320991532,42.8243095638127));
#38532=CARTESIAN_POINT('Origin',(17.2667796429711,42.8553320991532,42.8243095638127));
#38533=CARTESIAN_POINT('Origin',(16.627698370541,42.8553320991532,42.8897227103981));
#38534=CARTESIAN_POINT('',(16.627698370541,42.8553320991532,42.8897227103981));
#38535=CARTESIAN_POINT('Origin',(16.627698370541,42.8553320991532,42.8897227103981));
#38536=CARTESIAN_POINT('Origin',(15.9854118096116,42.8553320991532,42.9028271434904));
#38537=CARTESIAN_POINT('',(15.9854118096116,42.8553320991532,42.9028271434904));
#38538=CARTESIAN_POINT('Origin',(15.9854118096116,42.8553320991532,42.9028271434904));
#38539=CARTESIAN_POINT('Origin',(15.3441942712763,42.8553320991532,42.8635356552493));
#38540=CARTESIAN_POINT('',(15.3441942712763,42.8553320991532,42.8635356552493));
#38541=CARTESIAN_POINT('Origin',(15.3441942712763,42.8553320991532,42.8635356552493));
#38542=CARTESIAN_POINT('Origin',(14.708312952459,42.8553320991532,42.7721097240465));
#38543=CARTESIAN_POINT('',(14.708312952459,42.8553320991532,42.7721097240465));
#38544=CARTESIAN_POINT('Origin',(14.708312952459,42.8553320991532,42.7721097240465));
#38545=CARTESIAN_POINT('Origin',(14.0819995384235,42.8553320991532,42.6291577743698));
#38546=CARTESIAN_POINT('',(14.0819995384235,42.8553320991532,42.6291577743698));
#38547=CARTESIAN_POINT('Origin',(14.0819995384235,42.8553320991532,42.6291577743698));
#38548=CARTESIAN_POINT('Origin',(13.4694220416058,42.8553320991532,42.4356311278591));
#38549=CARTESIAN_POINT('',(13.4694220416058,42.8553320991532,42.4356311278591));
#38550=CARTESIAN_POINT('Origin',(13.4694220416058,42.8553320991532,42.4356311278591));
#38551=CARTESIAN_POINT('Origin',(12.8746570641791,42.8553320991532,42.1928176724172));
#38552=CARTESIAN_POINT('',(12.8746570641791,42.8553320991532,42.1928176724172));
#38553=CARTESIAN_POINT('Origin',(12.8746570641791,42.8553320991532,42.1928176724172));
#38554=CARTESIAN_POINT('Origin',(12.3016626689387,42.8553320991532,41.9023332915286));
#38555=CARTESIAN_POINT('',(12.3016626689387,42.8553320991532,41.9023332915286));
#38556=CARTESIAN_POINT('Origin',(12.3016626689387,42.8553320991532,41.9023332915286));
#38557=CARTESIAN_POINT('Origin',(11.7542520390477,42.8553320991532,41.5661111108216));
#38558=CARTESIAN_POINT('',(11.7542520390477,42.8553320991532,41.5661111108216));
#38559=CARTESIAN_POINT('Origin',(11.7542520390477,42.8553320991532,41.5661111108216));
#38560=CARTESIAN_POINT('Origin',(11.2360681019314,42.8553320991532,41.1863886334361));
#38561=CARTESIAN_POINT('',(11.2360681019314,42.8553320991532,41.1863886334361));
#38562=CARTESIAN_POINT('Origin',(11.2360681019314,42.8553320991532,41.1863886334361));
#38563=CARTESIAN_POINT('Origin',(10.7505592861972,42.8553320991532,40.7656928498092));
#38564=CARTESIAN_POINT('',(10.7505592861972,42.8553320991532,40.7656928498092));
#38565=CARTESIAN_POINT('Origin',(10.7505592861972,42.8553320991532,40.7656928498092));
#38566=CARTESIAN_POINT('Origin',(10.3009565729103,42.8553320991532,40.3068234209711));
#38567=CARTESIAN_POINT('',(10.3009565729103,42.8553320991532,40.3068234209711));
#38568=CARTESIAN_POINT('Origin',(10.3009565729103,42.8553320991532,40.3068234209711));
#38569=CARTESIAN_POINT('Origin',(9.89025199394856,42.8553320991532,39.8128340472626));
#38570=CARTESIAN_POINT('',(9.89025199394856,42.8553320991532,39.8128340472626));
#38571=CARTESIAN_POINT('Origin',(9.89025199394856,42.8553320991532,39.8128340472626));
#38572=CARTESIAN_POINT('Origin',(9.52117872052339,42.8553320991532,39.2870121464632));
#38573=CARTESIAN_POINT('',(9.52117872052339,42.8553320991532,39.2870121464632));
#38574=CARTESIAN_POINT('Origin',(9.52117872052339,42.8553320991532,39.2870121464632));
#38575=CARTESIAN_POINT('Origin',(9.19619287437666,42.8553320991532,38.7328569765682));
#38576=CARTESIAN_POINT('',(9.19619287437666,42.8553320991532,38.7328569765682));
#38577=CARTESIAN_POINT('Origin',(9.19619287437666,42.8553320991532,38.7328569765682));
#38578=CARTESIAN_POINT('Origin',(8.91745718269558,42.8553320991532,38.154056348804));
#38579=CARTESIAN_POINT('',(8.91745718269558,42.8553320991532,38.154056348804));
#38580=CARTESIAN_POINT('Origin',(8.91745718269558,42.8553320991532,38.154056348804));
#38581=CARTESIAN_POINT('Origin',(8.68682658552015,42.8553320991532,37.5544620858532));
#38582=CARTESIAN_POINT('',(8.68682658552015,42.8553320991532,37.5544620858532));
#38583=CARTESIAN_POINT('Origin',(8.68682658552015,42.8553320991532,37.5544620858532));
#38584=CARTESIAN_POINT('Origin',(8.50583589142318,42.8553320991532,36.9380643886094));
#38585=CARTESIAN_POINT('',(8.50583589142318,42.8553320991532,36.9380643886094));
#38586=CARTESIAN_POINT('Origin',(8.50583589142318,42.8553320991532,36.9380643886094));
#38587=CARTESIAN_POINT('Origin',(8.37568956361254,42.8553320991532,36.3089652820495));
#38588=CARTESIAN_POINT('',(8.37568956361254,42.8553320991532,36.3089652820495));
#38589=CARTESIAN_POINT('Origin',(8.37568956361254,42.8553320991532,36.3089652820495));
#38618=UNCERTAINTY_MEASURE_WITH_UNIT(LENGTH_MEASURE(0.01),#38636,
'DISTANCE_ACCURACY_VALUE',
'Maximum model space distance between geometric entities at asserted c
onnectivities');
#38619=UNCERTAINTY_MEASURE_WITH_UNIT(LENGTH_MEASURE(0.01),#38636,
'DISTANCE_ACCURACY_VALUE',
'Maximum model space distance between geometric entities at asserted c
onnectivities');
#38634=(
GEOMETRIC_REPRESENTATION_CONTEXT(3)
GLOBAL_UNCERTAINTY_ASSIGNED_CONTEXT((#38618))
GLOBAL_UNIT_ASSIGNED_CONTEXT((#38636,#38638,#38639))
REPRESENTATION_CONTEXT('','3D')
);
#38635=(
GEOMETRIC_REPRESENTATION_CONTEXT(3)
GLOBAL_UNCERTAINTY_ASSIGNED_CONTEXT((#38619))
GLOBAL_UNIT_ASSIGNED_CONTEXT((#38636,#38638,#38639))
REPRESENTATION_CONTEXT('','3D')
);
#38636=(
LENGTH_UNIT()
NAMED_UNIT(*)
SI_UNIT(.MILLI.,.METRE.)
);
#38638=(
NAMED_UNIT(*)
PLANE_ANGLE_UNIT()
SI_UNIT($,.RADIAN.)
);
#38639=(
NAMED_UNIT(*)
SI_UNIT($,.STERADIAN.)
SOLID_ANGLE_UNIT()
);
#38654=SHAPE_DEFINITION_REPRESENTATION(#38669,#38698);
#38669=PRODUCT_DEFINITION_SHAPE('',$,#38714);
#38698=SHAPE_REPRESENTATION('',(#18447),#38634);
#38699=PRODUCT_DEFINITION_CONTEXT('part definition',#38746,'design');
#38714=PRODUCT_DEFINITION('Microfeed Holder','Microfeed Holder',#38729,
#38699);
#38729=PRODUCT_DEFINITION_FORMATION('',$,#38762);
#38746=APPLICATION_CONTEXT(
'Core Data for Automotive Mechanical Design Process');
#38747=PRODUCT_CONTEXT('part definition',#38746,'mechanical');
#38762=PRODUCT('Microfeed Holder','Microfeed Holder',$,(#38747));
#38765=PRESENTATION_STYLE_ASSIGNMENT((#38772));
#38772=SURFACE_STYLE_USAGE(.BOTH.,#38779);
#38779=SURFACE_SIDE_STYLE('',(#38786));
#38786=SURFACE_STYLE_FILL_AREA(#38793);
#38793=FILL_AREA_STYLE('Opaque(227,224,212)',(#38800));
#38800=FILL_AREA_STYLE_COLOUR('Opaque(227,224,212)',#38807);
#38807=COLOUR_RGB('Opaque(227,224,212)',0.890196078431372,0.87843137254902,
0.831372549019608);
ENDSEC;
END-ISO-10303-21;
